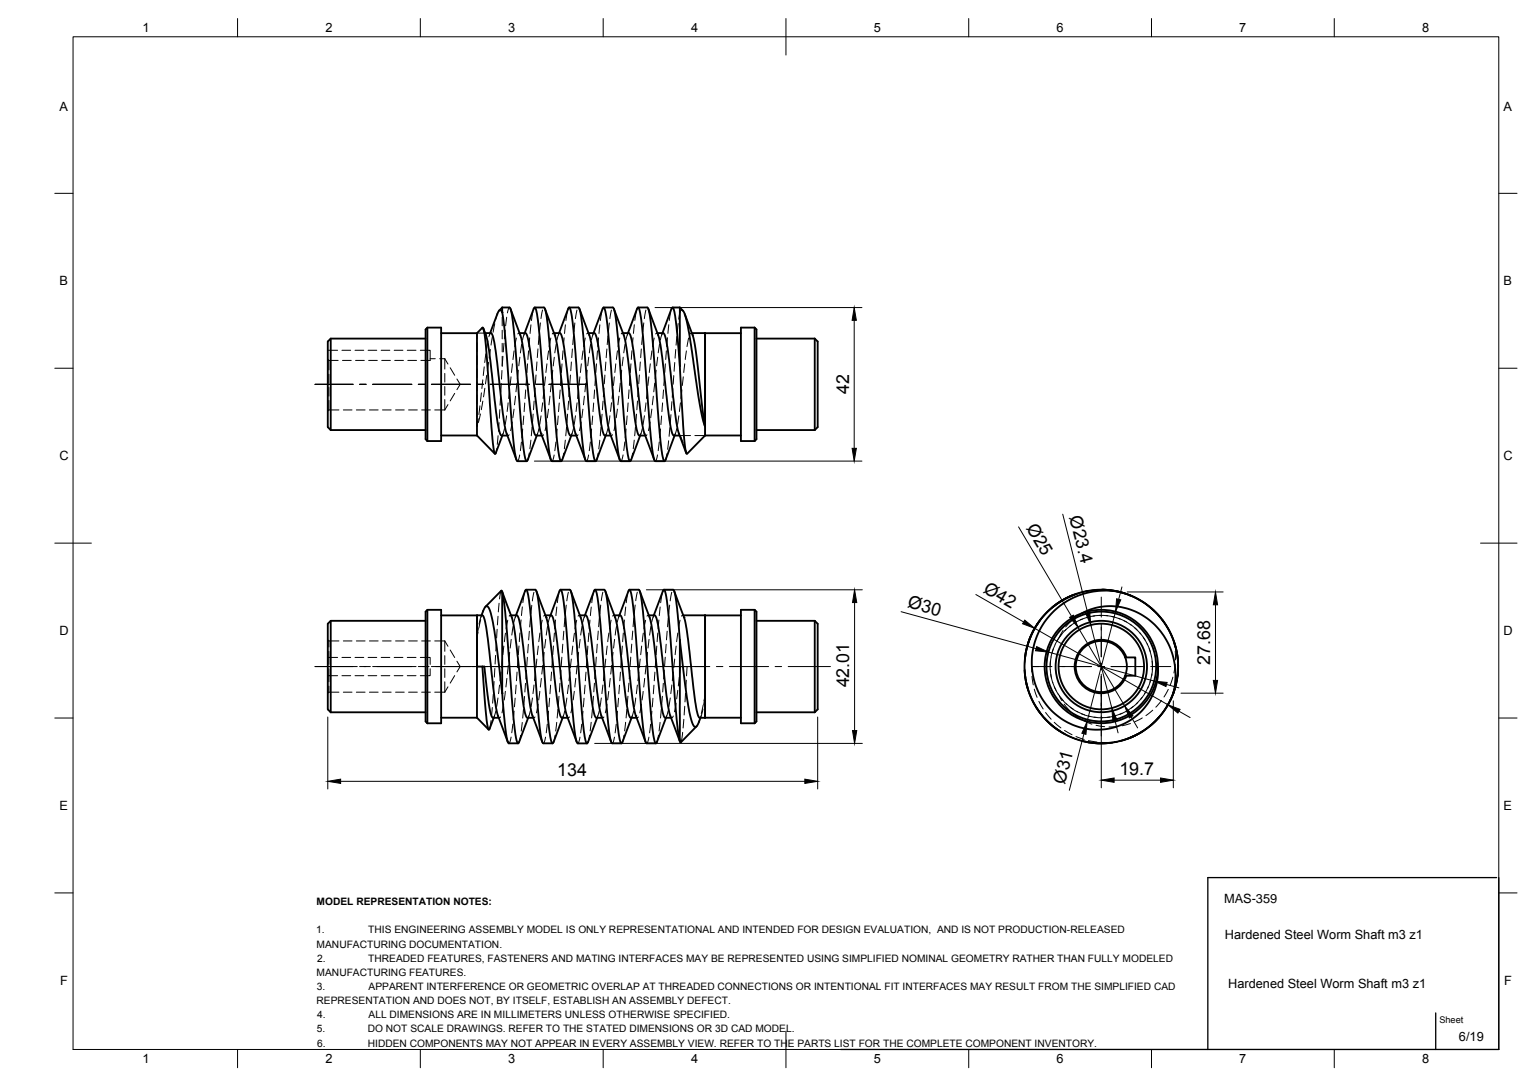
ISO-10303-21;
HEADER;
/* Generated by software containing ST-Developer
 * from STEP Tools, Inc. (www.steptools.com) 
 */

FILE_DESCRIPTION(
/* description */ (''),
/* implementation_level */ '2;1');

FILE_NAME(
/* name */ 'Hardened Steel Worm Shaft m3 z1.step',
/* time_stamp */ '2026-10-15T14:25:16-07:00',
/* author */ (''),
/* organization */ (''),
/* preprocessor_version */ 'ST-DEVELOPER v20.2',
/* originating_system */ 'Autodesk Translation Framework v15.15.0.0',
/* authorisation */ '');

FILE_SCHEMA (('AUTOMOTIVE_DESIGN { 1 0 10303 214 3 1 1 }'));
ENDSEC;

DATA;
#10=MECHANICAL_DESIGN_GEOMETRIC_PRESENTATION_REPRESENTATION('',(#326),#86429);
#161=B_SPLINE_SURFACE_WITH_KNOTS('',3,3,((#24275,#24276,#24277,#24278,#24279,
#24280,#24281,#24282,#24283,#24284,#24285,#24286,#24287,#24288,#24289,#24290,
#24291,#24292,#24293,#24294,#24295,#24296,#24297,#24298,#24299,#24300,#24301,
#24302,#24303,#24304,#24305,#24306,#24307,#24308,#24309,#24310,#24311,#24312,
#24313,#24314,#24315,#24316,#24317,#24318,#24319,#24320,#24321,#24322,#24323,
#24324,#24325,#24326,#24327,#24328,#24329,#24330,#24331,#24332,#24333,#24334,
#24335,#24336,#24337,#24338,#24339,#24340,#24341,#24342,#24343,#24344,#24345,
#24346,#24347,#24348,#24349,#24350,#24351,#24352,#24353,#24354,#24355,#24356,
#24357,#24358,#24359,#24360,#24361,#24362,#24363,#24364,#24365,#24366,#24367,
#24368,#24369,#24370,#24371,#24372,#24373,#24374,#24375,#24376,#24377,#24378,
#24379,#24380,#24381,#24382,#24383,#24384,#24385,#24386,#24387,#24388,#24389,
#24390,#24391,#24392,#24393,#24394,#24395,#24396,#24397,#24398,#24399,#24400,
#24401,#24402,#24403,#24404,#24405,#24406,#24407,#24408,#24409,#24410,#24411,
#24412,#24413,#24414,#24415,#24416,#24417),(#24418,#24419,#24420,#24421,
#24422,#24423,#24424,#24425,#24426,#24427,#24428,#24429,#24430,#24431,#24432,
#24433,#24434,#24435,#24436,#24437,#24438,#24439,#24440,#24441,#24442,#24443,
#24444,#24445,#24446,#24447,#24448,#24449,#24450,#24451,#24452,#24453,#24454,
#24455,#24456,#24457,#24458,#24459,#24460,#24461,#24462,#24463,#24464,#24465,
#24466,#24467,#24468,#24469,#24470,#24471,#24472,#24473,#24474,#24475,#24476,
#24477,#24478,#24479,#24480,#24481,#24482,#24483,#24484,#24485,#24486,#24487,
#24488,#24489,#24490,#24491,#24492,#24493,#24494,#24495,#24496,#24497,#24498,
#24499,#24500,#24501,#24502,#24503,#24504,#24505,#24506,#24507,#24508,#24509,
#24510,#24511,#24512,#24513,#24514,#24515,#24516,#24517,#24518,#24519,#24520,
#24521,#24522,#24523,#24524,#24525,#24526,#24527,#24528,#24529,#24530,#24531,
#24532,#24533,#24534,#24535,#24536,#24537,#24538,#24539,#24540,#24541,#24542,
#24543,#24544,#24545,#24546,#24547,#24548,#24549,#24550,#24551,#24552,#24553,
#24554,#24555,#24556,#24557,#24558,#24559,#24560),(#24561,#24562,#24563,
#24564,#24565,#24566,#24567,#24568,#24569,#24570,#24571,#24572,#24573,#24574,
#24575,#24576,#24577,#24578,#24579,#24580,#24581,#24582,#24583,#24584,#24585,
#24586,#24587,#24588,#24589,#24590,#24591,#24592,#24593,#24594,#24595,#24596,
#24597,#24598,#24599,#24600,#24601,#24602,#24603,#24604,#24605,#24606,#24607,
#24608,#24609,#24610,#24611,#24612,#24613,#24614,#24615,#24616,#24617,#24618,
#24619,#24620,#24621,#24622,#24623,#24624,#24625,#24626,#24627,#24628,#24629,
#24630,#24631,#24632,#24633,#24634,#24635,#24636,#24637,#24638,#24639,#24640,
#24641,#24642,#24643,#24644,#24645,#24646,#24647,#24648,#24649,#24650,#24651,
#24652,#24653,#24654,#24655,#24656,#24657,#24658,#24659,#24660,#24661,#24662,
#24663,#24664,#24665,#24666,#24667,#24668,#24669,#24670,#24671,#24672,#24673,
#24674,#24675,#24676,#24677,#24678,#24679,#24680,#24681,#24682,#24683,#24684,
#24685,#24686,#24687,#24688,#24689,#24690,#24691,#24692,#24693,#24694,#24695,
#24696,#24697,#24698,#24699,#24700,#24701,#24702,#24703),(#24704,#24705,
#24706,#24707,#24708,#24709,#24710,#24711,#24712,#24713,#24714,#24715,#24716,
#24717,#24718,#24719,#24720,#24721,#24722,#24723,#24724,#24725,#24726,#24727,
#24728,#24729,#24730,#24731,#24732,#24733,#24734,#24735,#24736,#24737,#24738,
#24739,#24740,#24741,#24742,#24743,#24744,#24745,#24746,#24747,#24748,#24749,
#24750,#24751,#24752,#24753,#24754,#24755,#24756,#24757,#24758,#24759,#24760,
#24761,#24762,#24763,#24764,#24765,#24766,#24767,#24768,#24769,#24770,#24771,
#24772,#24773,#24774,#24775,#24776,#24777,#24778,#24779,#24780,#24781,#24782,
#24783,#24784,#24785,#24786,#24787,#24788,#24789,#24790,#24791,#24792,#24793,
#24794,#24795,#24796,#24797,#24798,#24799,#24800,#24801,#24802,#24803,#24804,
#24805,#24806,#24807,#24808,#24809,#24810,#24811,#24812,#24813,#24814,#24815,
#24816,#24817,#24818,#24819,#24820,#24821,#24822,#24823,#24824,#24825,#24826,
#24827,#24828,#24829,#24830,#24831,#24832,#24833,#24834,#24835,#24836,#24837,
#24838,#24839,#24840,#24841,#24842,#24843,#24844,#24845,#24846)),
 .UNSPECIFIED.,.F.,.F.,.F.,(4,4),(4,1,1,1,2,1,1,1,1,1,1,1,1,1,2,1,1,1,1,
2,1,1,1,1,2,1,1,2,2,1,1,1,1,1,1,2,1,2,1,1,1,2,1,1,1,2,1,1,1,2,1,1,1,2,1,
1,1,2,1,1,1,2,1,1,1,2,1,1,1,1,1,2,1,1,1,1,1,1,2,2,1,1,2,1,1,1,1,2,1,1,1,
1,2,1,1,1,1,1,1,1,1,1,2,1,1,1,1,1,2,2,1,1,1,1,1,1,4),(-7.42398645807014E-6,
0.252864181465206),(0.121233664526765,0.122596153817018,0.123197115362701,
0.123397435877929,0.124999999999751,0.135817307706478,0.146634615413206,
0.15745192309109,0.168269230768974,0.177884615384371,0.187499999999768,
0.199519230740103,0.206730769230503,0.210336538446854,0.211538461538235,
0.213942307720923,0.218749999970821,0.228365384586246,0.237980769201671,
0.249999999999808,0.25841346152381,0.266826923047812,0.281250000028623,
0.289663461552636,0.298076923076649,0.312499999999747,0.31971153849016,
0.326923076922846,0.33653846153821,0.338942307720942,0.340144230783416,
0.343749999970879,0.353365384586257,0.358173076951719,0.362980769201619,
0.365384615384414,0.370192307692066,0.37499999999969,0.389423076922836,
0.397836538475728,0.406250000028619,0.413461538461298,0.420673076893946,
0.425480769259405,0.427884615384363,0.432692307692057,0.433894230783419,
0.43509615387478,0.437499999999749,0.442307692307468,0.455528846139201,
0.468749999970934,0.483173076951685,0.49999999999975,0.516826923047797,
0.531250000028611,0.544471153860329,0.557692307692047,0.562499999999739,
0.563701923062234,0.564903846124729,0.567307692307427,0.569711538490167,
0.574519230740095,0.579326923105555,0.586538461538202,0.593749999970866,
0.602163461523769,0.610576923076672,0.624999999999777,0.629807692307439,
0.634615384615125,0.637019230797861,0.641826923047781,0.646634615413246,
0.656250000028622,0.659855769216081,0.661057692278563,0.663461538461287,
0.673076923076666,0.680288461509321,0.687499999999755,0.701923076922838,
0.710336538446858,0.718749999970878,0.733173076951697,0.741586538475723,
0.749999999999749,0.762019230797881,0.771634615413259,0.781250000028636,
0.786057692278561,0.788461538461294,0.78966346155265,0.793269230768981,
0.800480769259399,0.812499999999748,0.822115384615134,0.83173076923052,
0.842548076908385,0.853365384586251,0.864182692292999,0.874999999999748,
0.876602564121565,0.876802884636793,0.877403846182474,0.879807692307444,
0.882211538432407,0.884615384615134,0.894230769230516,0.895432692321882,
0.906250000028634,0.915865384644013,0.926682692321841,0.937499999999668,
0.949519230731432,0.955682525542283),.UNSPECIFIED.);
#162=B_SPLINE_SURFACE_WITH_KNOTS('',3,3,((#25484,#25485,#25486,#25487,#25488,
#25489,#25490,#25491,#25492,#25493,#25494,#25495,#25496,#25497,#25498,#25499,
#25500,#25501,#25502,#25503,#25504,#25505,#25506,#25507,#25508,#25509,#25510,
#25511,#25512,#25513,#25514,#25515,#25516,#25517,#25518,#25519,#25520,#25521,
#25522,#25523,#25524,#25525,#25526,#25527,#25528,#25529,#25530,#25531,#25532,
#25533,#25534,#25535,#25536,#25537,#25538,#25539,#25540,#25541,#25542,#25543,
#25544,#25545,#25546,#25547,#25548,#25549,#25550,#25551,#25552,#25553,#25554,
#25555,#25556,#25557,#25558,#25559,#25560,#25561,#25562,#25563,#25564,#25565,
#25566,#25567,#25568,#25569,#25570,#25571,#25572,#25573,#25574,#25575,#25576,
#25577,#25578,#25579,#25580,#25581,#25582,#25583,#25584,#25585,#25586,#25587,
#25588,#25589,#25590,#25591,#25592,#25593,#25594,#25595,#25596,#25597,#25598,
#25599,#25600,#25601,#25602,#25603,#25604,#25605,#25606,#25607,#25608,#25609,
#25610,#25611,#25612,#25613,#25614,#25615,#25616,#25617,#25618,#25619,#25620,
#25621,#25622,#25623,#25624,#25625,#25626,#25627,#25628,#25629,#25630,#25631,
#25632,#25633,#25634,#25635,#25636,#25637,#25638,#25639,#25640,#25641,#25642,
#25643,#25644,#25645,#25646),(#25647,#25648,#25649,#25650,#25651,#25652,
#25653,#25654,#25655,#25656,#25657,#25658,#25659,#25660,#25661,#25662,#25663,
#25664,#25665,#25666,#25667,#25668,#25669,#25670,#25671,#25672,#25673,#25674,
#25675,#25676,#25677,#25678,#25679,#25680,#25681,#25682,#25683,#25684,#25685,
#25686,#25687,#25688,#25689,#25690,#25691,#25692,#25693,#25694,#25695,#25696,
#25697,#25698,#25699,#25700,#25701,#25702,#25703,#25704,#25705,#25706,#25707,
#25708,#25709,#25710,#25711,#25712,#25713,#25714,#25715,#25716,#25717,#25718,
#25719,#25720,#25721,#25722,#25723,#25724,#25725,#25726,#25727,#25728,#25729,
#25730,#25731,#25732,#25733,#25734,#25735,#25736,#25737,#25738,#25739,#25740,
#25741,#25742,#25743,#25744,#25745,#25746,#25747,#25748,#25749,#25750,#25751,
#25752,#25753,#25754,#25755,#25756,#25757,#25758,#25759,#25760,#25761,#25762,
#25763,#25764,#25765,#25766,#25767,#25768,#25769,#25770,#25771,#25772,#25773,
#25774,#25775,#25776,#25777,#25778,#25779,#25780,#25781,#25782,#25783,#25784,
#25785,#25786,#25787,#25788,#25789,#25790,#25791,#25792,#25793,#25794,#25795,
#25796,#25797,#25798,#25799,#25800,#25801,#25802,#25803,#25804,#25805,#25806,
#25807,#25808,#25809),(#25810,#25811,#25812,#25813,#25814,#25815,#25816,
#25817,#25818,#25819,#25820,#25821,#25822,#25823,#25824,#25825,#25826,#25827,
#25828,#25829,#25830,#25831,#25832,#25833,#25834,#25835,#25836,#25837,#25838,
#25839,#25840,#25841,#25842,#25843,#25844,#25845,#25846,#25847,#25848,#25849,
#25850,#25851,#25852,#25853,#25854,#25855,#25856,#25857,#25858,#25859,#25860,
#25861,#25862,#25863,#25864,#25865,#25866,#25867,#25868,#25869,#25870,#25871,
#25872,#25873,#25874,#25875,#25876,#25877,#25878,#25879,#25880,#25881,#25882,
#25883,#25884,#25885,#25886,#25887,#25888,#25889,#25890,#25891,#25892,#25893,
#25894,#25895,#25896,#25897,#25898,#25899,#25900,#25901,#25902,#25903,#25904,
#25905,#25906,#25907,#25908,#25909,#25910,#25911,#25912,#25913,#25914,#25915,
#25916,#25917,#25918,#25919,#25920,#25921,#25922,#25923,#25924,#25925,#25926,
#25927,#25928,#25929,#25930,#25931,#25932,#25933,#25934,#25935,#25936,#25937,
#25938,#25939,#25940,#25941,#25942,#25943,#25944,#25945,#25946,#25947,#25948,
#25949,#25950,#25951,#25952,#25953,#25954,#25955,#25956,#25957,#25958,#25959,
#25960,#25961,#25962,#25963,#25964,#25965,#25966,#25967,#25968,#25969,#25970,
#25971,#25972),(#25973,#25974,#25975,#25976,#25977,#25978,#25979,#25980,
#25981,#25982,#25983,#25984,#25985,#25986,#25987,#25988,#25989,#25990,#25991,
#25992,#25993,#25994,#25995,#25996,#25997,#25998,#25999,#26000,#26001,#26002,
#26003,#26004,#26005,#26006,#26007,#26008,#26009,#26010,#26011,#26012,#26013,
#26014,#26015,#26016,#26017,#26018,#26019,#26020,#26021,#26022,#26023,#26024,
#26025,#26026,#26027,#26028,#26029,#26030,#26031,#26032,#26033,#26034,#26035,
#26036,#26037,#26038,#26039,#26040,#26041,#26042,#26043,#26044,#26045,#26046,
#26047,#26048,#26049,#26050,#26051,#26052,#26053,#26054,#26055,#26056,#26057,
#26058,#26059,#26060,#26061,#26062,#26063,#26064,#26065,#26066,#26067,#26068,
#26069,#26070,#26071,#26072,#26073,#26074,#26075,#26076,#26077,#26078,#26079,
#26080,#26081,#26082,#26083,#26084,#26085,#26086,#26087,#26088,#26089,#26090,
#26091,#26092,#26093,#26094,#26095,#26096,#26097,#26098,#26099,#26100,#26101,
#26102,#26103,#26104,#26105,#26106,#26107,#26108,#26109,#26110,#26111,#26112,
#26113,#26114,#26115,#26116,#26117,#26118,#26119,#26120,#26121,#26122,#26123,
#26124,#26125,#26126,#26127,#26128,#26129,#26130,#26131,#26132,#26133,#26134,
#26135)),.UNSPECIFIED.,.F.,.F.,.F.,(4,4),(4,1,1,1,1,1,1,1,1,1,1,2,2,1,1,
1,1,1,2,1,1,1,1,1,1,1,1,1,2,1,1,1,1,2,1,1,1,1,2,1,1,2,2,1,1,1,1,1,1,2,1,
2,1,1,1,2,1,1,1,2,1,1,1,2,1,1,1,2,1,1,1,2,1,1,1,2,1,1,1,2,1,1,1,2,1,2,1,
1,1,1,1,1,2,2,1,1,2,1,1,1,1,2,1,1,1,1,2,1,1,1,1,1,1,1,1,1,2,1,1,1,1,1,2,
2,1,1,1,1,1,1,1,1,1,4),(0.0100803267684296,0.756239113823487),(-3.07676242782602E-5,
0.00841344965183915,0.0168268993036783,0.0312500013956658,0.0408653845261411,
0.0504807692681131,0.062499999999838,0.0733173076776515,0.0841346153554649,
0.0937499999708451,0.104567307677615,0.105769230768995,0.115384615384363,
0.117788461567088,0.120192307692056,0.122596153817018,0.123197115362701,
0.123397435877929,0.124999999999751,0.135817307706478,0.146634615413206,
0.15745192309109,0.168269230768974,0.177884615384371,0.187499999999768,
0.199519230740103,0.206730769230503,0.210336538446854,0.211538461538235,
0.213942307720923,0.218749999970821,0.228365384586246,0.237980769201671,
0.249999999999808,0.25841346152381,0.266826923047812,0.281250000028623,
0.289663461552636,0.298076923076649,0.312499999999747,0.31971153849016,
0.326923076922846,0.33653846153821,0.338942307720942,0.340144230783416,
0.343749999970879,0.353365384586257,0.358173076951719,0.362980769201619,
0.365384615384414,0.370192307692066,0.37499999999969,0.389423076922836,
0.397836538475728,0.406250000028619,0.413461538461298,0.420673076893946,
0.425480769259405,0.427884615384363,0.432692307692057,0.433894230783419,
0.43509615387478,0.437499999999749,0.442307692307468,0.455528846139201,
0.468749999970934,0.483173076951685,0.49999999999975,0.516826923047797,
0.531250000028611,0.544471153860329,0.557692307692047,0.562499999999739,
0.563701923062234,0.564903846124729,0.567307692307427,0.569711538490167,
0.574519230740095,0.579326923105555,0.586538461538202,0.593749999970866,
0.602163461523769,0.610576923076672,0.624999999999777,0.629807692307439,
0.634615384615125,0.637019230797861,0.641826923047781,0.646634615413246,
0.656250000028622,0.659855769216081,0.661057692278563,0.663461538461287,
0.673076923076666,0.680288461509321,0.687499999999755,0.701923076922838,
0.710336538446858,0.718749999970878,0.733173076951697,0.741586538475723,
0.749999999999749,0.762019230797881,0.771634615413259,0.781250000028636,
0.786057692278561,0.788461538461294,0.78966346155265,0.793269230768981,
0.800480769259399,0.812499999999748,0.822115384615134,0.83173076923052,
0.842548076908385,0.853365384586251,0.864182692292999,0.874999999999748,
0.876602564121565,0.876802884636793,0.877403846182474,0.879807692307444,
0.882211538432407,0.884615384615134,0.894230769230516,0.895432692321882,
0.906250000028634,0.915865384644013,0.926682692321841,0.937499999999668,
0.949519230731432,0.95913461547336,0.968749998603834,0.983173100695849,
0.985231553658313),.UNSPECIFIED.);
#163=B_SPLINE_SURFACE_WITH_KNOTS('',3,3,((#26138,#26139,#26140,#26141,#26142,
#26143,#26144,#26145,#26146,#26147,#26148,#26149,#26150,#26151,#26152,#26153,
#26154,#26155,#26156,#26157,#26158,#26159,#26160,#26161,#26162,#26163,#26164,
#26165,#26166,#26167,#26168,#26169,#26170,#26171,#26172,#26173,#26174,#26175,
#26176,#26177,#26178,#26179,#26180,#26181,#26182,#26183,#26184,#26185,#26186,
#26187,#26188,#26189,#26190,#26191,#26192,#26193,#26194,#26195,#26196,#26197,
#26198,#26199,#26200,#26201,#26202,#26203,#26204,#26205,#26206,#26207,#26208,
#26209,#26210,#26211,#26212,#26213,#26214,#26215,#26216,#26217,#26218,#26219,
#26220,#26221,#26222,#26223,#26224,#26225,#26226,#26227,#26228,#26229,#26230,
#26231,#26232,#26233,#26234,#26235,#26236,#26237,#26238,#26239,#26240,#26241,
#26242,#26243,#26244,#26245,#26246,#26247,#26248,#26249,#26250,#26251,#26252,
#26253,#26254,#26255,#26256,#26257,#26258,#26259,#26260,#26261,#26262,#26263,
#26264,#26265,#26266,#26267,#26268,#26269,#26270,#26271,#26272,#26273,#26274,
#26275,#26276,#26277,#26278,#26279,#26280,#26281,#26282,#26283,#26284,#26285,
#26286,#26287,#26288,#26289,#26290,#26291,#26292,#26293),(#26294,#26295,
#26296,#26297,#26298,#26299,#26300,#26301,#26302,#26303,#26304,#26305,#26306,
#26307,#26308,#26309,#26310,#26311,#26312,#26313,#26314,#26315,#26316,#26317,
#26318,#26319,#26320,#26321,#26322,#26323,#26324,#26325,#26326,#26327,#26328,
#26329,#26330,#26331,#26332,#26333,#26334,#26335,#26336,#26337,#26338,#26339,
#26340,#26341,#26342,#26343,#26344,#26345,#26346,#26347,#26348,#26349,#26350,
#26351,#26352,#26353,#26354,#26355,#26356,#26357,#26358,#26359,#26360,#26361,
#26362,#26363,#26364,#26365,#26366,#26367,#26368,#26369,#26370,#26371,#26372,
#26373,#26374,#26375,#26376,#26377,#26378,#26379,#26380,#26381,#26382,#26383,
#26384,#26385,#26386,#26387,#26388,#26389,#26390,#26391,#26392,#26393,#26394,
#26395,#26396,#26397,#26398,#26399,#26400,#26401,#26402,#26403,#26404,#26405,
#26406,#26407,#26408,#26409,#26410,#26411,#26412,#26413,#26414,#26415,#26416,
#26417,#26418,#26419,#26420,#26421,#26422,#26423,#26424,#26425,#26426,#26427,
#26428,#26429,#26430,#26431,#26432,#26433,#26434,#26435,#26436,#26437,#26438,
#26439,#26440,#26441,#26442,#26443,#26444,#26445,#26446,#26447,#26448,#26449),
(#26450,#26451,#26452,#26453,#26454,#26455,#26456,#26457,#26458,#26459,
#26460,#26461,#26462,#26463,#26464,#26465,#26466,#26467,#26468,#26469,#26470,
#26471,#26472,#26473,#26474,#26475,#26476,#26477,#26478,#26479,#26480,#26481,
#26482,#26483,#26484,#26485,#26486,#26487,#26488,#26489,#26490,#26491,#26492,
#26493,#26494,#26495,#26496,#26497,#26498,#26499,#26500,#26501,#26502,#26503,
#26504,#26505,#26506,#26507,#26508,#26509,#26510,#26511,#26512,#26513,#26514,
#26515,#26516,#26517,#26518,#26519,#26520,#26521,#26522,#26523,#26524,#26525,
#26526,#26527,#26528,#26529,#26530,#26531,#26532,#26533,#26534,#26535,#26536,
#26537,#26538,#26539,#26540,#26541,#26542,#26543,#26544,#26545,#26546,#26547,
#26548,#26549,#26550,#26551,#26552,#26553,#26554,#26555,#26556,#26557,#26558,
#26559,#26560,#26561,#26562,#26563,#26564,#26565,#26566,#26567,#26568,#26569,
#26570,#26571,#26572,#26573,#26574,#26575,#26576,#26577,#26578,#26579,#26580,
#26581,#26582,#26583,#26584,#26585,#26586,#26587,#26588,#26589,#26590,#26591,
#26592,#26593,#26594,#26595,#26596,#26597,#26598,#26599,#26600,#26601,#26602,
#26603,#26604,#26605),(#26606,#26607,#26608,#26609,#26610,#26611,#26612,
#26613,#26614,#26615,#26616,#26617,#26618,#26619,#26620,#26621,#26622,#26623,
#26624,#26625,#26626,#26627,#26628,#26629,#26630,#26631,#26632,#26633,#26634,
#26635,#26636,#26637,#26638,#26639,#26640,#26641,#26642,#26643,#26644,#26645,
#26646,#26647,#26648,#26649,#26650,#26651,#26652,#26653,#26654,#26655,#26656,
#26657,#26658,#26659,#26660,#26661,#26662,#26663,#26664,#26665,#26666,#26667,
#26668,#26669,#26670,#26671,#26672,#26673,#26674,#26675,#26676,#26677,#26678,
#26679,#26680,#26681,#26682,#26683,#26684,#26685,#26686,#26687,#26688,#26689,
#26690,#26691,#26692,#26693,#26694,#26695,#26696,#26697,#26698,#26699,#26700,
#26701,#26702,#26703,#26704,#26705,#26706,#26707,#26708,#26709,#26710,#26711,
#26712,#26713,#26714,#26715,#26716,#26717,#26718,#26719,#26720,#26721,#26722,
#26723,#26724,#26725,#26726,#26727,#26728,#26729,#26730,#26731,#26732,#26733,
#26734,#26735,#26736,#26737,#26738,#26739,#26740,#26741,#26742,#26743,#26744,
#26745,#26746,#26747,#26748,#26749,#26750,#26751,#26752,#26753,#26754,#26755,
#26756,#26757,#26758,#26759,#26760,#26761)),.UNSPECIFIED.,.F.,.F.,.F.,(4,
4),(4,1,1,2,2,1,1,1,1,1,2,1,1,1,1,1,1,1,1,1,2,1,1,1,1,2,1,1,1,1,2,1,1,2,
2,1,1,1,1,1,1,2,1,2,1,1,1,2,1,1,1,2,1,1,1,2,1,1,1,2,1,1,1,2,1,1,1,2,1,1,
1,2,1,1,1,2,1,2,1,1,1,1,1,1,2,2,1,1,2,1,1,1,1,2,1,1,1,1,2,1,1,1,1,1,1,1,
1,1,2,1,1,1,1,1,2,2,1,1,1,1,1,1,1,1,1,1,4),(-0.000390275080997305,0.745485974455544),
(0.0915777109701609,0.0937499999708451,0.104567307677615,0.105769230768995,
0.115384615384363,0.117788461567088,0.120192307692056,0.122596153817018,
0.123197115362701,0.123397435877929,0.124999999999751,0.135817307706478,
0.146634615413206,0.15745192309109,0.168269230768974,0.177884615384371,
0.187499999999768,0.199519230740103,0.206730769230503,0.210336538446854,
0.211538461538235,0.213942307720923,0.218749999970821,0.228365384586246,
0.237980769201671,0.249999999999808,0.25841346152381,0.266826923047812,
0.281250000028623,0.289663461552636,0.298076923076649,0.312499999999747,
0.31971153849016,0.326923076922846,0.33653846153821,0.338942307720942,0.340144230783416,
0.343749999970879,0.353365384586257,0.358173076951719,0.362980769201619,
0.365384615384414,0.370192307692066,0.37499999999969,0.389423076922836,
0.397836538475728,0.406250000028619,0.413461538461298,0.420673076893946,
0.425480769259405,0.427884615384363,0.432692307692057,0.433894230783419,
0.43509615387478,0.437499999999749,0.442307692307468,0.455528846139201,
0.468749999970934,0.483173076951685,0.49999999999975,0.516826923047797,
0.531250000028611,0.544471153860329,0.557692307692047,0.562499999999739,
0.563701923062234,0.564903846124729,0.567307692307427,0.569711538490167,
0.574519230740095,0.579326923105555,0.586538461538202,0.593749999970866,
0.602163461523769,0.610576923076672,0.624999999999777,0.629807692307439,
0.634615384615125,0.637019230797861,0.641826923047781,0.646634615413246,
0.656250000028622,0.659855769216081,0.661057692278563,0.663461538461287,
0.673076923076666,0.680288461509321,0.687499999999755,0.701923076922838,
0.710336538446858,0.718749999970878,0.733173076951697,0.741586538475723,
0.749999999999749,0.762019230797881,0.771634615413259,0.781250000028636,
0.786057692278561,0.788461538461294,0.78966346155265,0.793269230768981,
0.800480769259399,0.812499999999748,0.822115384615134,0.83173076923052,
0.842548076908385,0.853365384586251,0.864182692292999,0.874999999999748,
0.876602564121565,0.876802884636793,0.877403846182474,0.879807692307444,
0.882211538432407,0.884615384615134,0.894230769230516,0.895432692321882,
0.906250000028634,0.915865384644013,0.926682692321841,0.937499999999668,
0.949519230731432,0.95913461547336,0.968749998603834,0.983173100695849,
0.991586550347924,1.0000372584433),.UNSPECIFIED.);
#260=(
BOUNDED_CURVE()
B_SPLINE_CURVE(2,(#23943,#23944,#23945),.UNSPECIFIED.,.F.,.F.)
B_SPLINE_CURVE_WITH_KNOTS((3,3),(0.,0.0438796975155138),.UNSPECIFIED.)
CURVE()
GEOMETRIC_REPRESENTATION_ITEM()
RATIONAL_B_SPLINE_CURVE((1.,1.00025082231383,1.))
REPRESENTATION_ITEM('')
);
#261=(
BOUNDED_CURVE()
B_SPLINE_CURVE(2,(#23957,#23958,#23959),.UNSPECIFIED.,.F.,.F.)
B_SPLINE_CURVE_WITH_KNOTS((3,3),(0.,0.0438796975155138),.UNSPECIFIED.)
CURVE()
GEOMETRIC_REPRESENTATION_ITEM()
RATIONAL_B_SPLINE_CURVE((1.,1.00025082231383,1.))
REPRESENTATION_ITEM('')
);
#290=SHAPE_REPRESENTATION_RELATIONSHIP('SRR','None',#86505,#308);
#308=ADVANCED_BREP_SHAPE_REPRESENTATION('',(#344),#86414);
#326=STYLED_ITEM('',(#86604),#344);
#344=MANIFOLD_SOLID_BREP('Body1',#15616);
#395=B_SPLINE_CURVE_WITH_KNOTS('',3,(#23127,#23128,#23129,#23130,#23131,
#23132,#23133,#23134,#23135,#23136,#23137,#23138,#23139,#23140,#23141,#23142,
#23143,#23144,#23145,#23146,#23147,#23148,#23149,#23150,#23151,#23152,#23153,
#23154,#23155,#23156,#23157,#23158,#23159,#23160,#23161,#23162,#23163,#23164,
#23165,#23166,#23167,#23168,#23169,#23170,#23171,#23172,#23173,#23174,#23175,
#23176,#23177,#23178,#23179,#23180,#23181,#23182,#23183,#23184,#23185,#23186,
#23187,#23188),.UNSPECIFIED.,.F.,.F.,(4,2,2,2,2,2,2,2,2,2,2,2,2,2,2,2,2,
2,2,2,2,2,2,2,2,2,2,2,2,2,4),(48.3095209509747,48.3438126061204,48.481226208238,
48.7564115875427,48.8943879405152,49.1670882523347,49.4057479328213,49.5435390452519,
49.8157502041263,50.086596913725,50.3608603822337,50.907937332897,51.1838264118632,
51.4592719418958,52.0080440963282,52.2810596578922,52.4186420978999,52.6942356980283,
53.2414178320407,53.3792880152578,53.6599840542201,53.9346199725026,54.4787854744381,
54.7497288191555,55.0208858330499,55.5745224561154,55.8470714557858,56.2861992300559,
56.5144008207168,56.6298096390493,56.7452388041896),.UNSPECIFIED.);
#396=B_SPLINE_CURVE_WITH_KNOTS('',3,(#23193,#23194,#23195,#23196,#23197,
#23198),.UNSPECIFIED.,.F.,.F.,(4,2,4),(0.000824378371301782,0.307333000414166,
0.426549198415677),.UNSPECIFIED.);
#397=B_SPLINE_CURVE_WITH_KNOTS('',3,(#23203,#23204,#23205,#23206,#23207,
#23208,#23209,#23210,#23211,#23212,#23213,#23214,#23215,#23216,#23217,#23218,
#23219,#23220,#23221,#23222,#23223,#23224,#23225,#23226,#23227,#23228,#23229,
#23230,#23231,#23232,#23233,#23234,#23235,#23236,#23237,#23238,#23239,#23240,
#23241,#23242,#23243,#23244,#23245,#23246,#23247,#23248,#23249,#23250,#23251,
#23252,#23253,#23254,#23255,#23256,#23257,#23258),.UNSPECIFIED.,.F.,.F.,
(4,2,2,2,2,2,2,2,2,2,2,2,2,2,2,2,2,2,2,2,2,2,2,2,2,2,2,4),(39.4473895294157,
39.6410372250372,40.0957750453416,40.3654377525067,40.6583563356197,40.9344854155672,
41.4872248887745,41.755996746073,42.1841163903161,42.557814705178,42.8338667979832,
43.1095103949903,43.6634534770776,43.9349491227225,44.2067442703658,44.4807550283175,
44.7532491351571,45.0271301508351,45.3010640927362,45.5768720367176,46.1309839511959,
46.5611880266105,46.8321636906455,47.0750044321246,47.350424720883,47.6223526303686,
47.8963704741162,48.3095209509747),.UNSPECIFIED.);
#398=B_SPLINE_CURVE_WITH_KNOTS('',3,(#23259,#23260,#23261,#23262,#23263,
#23264,#23265,#23266,#23267,#23268,#23269,#23270,#23271,#23272,#23273,#23274,
#23275,#23276,#23277,#23278,#23279,#23280,#23281,#23282,#23283,#23284,#23285,
#23286,#23287,#23288,#23289,#23290,#23291,#23292,#23293,#23294,#23295,#23296,
#23297,#23298,#23299,#23300,#23301,#23302,#23303,#23304,#23305,#23306,#23307,
#23308,#23309,#23310,#23311,#23312,#23313,#23314,#23315,#23316,#23317,#23318),
 .UNSPECIFIED.,.F.,.F.,(4,2,2,2,2,2,2,2,2,2,2,2,2,2,2,2,2,2,2,2,2,2,2,2,
2,2,2,2,2,4),(0.426549198415677,0.614191706618979,1.01002600072371,1.48582906984535,
1.73759812188067,2.01062010057207,2.56389527135009,2.83633022706529,3.1081672480776,
3.64857217350429,3.78620389269443,4.34106360761934,4.61723684328365,4.89201771080173,
5.16743328258393,5.44296844699991,5.58036719526417,6.12790418811079,6.4032185522103,
6.67910469076678,6.95504464088112,7.2275421020416,7.36514240490451,7.83280211438953,
7.97052980987632,8.45937656117122,8.59709328117351,9.08556481291611,9.22324652695596,
9.28838277977079),.UNSPECIFIED.);
#399=B_SPLINE_CURVE_WITH_KNOTS('',3,(#23323,#23324,#23325,#23326,#23327,
#23328,#23329,#23330,#23331,#23332,#23333,#23334,#23335,#23336,#23337,#23338,
#23339,#23340,#23341,#23342,#23343,#23344,#23345,#23346,#23347,#23348,#23349,
#23350,#23351,#23352,#23353,#23354,#23355,#23356,#23357,#23358,#23359,#23360,
#23361,#23362,#23363,#23364,#23365,#23366,#23367,#23368,#23369,#23370,#23371,
#23372,#23373,#23374,#23375,#23376,#23377,#23378,#23379,#23380,#23381,#23382,
#23383,#23384,#23385,#23386,#23387,#23388,#23389,#23390),.UNSPECIFIED.,
 .F.,.F.,(4,2,2,2,2,2,2,2,2,2,2,2,2,2,2,2,2,2,2,2,2,2,2,2,2,2,2,2,2,2,2,
2,2,4),(30.5866212966661,30.6469362186711,31.0261209213079,31.2978607379824,
31.7939621385182,32.0654867500116,32.2460223109104,32.7976124523937,32.9354482217323,
33.0733378306324,33.2112285916035,33.3491078585792,33.6242471271187,33.7619713364408,
34.0361140014156,34.1738247544983,34.4478069684183,34.7232900527495,35.2770415980905,
35.5501868477252,35.7887137967358,36.3430806261292,36.6190105141371,36.8949931496492,
37.1708524034991,37.4465777704499,37.5844613566104,37.8577982383939,37.9952584033865,
38.2699550429054,38.5435740429261,38.8173456070261,39.0912255075645,39.4473895294157),
 .UNSPECIFIED.);
#400=B_SPLINE_CURVE_WITH_KNOTS('',3,(#23391,#23392,#23393,#23394,#23395,
#23396,#23397,#23398,#23399,#23400,#23401,#23402,#23403,#23404,#23405,#23406,
#23407,#23408,#23409,#23410,#23411,#23412,#23413,#23414,#23415,#23416,#23417,
#23418,#23419,#23420,#23421,#23422,#23423,#23424,#23425,#23426,#23427,#23428,
#23429,#23430,#23431,#23432,#23433,#23434,#23435,#23436,#23437,#23438,#23439,
#23440,#23441,#23442,#23443,#23444,#23445,#23446,#23447,#23448),
 .UNSPECIFIED.,.F.,.F.,(4,2,2,2,2,2,2,2,2,2,2,2,2,2,2,2,2,2,2,2,2,2,2,2,
2,2,2,2,4),(9.28838277977079,9.69957849302504,9.97380096579599,10.2462470500306,
10.3838569093476,10.8129824883417,10.9507459110335,11.5141586961433,11.7884642076982,
12.0640566356795,12.3397813255604,12.614174112575,12.8892030655763,13.1614192721906,
13.2991037273397,13.5746845444855,14.1259124003885,14.2636924951075,14.8151556448298,
15.0915097232107,15.3718497780372,15.9274951705087,16.0651506906214,16.6104057666243,
16.8859839527044,17.2493313174359,17.5200638539738,18.0608178392373,18.1514671267416),
 .UNSPECIFIED.);
#401=B_SPLINE_CURVE_WITH_KNOTS('',3,(#23453,#23454,#23455,#23456,#23457,
#23458,#23459,#23460,#23461,#23462,#23463,#23464,#23465,#23466,#23467,#23468,
#23469,#23470,#23471,#23472,#23473,#23474,#23475,#23476,#23477,#23478,#23479,
#23480,#23481,#23482,#23483,#23484,#23485,#23486,#23487,#23488,#23489,#23490,
#23491,#23492,#23493,#23494,#23495,#23496,#23497,#23498,#23499,#23500,#23501,
#23502,#23503,#23504,#23505,#23506,#23507,#23508,#23509,#23510,#23511,#23512,
#23513,#23514,#23515,#23516,#23517,#23518,#23519,#23520),.UNSPECIFIED.,
 .F.,.F.,(4,2,2,2,2,2,2,2,2,2,2,2,2,2,2,2,2,2,2,2,2,2,2,2,2,2,2,2,2,2,2,
2,2,4),(21.7281508769804,21.859292462676,22.1347421134665,22.4138620953436,
22.6872284752932,22.9632671779943,23.1008811145477,23.3736294193785,23.6486966165464,
23.7864302925312,24.0619441755822,24.199625648023,24.3374800874459,24.6134095278544,
24.7512635221148,25.0272402972866,25.1650661303055,25.3026888072312,25.5774460693942,
25.8508320352646,26.2838985525551,26.5551310298002,26.9440332751233,27.2126940433332,
27.7565528573337,28.0278344389847,28.3724041446136,28.708047633284,28.9733600116614,
29.2041603109075,29.5653567879662,29.8366592676533,30.3783623722413,30.5866212966661),
 .UNSPECIFIED.);
#402=B_SPLINE_CURVE_WITH_KNOTS('',3,(#23521,#23522,#23523,#23524,#23525,
#23526,#23527,#23528,#23529,#23530,#23531,#23532,#23533,#23534,#23535,#23536,
#23537,#23538,#23539,#23540,#23541,#23542,#23543,#23544,#23545,#23546,#23547,
#23548,#23549,#23550,#23551,#23552,#23553,#23554,#23555,#23556,#23557,#23558,
#23559,#23560,#23561,#23562,#23563,#23564,#23565,#23566,#23567,#23568,#23569,
#23570,#23571,#23572,#23573,#23574,#23575,#23576,#23577,#23578,#23579,#23580,
#23581,#23582,#23583,#23584,#23585,#23586,#23587,#23588),.UNSPECIFIED.,
 .F.,.F.,(4,2,2,2,2,2,2,2,2,2,2,2,2,2,2,2,2,2,2,2,2,2,2,2,2,2,2,2,2,2,2,
2,2,4),(18.1514671267416,18.3359725867351,18.8879297461098,19.1636965767125,
19.3013917945595,19.8552808656922,20.1308659781475,20.4060615379671,20.6818851569234,
20.9577875123256,21.2337405314606,21.5081460257525,21.6197260439793,22.172500653785,
22.3102732515512,22.8627418433339,23.138149633494,23.4111694467411,23.5489071631255,
23.8222381557675,23.9599828842976,24.2346751933028,24.3725314687067,24.5103462088827,
24.6482043889914,24.785933581394,24.9238088698136,25.4775940615791,25.6160547495808,
25.8909936109743,26.1614289065469,26.7114543958306,26.9823357781454,27.0126062280082),
 .UNSPECIFIED.);
#403=B_SPLINE_CURVE_WITH_KNOTS('',3,(#23593,#23594,#23595,#23596,#23597,
#23598,#23599,#23600,#23601,#23602,#23603,#23604,#23605,#23606,#23607,#23608,
#23609,#23610,#23611,#23612,#23613,#23614,#23615,#23616,#23617,#23618,#23619,
#23620,#23621,#23622,#23623,#23624,#23625,#23626,#23627,#23628,#23629,#23630,
#23631,#23632,#23633,#23634,#23635,#23636,#23637,#23638,#23639,#23640,#23641,
#23642,#23643,#23644,#23645,#23646,#23647,#23648,#23649,#23650,#23651,#23652,
#23653,#23654),.UNSPECIFIED.,.F.,.F.,(4,2,2,2,2,2,2,2,2,2,2,2,2,2,2,2,2,
2,2,2,2,2,2,2,2,2,2,2,2,2,4),(12.8673372881869,13.1045912480947,13.3784206922435,
13.6508493140918,13.9224251719806,14.4747733220309,14.7502018033826,15.0261882292162,
15.2867204870524,15.7143806877064,16.1397500990148,16.4122973490567,16.9672169387799,
17.2033227276788,17.4726908823725,18.037876335385,18.3124420816258,18.8598305789335,
18.9974121921246,19.2729763606579,19.5488031042003,19.8228552663192,20.097625942618,
20.3704230665631,20.6463274234226,20.9217341125824,21.0596243445807,21.3351615072599,
21.4724476291603,21.721963084712,21.7281508769804),.UNSPECIFIED.);
#404=B_SPLINE_CURVE_WITH_KNOTS('',3,(#23655,#23656,#23657,#23658,#23659,
#23660,#23661,#23662,#23663,#23664,#23665,#23666,#23667,#23668,#23669,#23670,
#23671,#23672,#23673,#23674,#23675,#23676,#23677,#23678,#23679,#23680,#23681,
#23682,#23683,#23684,#23685,#23686,#23687,#23688,#23689,#23690,#23691,#23692,
#23693,#23694,#23695,#23696,#23697,#23698,#23699,#23700,#23701,#23702,#23703,
#23704,#23705,#23706,#23707,#23708,#23709,#23710,#23711,#23712,#23713,#23714,
#23715,#23716,#23717,#23718),.UNSPECIFIED.,.F.,.F.,(4,2,2,2,2,2,2,2,2,2,
2,2,2,2,2,2,2,2,2,2,2,2,2,2,2,2,2,2,2,2,2,4),(27.0126062280082,27.3028829986553,
27.8351272737622,28.0388596861804,28.4737664649467,28.7408417219884,28.9998149350992,
29.2355762469122,29.4192788621494,29.6954983810387,30.0670604013279,30.6244762789582,
30.9498794660956,31.4902800694265,31.763897147745,32.0371486886421,32.3104751893334,
32.4482035971803,32.72417276819,32.8620543008062,32.9999247087657,33.2758973613899,
33.5518702088626,33.8273566843513,33.9652030027378,34.240225672795,34.5140108716027,
34.6516577003026,34.9275167223425,35.2011094137945,35.6443705723813,35.8725192426511),
 .UNSPECIFIED.);
#405=B_SPLINE_CURVE_WITH_KNOTS('',3,(#23723,#23724,#23725,#23726,#23727,
#23728,#23729,#23730,#23731,#23732,#23733,#23734,#23735,#23736,#23737,#23738,
#23739,#23740,#23741,#23742,#23743,#23744,#23745,#23746,#23747,#23748,#23749,
#23750,#23751,#23752,#23753,#23754,#23755,#23756,#23757,#23758,#23759,#23760,
#23761,#23762,#23763,#23764,#23765,#23766,#23767,#23768,#23769,#23770,#23771,
#23772,#23773,#23774,#23775,#23776,#23777,#23778,#23779,#23780,#23781,#23782,
#23783,#23784),.UNSPECIFIED.,.F.,.F.,(4,2,2,2,2,2,2,2,2,2,2,2,2,2,2,2,2,
2,2,2,2,2,2,2,2,2,2,2,2,2,4),(4.00579666373733,4.22413930375615,4.36190267992724,
4.91034098288094,5.18600966471709,5.32349953457887,5.59632872461622,6.14663667970456,
6.42222459948757,6.69804980819117,7.2474319093848,7.38486184776289,7.83922119968481,
7.97688389264115,8.52926536854384,8.80482269152215,9.08530248842244,9.22296907620534,
9.71155236699991,9.98575858600692,10.2588795271958,10.5345327905916,10.7699146367297,
11.0408326712101,11.5939442609587,11.8696146241601,12.1455514363969,12.2834279870469,
12.5577920931176,12.8314615618714,12.8673372881869),.UNSPECIFIED.);
#406=B_SPLINE_CURVE_WITH_KNOTS('',3,(#23785,#23786,#23787,#23788,#23789,
#23790,#23791,#23792,#23793,#23794,#23795,#23796,#23797,#23798,#23799,#23800,
#23801,#23802,#23803,#23804,#23805,#23806,#23807,#23808,#23809,#23810,#23811,
#23812,#23813,#23814,#23815,#23816,#23817,#23818,#23819,#23820,#23821,#23822,
#23823,#23824,#23825,#23826,#23827,#23828,#23829,#23830,#23831,#23832,#23833,
#23834,#23835,#23836,#23837,#23838,#23839,#23840,#23841,#23842),
 .UNSPECIFIED.,.F.,.F.,(4,2,2,2,2,2,2,2,2,2,2,2,2,2,2,2,2,2,2,2,2,2,2,2,
2,2,2,2,4),(35.8725192426511,35.9151842174268,36.09983440795,36.3742808891897,
36.5122035519266,36.6501205150463,36.9260423900668,37.2019237953068,37.4769431036303,
37.7524677979035,38.3063620750602,38.4441238522539,38.7198610588383,39.2714120779741,
39.5465499155902,40.1111820373952,40.3816152785012,40.6708302493013,40.946855041263,
41.4986518734995,41.7690904826401,42.2242805568422,42.5186658754165,42.7949816988295,
43.3460251568471,43.6210829792625,43.8937594718918,44.3327289395869,44.7369456500769),
 .UNSPECIFIED.);
#407=B_SPLINE_CURVE_WITH_KNOTS('',3,(#23845,#23846,#23847,#23848,#23849,
#23850,#23851,#23852,#23853,#23854,#23855,#23856,#23857,#23858,#23859,#23860,
#23861,#23862,#23863,#23864,#23865,#23866,#23867,#23868,#23869,#23870,#23871,
#23872,#23873,#23874,#23875,#23876,#23877,#23878,#23879,#23880,#23881,#23882,
#23883,#23884,#23885,#23886,#23887,#23888,#23889,#23890,#23891,#23892,#23893,
#23894,#23895,#23896,#23897,#23898,#23899,#23900,#23901,#23902),
 .UNSPECIFIED.,.F.,.F.,(4,2,2,2,2,2,2,2,2,2,2,2,2,2,2,2,2,2,2,2,2,2,2,2,
2,2,2,2,4),(44.7369456500769,44.8867742748783,45.0245971947796,45.2985652981441,
45.5743906456427,46.1283912454116,46.5570552926755,46.8287680120469,47.0682425531597,
47.3440177136997,47.6178066999295,47.8923482402771,48.1645791411325,48.3023652432245,
48.574971680631,48.8464001383451,49.1209239039586,49.3951619578507,49.5330723902179,
49.8059417425042,50.0766678420903,50.3516170304178,50.9023268700414,51.1781921554573,
51.453978195975,51.8867436693424,52.1031849749825,52.2112916210837,52.3187924201233),
 .UNSPECIFIED.);
#408=B_SPLINE_CURVE_WITH_KNOTS('',3,(#23907,#23908,#23909,#23910,#23911,
#23912,#23913,#23914,#23915,#23916,#23917,#23918,#23919,#23920,#23921,#23922,
#23923,#23924,#23925,#23926,#23927,#23928,#23929,#23930,#23931,#23932),
 .UNSPECIFIED.,.F.,.F.,(4,2,2,2,2,2,2,2,2,2,2,2,4),(0.000824364847128334,
0.279789559980365,0.559133666621795,1.03110720678431,1.40797268178914,1.75551901563212,
2.02774233750806,2.58176080895605,2.85228694703896,3.12295036047126,3.66872486797347,
3.9434825123866,4.00579666373733),.UNSPECIFIED.);
#409=B_SPLINE_CURVE_WITH_KNOTS('',3,(#23985,#23986,#23987,#23988,#23989,
#23990,#23991,#23992,#23993,#23994,#23995,#23996,#23997,#23998,#23999,#24000,
#24001,#24002,#24003,#24004,#24005,#24006,#24007,#24008,#24009,#24010),
 .UNSPECIFIED.,.F.,.F.,(4,2,2,2,2,2,2,2,2,2,2,2,4),(9.99999998997544E-7,
0.277509193145354,0.559562005090733,1.13595993001213,1.45422004501248,2.10759695469075,
2.43887984940046,3.11114962502898,3.45649386180175,3.80276810060717,4.51975710851416,
5.24677359279633,5.41878430004213),.UNSPECIFIED.);
#410=B_SPLINE_CURVE_WITH_KNOTS('',3,(#24013,#24014,#24015,#24016,#24017,
#24018,#24019,#24020,#24021,#24022,#24023,#24024,#24025,#24026,#24027,#24028,
#24029,#24030,#24031,#24032,#24033,#24034,#24035,#24036,#24037,#24038,#24039,
#24040,#24041,#24042,#24043,#24044,#24045,#24046,#24047,#24048,#24049,#24050,
#24051,#24052,#24053,#24054,#24055,#24056,#24057,#24058,#24059,#24060,#24061,
#24062,#24063,#24064,#24065,#24066,#24067,#24068,#24069,#24070,#24071,#24072,
#24073,#24074,#24075,#24076,#24077,#24078,#24079,#24080,#24081,#24082,#24083,
#24084,#24085,#24086,#24087,#24088,#24089,#24090,#24091,#24092,#24093,#24094,
#24095,#24096,#24097,#24098,#24099,#24100,#24101,#24102,#24103,#24104,#24105,
#24106,#24107,#24108,#24109,#24110,#24111,#24112,#24113,#24114,#24115,#24116,
#24117,#24118),.UNSPECIFIED.,.F.,.F.,(4,3,3,3,3,3,3,3,3,3,3,3,3,3,3,3,3,
3,3,3,3,3,3,3,3,3,3,3,3,3,3,3,3,3,3,4),(-5.14602986437962,-4.9124571768068,
-4.71371046276571,-4.54086707520652,-4.32250456683061,-4.10713809464024,
-3.95554536139003,-3.82420547225028,-3.61585834214411,-3.41052234213242,
-3.20824947806771,-3.00469258194512,-2.97873918630968,-2.77502713067335,
-2.57493296082448,-2.49620314801143,-2.29768232080681,-2.17849548023144,
-2.06364564461087,-2.04936478423458,-2.00662821804358,-1.83737350397171,
-1.81938711170177,-1.67044184854484,-1.50530496693403,-1.31867939695959,
-1.17777177287489,-0.994244625335878,-0.867823569922663,-0.790542128771154,
-0.608686868523352,-0.571323537610721,-0.394394587266291,-0.220420986284586,
-0.120990393829573,-0.00018052822953134),.UNSPECIFIED.);
#411=B_SPLINE_CURVE_WITH_KNOTS('',3,(#24120,#24121,#24122,#24123,#24124,
#24125,#24126,#24127,#24128,#24129,#24130,#24131,#24132,#24133,#24134,#24135,
#24136,#24137,#24138,#24139,#24140,#24141,#24142,#24143,#24144,#24145,#24146,
#24147,#24148,#24149,#24150,#24151,#24152,#24153,#24154,#24155,#24156,#24157,
#24158,#24159,#24160,#24161,#24162,#24163,#24164,#24165,#24166,#24167,#24168,
#24169,#24170,#24171,#24172,#24173,#24174,#24175,#24176,#24177,#24178,#24179,
#24180,#24181,#24182,#24183),.UNSPECIFIED.,.F.,.F.,(4,3,3,3,3,3,3,3,3,3,
3,3,3,3,3,3,3,3,3,3,3,4),(-3.54929782707136,-3.43298875244871,-3.38136321121889,
-3.36415083557511,-3.22642372778473,-3.00517870020166,-2.77298587052083,
-2.54081959100311,-2.46105968243433,-2.29735828955663,-2.06510807290758,
-1.83230960956431,-1.64070659226555,-1.40756763421874,-1.36661117934383,
-1.133848457372,-0.90127112443142,-0.820353364661033,-0.587108315483886,
-0.435770693368578,-0.202446776608828,-1.64264001317083E-5),
 .UNSPECIFIED.);
#412=B_SPLINE_CURVE_WITH_KNOTS('',3,(#24184,#24185,#24186,#24187,#24188,
#24189,#24190,#24191,#24192,#24193,#24194,#24195,#24196,#24197,#24198,#24199,
#24200,#24201,#24202,#24203),.UNSPECIFIED.,.F.,.F.,(4,2,2,2,2,2,2,2,2,4),
(5.41878430004213,5.612905067052,5.98508461978949,6.35542810705476,6.73497483683354,
7.11388681821555,7.89769154966654,8.16903003314377,8.58256664643331,8.99852632498306),
 .UNSPECIFIED.);
#413=B_SPLINE_CURVE_WITH_KNOTS('',3,(#24207,#24208,#24209,#24210,#24211,
#24212,#24213,#24214,#24215,#24216,#24217,#24218,#24219,#24220,#24221,#24222,
#24223,#24224,#24225,#24226,#24227,#24228,#24229,#24230,#24231,#24232),
 .UNSPECIFIED.,.F.,.F.,(4,2,2,2,2,2,2,2,2,2,2,2,4),(2.24906504782965E-5,
0.571634272981765,1.12074908741776,1.48125473010532,1.85616076048785,2.58661322797785,
2.93330821431849,3.27144832173647,3.91512369926488,4.53192872349113,4.84787148574749,
5.00150736838493,5.15431373386902),.UNSPECIFIED.);
#414=B_SPLINE_CURVE_WITH_KNOTS('',3,(#24234,#24235,#24236,#24237,#24238,
#24239,#24240,#24241,#24242,#24243,#24244,#24245,#24246,#24247),
 .UNSPECIFIED.,.F.,.F.,(4,2,2,2,2,2,4),(0.,0.474678646281976,0.942829047193473,
1.51670727039287,1.90291538542257,2.09764827213206,2.29412506652137),
 .UNSPECIFIED.);
#415=B_SPLINE_CURVE_WITH_KNOTS('',3,(#24249,#24250,#24251,#24252,#24253,
#24254,#24255,#24256,#24257,#24258,#24259,#24260,#24261,#24262,#24263,#24264,
#24265,#24266),.UNSPECIFIED.,.F.,.F.,(4,2,2,2,2,2,2,2,4),(0.,0.350415922095155,
0.706087820863965,1.42957591857985,1.81390106464849,2.61485609197721,3.11237077026773,
3.36521279740499,3.6186598959626),.UNSPECIFIED.);
#416=B_SPLINE_CURVE_WITH_KNOTS('',3,(#24847,#24848,#24849,#24850,#24851,
#24852,#24853,#24854,#24855,#24856,#24857,#24858,#24859,#24860,#24861,#24862,
#24863,#24864,#24865,#24866,#24867,#24868,#24869,#24870,#24871,#24872,#24873,
#24874,#24875,#24876,#24877,#24878,#24879,#24880,#24881,#24882,#24883,#24884,
#24885,#24886,#24887,#24888,#24889,#24890,#24891,#24892,#24893,#24894,#24895,
#24896,#24897,#24898,#24899,#24900,#24901,#24902,#24903,#24904,#24905,#24906,
#24907,#24908,#24909,#24910,#24911,#24912,#24913,#24914,#24915,#24916,#24917,
#24918,#24919,#24920,#24921,#24922,#24923,#24924,#24925,#24926,#24927,#24928,
#24929,#24930,#24931,#24932,#24933,#24934,#24935,#24936,#24937,#24938,#24939,
#24940,#24941,#24942,#24943,#24944,#24945,#24946,#24947,#24948,#24949,#24950,
#24951,#24952,#24953,#24954,#24955,#24956,#24957,#24958,#24959,#24960,#24961,
#24962,#24963,#24964,#24965,#24966,#24967,#24968,#24969,#24970,#24971,#24972,
#24973,#24974,#24975,#24976,#24977,#24978,#24979,#24980,#24981),
 .UNSPECIFIED.,.F.,.F.,(4,1,1,1,1,1,1,2,1,1,1,1,2,1,1,1,1,2,1,1,2,2,1,1,
1,1,1,1,2,1,2,1,1,1,2,1,1,1,2,1,1,1,2,1,1,1,2,1,1,1,2,1,1,1,2,1,1,1,2,1,
1,1,1,1,2,1,1,1,1,1,1,2,2,1,1,2,1,1,1,1,2,1,1,1,1,2,1,1,1,1,1,1,1,1,1,2,
1,1,1,1,1,2,2,1,1,1,1,1,1,4),(0.162516398693048,0.168269230768974,0.177884615384371,
0.187499999999768,0.199519230740103,0.206730769230503,0.210336538446854,
0.211538461538235,0.213942307720923,0.218749999970821,0.228365384586246,
0.237980769201671,0.249999999999808,0.25841346152381,0.266826923047812,
0.281250000028623,0.289663461552636,0.298076923076649,0.312499999999747,
0.31971153849016,0.326923076922846,0.33653846153821,0.338942307720942,0.340144230783416,
0.343749999970879,0.353365384586257,0.358173076951719,0.362980769201619,
0.365384615384414,0.370192307692066,0.37499999999969,0.389423076922836,
0.397836538475728,0.406250000028619,0.413461538461298,0.420673076893946,
0.425480769259405,0.427884615384363,0.432692307692057,0.433894230783419,
0.43509615387478,0.437499999999749,0.442307692307468,0.455528846139201,
0.468749999970934,0.483173076951685,0.49999999999975,0.516826923047797,
0.531250000028611,0.544471153860329,0.557692307692047,0.562499999999739,
0.563701923062234,0.564903846124729,0.567307692307427,0.569711538490167,
0.574519230740095,0.579326923105555,0.586538461538202,0.593749999970866,
0.602163461523769,0.610576923076672,0.624999999999777,0.629807692307439,
0.634615384615125,0.637019230797861,0.641826923047781,0.646634615413246,
0.656250000028622,0.659855769216081,0.661057692278563,0.663461538461287,
0.673076923076666,0.680288461509321,0.687499999999755,0.701923076922838,
0.710336538446858,0.718749999970878,0.733173076951697,0.741586538475723,
0.749999999999749,0.762019230797881,0.771634615413259,0.781250000028636,
0.786057692278561,0.788461538461294,0.78966346155265,0.793269230768981,
0.800480769259399,0.812499999999748,0.822115384615134,0.83173076923052,
0.842548076908385,0.853365384586251,0.864182692292999,0.874999999999748,
0.876602564121565,0.876802884636793,0.877403846182474,0.879807692307444,
0.882211538432407,0.884615384615134,0.894230769230516,0.895432692321882,
0.906250000028634,0.915865384644013,0.926682692321841,0.937499999999668,
0.949519230731432,0.955682525542283),.UNSPECIFIED.);
#417=B_SPLINE_CURVE_WITH_KNOTS('',3,(#24982,#24983,#24984,#24985,#24986,
#24987,#24988,#24989,#24990,#24991,#24992,#24993,#24994,#24995,#24996,#24997,
#24998,#24999,#25000,#25001,#25002,#25003,#25004,#25005,#25006,#25007,#25008,
#25009,#25010,#25011,#25012,#25013,#25014,#25015,#25016,#25017,#25018,#25019,
#25020,#25021,#25022,#25023,#25024,#25025,#25026,#25027,#25028,#25029,#25030,
#25031,#25032,#25033,#25034,#25035,#25036,#25037,#25038,#25039,#25040,#25041,
#25042,#25043,#25044,#25045,#25046,#25047,#25048,#25049,#25050,#25051,#25052,
#25053,#25054,#25055,#25056,#25057,#25058,#25059,#25060,#25061,#25062,#25063,
#25064,#25065,#25066,#25067,#25068,#25069,#25070,#25071,#25072,#25073,#25074,
#25075,#25076,#25077,#25078,#25079,#25080,#25081,#25082,#25083,#25084,#25085,
#25086,#25087,#25088,#25089,#25090,#25091,#25092,#25093,#25094,#25095,#25096,
#25097,#25098,#25099,#25100,#25101,#25102,#25103,#25104,#25105,#25106,#25107,
#25108,#25109,#25110,#25111,#25112,#25113,#25114,#25115,#25116,#25117,#25118,
#25119,#25120,#25121,#25122,#25123,#25124,#25125,#25126,#25127,#25128,#25129,
#25130,#25131,#25132,#25133,#25134,#25135,#25136,#25137,#25138,#25139,#25140,
#25141,#25142,#25143,#25144,#25145,#25146,#25147,#25148,#25149,#25150,#25151,
#25152,#25153,#25154,#25155,#25156,#25157,#25158,#25159,#25160,#25161,#25162,
#25163,#25164,#25165,#25166,#25167,#25168,#25169,#25170,#25171,#25172,#25173,
#25174,#25175,#25176,#25177,#25178,#25179,#25180,#25181,#25182,#25183,#25184,
#25185,#25186,#25187,#25188,#25189,#25190,#25191,#25192,#25193,#25194,#25195,
#25196,#25197,#25198,#25199,#25200,#25201,#25202,#25203,#25204,#25205,#25206,
#25207,#25208,#25209,#25210,#25211,#25212,#25213,#25214,#25215,#25216,#25217,
#25218,#25219,#25220,#25221,#25222,#25223,#25224,#25225,#25226,#25227,#25228,
#25229,#25230,#25231,#25232,#25233,#25234,#25235,#25236,#25237,#25238,#25239,
#25240,#25241,#25242,#25243,#25244,#25245,#25246,#25247,#25248,#25249,#25250,
#25251,#25252,#25253,#25254,#25255,#25256,#25257,#25258,#25259,#25260,#25261,
#25262,#25263,#25264,#25265,#25266,#25267,#25268,#25269,#25270,#25271,#25272,
#25273,#25274,#25275,#25276,#25277,#25278,#25279,#25280,#25281,#25282,#25283,
#25284,#25285,#25286,#25287,#25288,#25289,#25290,#25291,#25292,#25293,#25294,
#25295,#25296,#25297,#25298,#25299,#25300,#25301,#25302,#25303,#25304,#25305,
#25306,#25307,#25308,#25309,#25310,#25311,#25312,#25313,#25314,#25315,#25316,
#25317,#25318,#25319,#25320,#25321,#25322,#25323,#25324,#25325,#25326,#25327,
#25328,#25329,#25330,#25331,#25332,#25333,#25334,#25335,#25336,#25337,#25338,
#25339,#25340,#25341,#25342,#25343,#25344,#25345,#25346,#25347,#25348,#25349,
#25350,#25351,#25352,#25353,#25354,#25355,#25356,#25357,#25358,#25359,#25360,
#25361,#25362,#25363,#25364,#25365,#25366,#25367,#25368,#25369,#25370,#25371,
#25372,#25373,#25374,#25375,#25376,#25377,#25378,#25379,#25380,#25381,#25382,
#25383,#25384,#25385,#25386,#25387,#25388,#25389,#25390,#25391,#25392,#25393,
#25394,#25395,#25396,#25397,#25398,#25399,#25400,#25401,#25402,#25403,#25404,
#25405,#25406,#25407,#25408,#25409,#25410,#25411,#25412,#25413,#25414,#25415,
#25416,#25417,#25418,#25419,#25420,#25421,#25422,#25423,#25424,#25425,#25426,
#25427,#25428,#25429,#25430,#25431,#25432,#25433,#25434,#25435,#25436,#25437,
#25438,#25439,#25440,#25441,#25442,#25443,#25444,#25445,#25446,#25447,#25448,
#25449,#25450,#25451,#25452,#25453,#25454,#25455,#25456,#25457,#25458,#25459,
#25460,#25461,#25462,#25463,#25464,#25465,#25466,#25467,#25468,#25469,#25470,
#25471,#25472,#25473,#25474,#25475,#25476,#25477,#25478,#25479,#25480,#25481,
#25482,#25483),.UNSPECIFIED.,.F.,.F.,(4,3,3,3,3,3,3,3,3,3,3,3,3,3,3,3,3,
3,3,3,3,3,3,3,3,3,3,3,3,3,3,3,3,3,3,3,3,3,3,3,3,3,3,3,3,3,3,3,3,3,3,3,3,
3,3,3,3,3,3,3,3,3,3,3,3,3,3,3,3,3,3,3,3,3,3,3,3,3,3,3,3,3,3,3,3,3,3,3,3,
3,3,3,3,3,3,3,3,3,3,3,3,3,3,3,3,3,3,3,3,3,3,3,3,3,3,3,3,3,3,3,3,3,3,3,3,
3,3,3,3,3,3,3,3,3,3,3,3,3,3,3,3,3,3,3,3,3,3,3,3,3,3,3,3,3,3,3,3,3,3,3,3,
3,3,3,3,3,3,4),(0.121241235866819,0.122596333952119,0.123197306239647,0.123397630454117,
0.125000220490707,0.135817558564196,0.146634821242987,0.157452054343042,
0.16826930039866,0.177884615384371,0.177884648357071,0.187499999999768,
0.199519216306826,0.199519230740103,0.206730748861056,0.206730769230503,
0.210336516868093,0.210336538446854,0.211538439269354,0.211538461538235,
0.213942284455432,0.213942307720923,0.21874997552603,0.218749999970821,
0.22836536738934,0.228365384586246,0.237980769201671,0.250000006012719,
0.25841346152381,0.266826923047812,0.281250000028623,0.289663461552636,
0.298076913590586,0.312499999999747,0.31971153849016,0.326923094679332,
0.336538484588579,0.338942331282927,0.340144254583534,0.343750023825251,
0.35336540594336,0.358173095018189,0.362980782487174,0.365384626334338,
0.370192307692066,0.374999999391061,0.389423076922836,0.389423093033542,
0.397836575504186,0.406250058688912,0.413461607848517,0.420673152098523,
0.42548084303445,0.427884687070039,0.432692372895138,0.433894293991556,
0.435096214869763,0.43750005599482,0.442307736943911,0.455528868281594,
0.46875003733348,0.483173076951685,0.483173116205438,0.499999999838053,
0.51682688352103,0.516826923047797,0.531249962424686,0.531250000028611,
0.544471131109026,0.544471153860329,0.557692260171344,0.557692307692047,
0.562499939446951,0.562499999999739,0.563701859758352,0.563701923062234,
0.564903780248029,0.564903846124729,0.567307621420288,0.567307692307427,
0.569711463075703,0.569711538490167,0.574519148795765,0.574519230740095,
0.579326835836925,0.579326923105555,0.586538355389812,0.586538461538202,
0.593163510583565,0.593749999970866,0.593750080688083,0.600519790385705,
0.602163221950243,0.602163461523769,0.60896006288304,0.610576923076672,
0.61057724928789,0.617292450591262,0.623876825081465,0.624999612585041,
0.624999999999777,0.628545774026805,0.629807692307439,0.629808266711979,
0.63322388056985,0.634615284988846,0.634615384615125,0.637019175058555,
0.637019230797861,0.641826862941149,0.641826923047781,0.646634549684172,
0.646634615413246,0.656249954446322,0.656250000028622,0.659855725068628,
0.659855769216081,0.661057648907858,0.661057692278563,0.663461496685113,
0.663461538461287,0.673076896175284,0.673076923076666,0.680288447579257,
0.680288461509321,0.687499999999755,0.701923087601902,0.710336548577926,
0.718749999970878,0.733173076951697,0.741586538475723,0.749999993068343,
0.762019230797881,0.771634615413259,0.771634627337508,0.781250017474292,
0.786057708639458,0.788461554153435,0.789663476774355,0.79326924518666,
0.800480769259399,0.812499999999748,0.822115384615134,0.831730763372892,
0.842548076908385,0.853365384586251,0.864182692292999,0.874999982515718,
0.874999999999748,0.87660254418179,0.876602564121565,0.876802864442705,
0.876802884636793,0.877403825127061,0.877403846182474,0.879807666207773,
0.879807692307444,0.882211507161395,0.882211538432407,0.884615347276649,
0.884615384615134,0.894230680447608,0.894230769230516,0.895432604252924,
0.895432692321882,0.906249829255419,0.906250000028634,0.914406074621021),
 .UNSPECIFIED.);
#1227=CONICAL_SURFACE('',#16438,0.74,0.785398163397459);
#1228=CONICAL_SURFACE('',#16440,0.35,1.02974425867665);
#1229=CONICAL_SURFACE('',#16444,1.764,0.7936624380571);
#1230=CONICAL_SURFACE('',#16445,1.764,0.7936624380571);
#1231=CONICAL_SURFACE('',#16453,1.21,0.785398163397459);
#1232=CONICAL_SURFACE('',#16459,1.525,0.785398163397448);
#1233=CONICAL_SURFACE('',#16468,1.525,0.785398163397448);
#1234=CONICAL_SURFACE('',#16474,1.21,0.785398163397459);
#1432=CYLINDRICAL_SURFACE('',#16420,1.4);
#1433=CYLINDRICAL_SURFACE('',#16422,1.4);
#1434=CYLINDRICAL_SURFACE('',#16423,1.4);
#1435=CYLINDRICAL_SURFACE('',#16424,1.4);
#1436=CYLINDRICAL_SURFACE('',#16425,1.4);
#1437=CYLINDRICAL_SURFACE('',#16426,1.4);
#1438=CYLINDRICAL_SURFACE('',#16427,1.4);
#1439=CYLINDRICAL_SURFACE('',#16434,0.699999999999999);
#1440=CYLINDRICAL_SURFACE('',#16441,1.398);
#1441=CYLINDRICAL_SURFACE('',#16447,1.398);
#1442=CYLINDRICAL_SURFACE('',#16455,1.25);
#1443=CYLINDRICAL_SURFACE('',#16461,1.55);
#1444=CYLINDRICAL_SURFACE('',#16466,1.55);
#1445=CYLINDRICAL_SURFACE('',#16472,1.25);
#1699=FACE_BOUND('',#3727,.T.);
#1700=FACE_BOUND('',#3731,.T.);
#1701=FACE_BOUND('',#3733,.T.);
#1702=FACE_BOUND('',#3737,.T.);
#1703=FACE_BOUND('',#3741,.T.);
#1989=CIRCLE('',#16421,1.4);
#1990=CIRCLE('',#16428,1.4);
#1991=CIRCLE('',#16431,0.699999999999999);
#1992=CIRCLE('',#16435,0.699999999999999);
#1993=CIRCLE('',#16436,0.699999999999999);
#1994=CIRCLE('',#16437,0.699999999999999);
#1995=CIRCLE('',#16439,0.73);
#1996=CIRCLE('',#16442,1.398);
#1997=CIRCLE('',#16443,1.398);
#1998=CIRCLE('',#16446,1.398);
#1999=CIRCLE('',#16448,1.398);
#2000=CIRCLE('',#16452,1.17);
#2001=CIRCLE('',#16454,1.25);
#2002=CIRCLE('',#16456,1.25);
#2003=CIRCLE('',#16458,1.5);
#2004=CIRCLE('',#16460,1.55);
#2005=CIRCLE('',#16462,1.55);
#2006=CIRCLE('',#16465,1.55);
#2007=CIRCLE('',#16467,1.55);
#2008=CIRCLE('',#16469,1.5);
#2009=CIRCLE('',#16471,1.25);
#2010=CIRCLE('',#16473,1.25);
#2011=CIRCLE('',#16475,1.17);
#2731=FACE_OUTER_BOUND('',#3700,.T.);
#2732=FACE_OUTER_BOUND('',#3701,.T.);
#2733=FACE_OUTER_BOUND('',#3702,.T.);
#2734=FACE_OUTER_BOUND('',#3703,.T.);
#2735=FACE_OUTER_BOUND('',#3704,.T.);
#2736=FACE_OUTER_BOUND('',#3705,.T.);
#2737=FACE_OUTER_BOUND('',#3706,.T.);
#2738=FACE_OUTER_BOUND('',#3707,.T.);
#2739=FACE_OUTER_BOUND('',#3708,.T.);
#2740=FACE_OUTER_BOUND('',#3709,.T.);
#2741=FACE_OUTER_BOUND('',#3710,.T.);
#2742=FACE_OUTER_BOUND('',#3711,.T.);
#2743=FACE_OUTER_BOUND('',#3712,.T.);
#2744=FACE_OUTER_BOUND('',#3713,.T.);
#2745=FACE_OUTER_BOUND('',#3714,.T.);
#2746=FACE_OUTER_BOUND('',#3715,.T.);
#2747=FACE_OUTER_BOUND('',#3716,.T.);
#2748=FACE_OUTER_BOUND('',#3717,.T.);
#2749=FACE_OUTER_BOUND('',#3718,.T.);
#2750=FACE_OUTER_BOUND('',#3719,.T.);
#2751=FACE_OUTER_BOUND('',#3720,.T.);
#2752=FACE_OUTER_BOUND('',#3721,.T.);
#2753=FACE_OUTER_BOUND('',#3722,.T.);
#2754=FACE_OUTER_BOUND('',#3723,.T.);
#2755=FACE_OUTER_BOUND('',#3724,.T.);
#2756=FACE_OUTER_BOUND('',#3725,.T.);
#2757=FACE_OUTER_BOUND('',#3726,.T.);
#2758=FACE_OUTER_BOUND('',#3728,.T.);
#2759=FACE_OUTER_BOUND('',#3729,.T.);
#2760=FACE_OUTER_BOUND('',#3730,.T.);
#2761=FACE_OUTER_BOUND('',#3732,.T.);
#2762=FACE_OUTER_BOUND('',#3734,.T.);
#2763=FACE_OUTER_BOUND('',#3735,.T.);
#2764=FACE_OUTER_BOUND('',#3736,.T.);
#2765=FACE_OUTER_BOUND('',#3738,.T.);
#2766=FACE_OUTER_BOUND('',#3739,.T.);
#2767=FACE_OUTER_BOUND('',#3740,.T.);
#3700=EDGE_LOOP('',(#11531,#11532,#11533,#11534,#11535));
#3701=EDGE_LOOP('',(#11536,#11537,#11538,#11539));
#3702=EDGE_LOOP('',(#11540,#11541,#11542,#11543));
#3703=EDGE_LOOP('',(#11544,#11545,#11546,#11547));
#3704=EDGE_LOOP('',(#11548,#11549,#11550,#11551));
#3705=EDGE_LOOP('',(#11552,#11553,#11554,#11555));
#3706=EDGE_LOOP('',(#11556,#11557,#11558,#11559,#11560));
#3707=EDGE_LOOP('',(#11561,#11562,#11563,#11564,#11565));
#3708=EDGE_LOOP('',(#11566,#11567,#11568,#11569));
#3709=EDGE_LOOP('',(#11570,#11571,#11572,#11573,#11574));
#3710=EDGE_LOOP('',(#11575,#11576,#11577,#11578));
#3711=EDGE_LOOP('',(#11579,#11580,#11581,#11582,#11583,#11584,#11585,#11586));
#3712=EDGE_LOOP('',(#11587,#11588,#11589,#11590,#11591));
#3713=EDGE_LOOP('',(#11592,#11593,#11594));
#3714=EDGE_LOOP('',(#11595,#11596,#11597,#11598));
#3715=EDGE_LOOP('',(#11599,#11600,#11601,#11602,#11603,#11604,#11605,#11606,
#11607));
#3716=EDGE_LOOP('',(#11608,#11609,#11610,#11611,#11612,#11613,#11614,#11615));
#3717=EDGE_LOOP('',(#11616,#11617,#11618,#11619));
#3718=EDGE_LOOP('',(#11620,#11621,#11622,#11623));
#3719=EDGE_LOOP('',(#11624,#11625,#11626,#11627,#11628,#11629,#11630,#11631,
#11632,#11633,#11634,#11635));
#3720=EDGE_LOOP('',(#11636,#11637,#11638));
#3721=EDGE_LOOP('',(#11639,#11640,#11641,#11642,#11643,#11644,#11645,#11646,
#11647,#11648,#11649));
#3722=EDGE_LOOP('',(#11650,#11651,#11652));
#3723=EDGE_LOOP('',(#11653));
#3724=EDGE_LOOP('',(#11654,#11655,#11656,#11657));
#3725=EDGE_LOOP('',(#11658,#11659,#11660,#11661));
#3726=EDGE_LOOP('',(#11662));
#3727=EDGE_LOOP('',(#11663));
#3728=EDGE_LOOP('',(#11664,#11665,#11666,#11667));
#3729=EDGE_LOOP('',(#11668,#11669,#11670,#11671));
#3730=EDGE_LOOP('',(#11672));
#3731=EDGE_LOOP('',(#11673));
#3732=EDGE_LOOP('',(#11674));
#3733=EDGE_LOOP('',(#11675));
#3734=EDGE_LOOP('',(#11676,#11677,#11678,#11679));
#3735=EDGE_LOOP('',(#11680,#11681,#11682,#11683));
#3736=EDGE_LOOP('',(#11684));
#3737=EDGE_LOOP('',(#11685));
#3738=EDGE_LOOP('',(#11686,#11687,#11688,#11689));
#3739=EDGE_LOOP('',(#11690,#11691,#11692,#11693));
#3740=EDGE_LOOP('',(#11694));
#3741=EDGE_LOOP('',(#11695,#11696,#11697,#11698));
#4850=LINE('',#23125,#5710);
#4851=LINE('',#23192,#5711);
#4852=LINE('',#23202,#5712);
#4853=LINE('',#23322,#5713);
#4854=LINE('',#23452,#5714);
#4855=LINE('',#23592,#5715);
#4856=LINE('',#23722,#5716);
#4857=LINE('',#23906,#5717);
#4858=LINE('',#23936,#5718);
#4859=LINE('',#23938,#5719);
#4860=LINE('',#23940,#5720);
#4861=LINE('',#23942,#5721);
#4862=LINE('',#23950,#5722);
#4863=LINE('',#23951,#5723);
#4864=LINE('',#23955,#5724);
#4865=LINE('',#23960,#5725);
#4866=LINE('',#23961,#5726);
#4867=LINE('',#23963,#5727);
#4868=LINE('',#23968,#5728);
#4869=LINE('',#23975,#5729);
#4870=LINE('',#23980,#5730);
#4871=LINE('',#24011,#5731);
#4872=LINE('',#24204,#5732);
#4873=LINE('',#24267,#5733);
#4874=LINE('',#24269,#5734);
#4875=LINE('',#24273,#5735);
#4876=LINE('',#26136,#5736);
#4877=LINE('',#26762,#5737);
#4878=LINE('',#26770,#5738);
#4879=LINE('',#26774,#5739);
#4880=LINE('',#26781,#5740);
#4881=LINE('',#26785,#5741);
#4882=LINE('',#26793,#5742);
#4883=LINE('',#26796,#5743);
#4884=LINE('',#26804,#5744);
#4885=LINE('',#26807,#5745);
#5710=VECTOR('',#19037,1.4);
#5711=VECTOR('',#19040,1.);
#5712=VECTOR('',#19043,1.4);
#5713=VECTOR('',#19046,1.4);
#5714=VECTOR('',#19049,1.4);
#5715=VECTOR('',#19052,1.4);
#5716=VECTOR('',#19055,1.4);
#5717=VECTOR('',#19060,1.);
#5718=VECTOR('',#19063,1.);
#5719=VECTOR('',#19064,1.);
#5720=VECTOR('',#19065,1.);
#5721=VECTOR('',#19066,1.);
#5722=VECTOR('',#19071,1.);
#5723=VECTOR('',#19072,1.);
#5724=VECTOR('',#19075,1.);
#5725=VECTOR('',#19076,1.);
#5726=VECTOR('',#19077,1.);
#5727=VECTOR('',#19080,1.);
#5728=VECTOR('',#19085,0.699999999999999);
#5729=VECTOR('',#19096,0.35);
#5730=VECTOR('',#19101,1.398);
#5731=VECTOR('',#19106,1.);
#5732=VECTOR('',#19107,1.764);
#5733=VECTOR('',#19110,1.);
#5734=VECTOR('',#19111,1.764);
#5735=VECTOR('',#19116,1.398);
#5736=VECTOR('',#19119,1.);
#5737=VECTOR('',#19122,1.);
#5738=VECTOR('',#19133,1.21);
#5739=VECTOR('',#19138,1.25);
#5740=VECTOR('',#19147,1.525);
#5741=VECTOR('',#19152,1.55);
#5742=VECTOR('',#19163,1.55);
#5743=VECTOR('',#19166,1.525);
#5744=VECTOR('',#19177,1.25);
#5745=VECTOR('',#19180,1.21);
#6542=VERTEX_POINT('',#23123);
#6543=VERTEX_POINT('',#23124);
#6544=VERTEX_POINT('',#23126);
#6545=VERTEX_POINT('',#23189);
#6546=VERTEX_POINT('',#23191);
#6547=VERTEX_POINT('',#23200);
#6548=VERTEX_POINT('',#23201);
#6549=VERTEX_POINT('',#23320);
#6550=VERTEX_POINT('',#23321);
#6551=VERTEX_POINT('',#23450);
#6552=VERTEX_POINT('',#23451);
#6553=VERTEX_POINT('',#23590);
#6554=VERTEX_POINT('',#23591);
#6555=VERTEX_POINT('',#23720);
#6556=VERTEX_POINT('',#23721);
#6557=VERTEX_POINT('',#23844);
#6558=VERTEX_POINT('',#23903);
#6559=VERTEX_POINT('',#23905);
#6560=VERTEX_POINT('',#23934);
#6561=VERTEX_POINT('',#23935);
#6562=VERTEX_POINT('',#23937);
#6563=VERTEX_POINT('',#23939);
#6564=VERTEX_POINT('',#23941);
#6565=VERTEX_POINT('',#23947);
#6566=VERTEX_POINT('',#23949);
#6567=VERTEX_POINT('',#23953);
#6568=VERTEX_POINT('',#23954);
#6569=VERTEX_POINT('',#23956);
#6570=VERTEX_POINT('',#23965);
#6571=VERTEX_POINT('',#23967);
#6572=VERTEX_POINT('',#23974);
#6573=VERTEX_POINT('',#23977);
#6574=VERTEX_POINT('',#23979);
#6575=VERTEX_POINT('',#23983);
#6576=VERTEX_POINT('',#23984);
#6577=VERTEX_POINT('',#24012);
#6578=VERTEX_POINT('',#24119);
#6579=VERTEX_POINT('',#24206);
#6580=VERTEX_POINT('',#24233);
#6581=VERTEX_POINT('',#24248);
#6582=VERTEX_POINT('',#24268);
#6583=VERTEX_POINT('',#24272);
#6584=VERTEX_POINT('',#26765);
#6585=VERTEX_POINT('',#26768);
#6586=VERTEX_POINT('',#26772);
#6587=VERTEX_POINT('',#26776);
#6588=VERTEX_POINT('',#26779);
#6589=VERTEX_POINT('',#26783);
#6590=VERTEX_POINT('',#26788);
#6591=VERTEX_POINT('',#26791);
#6592=VERTEX_POINT('',#26795);
#6593=VERTEX_POINT('',#26799);
#6594=VERTEX_POINT('',#26802);
#6595=VERTEX_POINT('',#26806);
#8387=EDGE_CURVE('',#6542,#6543,#4850,.T.);
#8388=EDGE_CURVE('',#6542,#6544,#395,.T.);
#8389=EDGE_CURVE('',#6544,#6545,#1989,.T.);
#8390=EDGE_CURVE('',#6545,#6546,#4851,.T.);
#8391=EDGE_CURVE('',#6546,#6543,#396,.T.);
#8392=EDGE_CURVE('',#6547,#6548,#4852,.T.);
#8393=EDGE_CURVE('',#6547,#6542,#397,.T.);
#8394=EDGE_CURVE('',#6543,#6548,#398,.T.);
#8395=EDGE_CURVE('',#6549,#6550,#4853,.T.);
#8396=EDGE_CURVE('',#6549,#6547,#399,.T.);
#8397=EDGE_CURVE('',#6548,#6550,#400,.T.);
#8398=EDGE_CURVE('',#6551,#6552,#4854,.T.);
#8399=EDGE_CURVE('',#6551,#6549,#401,.T.);
#8400=EDGE_CURVE('',#6550,#6552,#402,.T.);
#8401=EDGE_CURVE('',#6553,#6554,#4855,.T.);
#8402=EDGE_CURVE('',#6553,#6551,#403,.T.);
#8403=EDGE_CURVE('',#6552,#6554,#404,.T.);
#8404=EDGE_CURVE('',#6555,#6556,#4856,.T.);
#8405=EDGE_CURVE('',#6555,#6553,#405,.T.);
#8406=EDGE_CURVE('',#6554,#6556,#406,.T.);
#8407=EDGE_CURVE('',#6556,#6557,#407,.T.);
#8408=EDGE_CURVE('',#6557,#6558,#1990,.T.);
#8409=EDGE_CURVE('',#6558,#6559,#4857,.T.);
#8410=EDGE_CURVE('',#6559,#6555,#408,.T.);
#8411=EDGE_CURVE('',#6560,#6561,#4858,.T.);
#8412=EDGE_CURVE('',#6560,#6562,#4859,.T.);
#8413=EDGE_CURVE('',#6563,#6562,#4860,.T.);
#8414=EDGE_CURVE('',#6564,#6563,#4861,.T.);
#8415=EDGE_CURVE('',#6561,#6564,#260,.T.);
#8416=EDGE_CURVE('',#6563,#6565,#1991,.T.);
#8417=EDGE_CURVE('',#6562,#6566,#4862,.T.);
#8418=EDGE_CURVE('',#6565,#6566,#4863,.T.);
#8419=EDGE_CURVE('',#6567,#6568,#4864,.T.);
#8420=EDGE_CURVE('',#6569,#6567,#261,.T.);
#8421=EDGE_CURVE('',#6565,#6569,#4865,.T.);
#8422=EDGE_CURVE('',#6566,#6568,#4866,.T.);
#8423=EDGE_CURVE('',#6568,#6560,#4867,.T.);
#8424=EDGE_CURVE('',#6570,#6570,#1992,.T.);
#8425=EDGE_CURVE('',#6570,#6571,#4868,.T.);
#8426=EDGE_CURVE('',#6571,#6564,#1993,.T.);
#8427=EDGE_CURVE('',#6569,#6571,#1994,.T.);
#8428=EDGE_CURVE('',#6561,#6567,#1995,.T.);
#8429=EDGE_CURVE('',#6572,#6570,#4869,.T.);
#8430=EDGE_CURVE('',#6573,#6573,#1996,.T.);
#8431=EDGE_CURVE('',#6573,#6574,#4870,.T.);
#8432=EDGE_CURVE('',#6574,#6574,#1997,.T.);
#8433=EDGE_CURVE('',#6575,#6576,#409,.T.);
#8434=EDGE_CURVE('',#6558,#6575,#4871,.T.);
#8435=EDGE_CURVE('',#6577,#6557,#410,.T.);
#8436=EDGE_CURVE('',#6578,#6577,#411,.T.);
#8437=EDGE_CURVE('',#6576,#6578,#412,.T.);
#8438=EDGE_CURVE('',#6576,#6574,#4872,.T.);
#8439=EDGE_CURVE('',#6579,#6544,#413,.T.);
#8440=EDGE_CURVE('',#6580,#6579,#414,.T.);
#8441=EDGE_CURVE('',#6581,#6580,#415,.T.);
#8442=EDGE_CURVE('',#6545,#6581,#4873,.T.);
#8443=EDGE_CURVE('',#6545,#6582,#4874,.T.);
#8444=EDGE_CURVE('',#6582,#6582,#1998,.T.);
#8445=EDGE_CURVE('',#6582,#6583,#4875,.T.);
#8446=EDGE_CURVE('',#6583,#6583,#1999,.T.);
#8447=EDGE_CURVE('',#6577,#6580,#416,.T.);
#8448=EDGE_CURVE('',#6578,#6579,#417,.T.);
#8449=EDGE_CURVE('',#6559,#6575,#4876,.T.);
#8450=EDGE_CURVE('',#6581,#6546,#4877,.T.);
#8451=EDGE_CURVE('',#6584,#6584,#2000,.T.);
#8452=EDGE_CURVE('',#6585,#6585,#2001,.T.);
#8453=EDGE_CURVE('',#6585,#6584,#4878,.T.);
#8454=EDGE_CURVE('',#6586,#6586,#2002,.T.);
#8455=EDGE_CURVE('',#6586,#6585,#4879,.T.);
#8456=EDGE_CURVE('',#6587,#6587,#2003,.T.);
#8457=EDGE_CURVE('',#6588,#6588,#2004,.T.);
#8458=EDGE_CURVE('',#6588,#6587,#4880,.T.);
#8459=EDGE_CURVE('',#6589,#6589,#2005,.T.);
#8460=EDGE_CURVE('',#6589,#6588,#4881,.T.);
#8461=EDGE_CURVE('',#6590,#6590,#2006,.T.);
#8462=EDGE_CURVE('',#6591,#6591,#2007,.T.);
#8463=EDGE_CURVE('',#6591,#6590,#4882,.T.);
#8464=EDGE_CURVE('',#6591,#6592,#4883,.T.);
#8465=EDGE_CURVE('',#6592,#6592,#2008,.T.);
#8466=EDGE_CURVE('',#6593,#6593,#2009,.T.);
#8467=EDGE_CURVE('',#6594,#6594,#2010,.T.);
#8468=EDGE_CURVE('',#6594,#6593,#4884,.T.);
#8469=EDGE_CURVE('',#6594,#6595,#4885,.T.);
#8470=EDGE_CURVE('',#6595,#6595,#2011,.T.);
#11531=ORIENTED_EDGE('',*,*,#8387,.F.);
#11532=ORIENTED_EDGE('',*,*,#8388,.T.);
#11533=ORIENTED_EDGE('',*,*,#8389,.T.);
#11534=ORIENTED_EDGE('',*,*,#8390,.T.);
#11535=ORIENTED_EDGE('',*,*,#8391,.T.);
#11536=ORIENTED_EDGE('',*,*,#8392,.F.);
#11537=ORIENTED_EDGE('',*,*,#8393,.T.);
#11538=ORIENTED_EDGE('',*,*,#8387,.T.);
#11539=ORIENTED_EDGE('',*,*,#8394,.T.);
#11540=ORIENTED_EDGE('',*,*,#8395,.F.);
#11541=ORIENTED_EDGE('',*,*,#8396,.T.);
#11542=ORIENTED_EDGE('',*,*,#8392,.T.);
#11543=ORIENTED_EDGE('',*,*,#8397,.T.);
#11544=ORIENTED_EDGE('',*,*,#8398,.F.);
#11545=ORIENTED_EDGE('',*,*,#8399,.T.);
#11546=ORIENTED_EDGE('',*,*,#8395,.T.);
#11547=ORIENTED_EDGE('',*,*,#8400,.T.);
#11548=ORIENTED_EDGE('',*,*,#8401,.F.);
#11549=ORIENTED_EDGE('',*,*,#8402,.T.);
#11550=ORIENTED_EDGE('',*,*,#8398,.T.);
#11551=ORIENTED_EDGE('',*,*,#8403,.T.);
#11552=ORIENTED_EDGE('',*,*,#8404,.F.);
#11553=ORIENTED_EDGE('',*,*,#8405,.T.);
#11554=ORIENTED_EDGE('',*,*,#8401,.T.);
#11555=ORIENTED_EDGE('',*,*,#8406,.T.);
#11556=ORIENTED_EDGE('',*,*,#8404,.T.);
#11557=ORIENTED_EDGE('',*,*,#8407,.T.);
#11558=ORIENTED_EDGE('',*,*,#8408,.T.);
#11559=ORIENTED_EDGE('',*,*,#8409,.T.);
#11560=ORIENTED_EDGE('',*,*,#8410,.T.);
#11561=ORIENTED_EDGE('',*,*,#8411,.F.);
#11562=ORIENTED_EDGE('',*,*,#8412,.T.);
#11563=ORIENTED_EDGE('',*,*,#8413,.F.);
#11564=ORIENTED_EDGE('',*,*,#8414,.F.);
#11565=ORIENTED_EDGE('',*,*,#8415,.F.);
#11566=ORIENTED_EDGE('',*,*,#8416,.F.);
#11567=ORIENTED_EDGE('',*,*,#8413,.T.);
#11568=ORIENTED_EDGE('',*,*,#8417,.T.);
#11569=ORIENTED_EDGE('',*,*,#8418,.F.);
#11570=ORIENTED_EDGE('',*,*,#8419,.F.);
#11571=ORIENTED_EDGE('',*,*,#8420,.F.);
#11572=ORIENTED_EDGE('',*,*,#8421,.F.);
#11573=ORIENTED_EDGE('',*,*,#8418,.T.);
#11574=ORIENTED_EDGE('',*,*,#8422,.T.);
#11575=ORIENTED_EDGE('',*,*,#8423,.F.);
#11576=ORIENTED_EDGE('',*,*,#8422,.F.);
#11577=ORIENTED_EDGE('',*,*,#8417,.F.);
#11578=ORIENTED_EDGE('',*,*,#8412,.F.);
#11579=ORIENTED_EDGE('',*,*,#8424,.F.);
#11580=ORIENTED_EDGE('',*,*,#8425,.T.);
#11581=ORIENTED_EDGE('',*,*,#8426,.T.);
#11582=ORIENTED_EDGE('',*,*,#8414,.T.);
#11583=ORIENTED_EDGE('',*,*,#8416,.T.);
#11584=ORIENTED_EDGE('',*,*,#8421,.T.);
#11585=ORIENTED_EDGE('',*,*,#8427,.T.);
#11586=ORIENTED_EDGE('',*,*,#8425,.F.);
#11587=ORIENTED_EDGE('',*,*,#8415,.T.);
#11588=ORIENTED_EDGE('',*,*,#8426,.F.);
#11589=ORIENTED_EDGE('',*,*,#8427,.F.);
#11590=ORIENTED_EDGE('',*,*,#8420,.T.);
#11591=ORIENTED_EDGE('',*,*,#8428,.F.);
#11592=ORIENTED_EDGE('',*,*,#8429,.T.);
#11593=ORIENTED_EDGE('',*,*,#8424,.T.);
#11594=ORIENTED_EDGE('',*,*,#8429,.F.);
#11595=ORIENTED_EDGE('',*,*,#8430,.F.);
#11596=ORIENTED_EDGE('',*,*,#8431,.T.);
#11597=ORIENTED_EDGE('',*,*,#8432,.T.);
#11598=ORIENTED_EDGE('',*,*,#8431,.F.);
#11599=ORIENTED_EDGE('',*,*,#8433,.F.);
#11600=ORIENTED_EDGE('',*,*,#8434,.F.);
#11601=ORIENTED_EDGE('',*,*,#8408,.F.);
#11602=ORIENTED_EDGE('',*,*,#8435,.F.);
#11603=ORIENTED_EDGE('',*,*,#8436,.F.);
#11604=ORIENTED_EDGE('',*,*,#8437,.F.);
#11605=ORIENTED_EDGE('',*,*,#8438,.T.);
#11606=ORIENTED_EDGE('',*,*,#8432,.F.);
#11607=ORIENTED_EDGE('',*,*,#8438,.F.);
#11608=ORIENTED_EDGE('',*,*,#8389,.F.);
#11609=ORIENTED_EDGE('',*,*,#8439,.F.);
#11610=ORIENTED_EDGE('',*,*,#8440,.F.);
#11611=ORIENTED_EDGE('',*,*,#8441,.F.);
#11612=ORIENTED_EDGE('',*,*,#8442,.F.);
#11613=ORIENTED_EDGE('',*,*,#8443,.T.);
#11614=ORIENTED_EDGE('',*,*,#8444,.T.);
#11615=ORIENTED_EDGE('',*,*,#8443,.F.);
#11616=ORIENTED_EDGE('',*,*,#8444,.F.);
#11617=ORIENTED_EDGE('',*,*,#8445,.T.);
#11618=ORIENTED_EDGE('',*,*,#8446,.T.);
#11619=ORIENTED_EDGE('',*,*,#8445,.F.);
#11620=ORIENTED_EDGE('',*,*,#8436,.T.);
#11621=ORIENTED_EDGE('',*,*,#8447,.T.);
#11622=ORIENTED_EDGE('',*,*,#8440,.T.);
#11623=ORIENTED_EDGE('',*,*,#8448,.F.);
#11624=ORIENTED_EDGE('',*,*,#8433,.T.);
#11625=ORIENTED_EDGE('',*,*,#8437,.T.);
#11626=ORIENTED_EDGE('',*,*,#8448,.T.);
#11627=ORIENTED_EDGE('',*,*,#8439,.T.);
#11628=ORIENTED_EDGE('',*,*,#8388,.F.);
#11629=ORIENTED_EDGE('',*,*,#8393,.F.);
#11630=ORIENTED_EDGE('',*,*,#8396,.F.);
#11631=ORIENTED_EDGE('',*,*,#8399,.F.);
#11632=ORIENTED_EDGE('',*,*,#8402,.F.);
#11633=ORIENTED_EDGE('',*,*,#8405,.F.);
#11634=ORIENTED_EDGE('',*,*,#8410,.F.);
#11635=ORIENTED_EDGE('',*,*,#8449,.T.);
#11636=ORIENTED_EDGE('',*,*,#8434,.T.);
#11637=ORIENTED_EDGE('',*,*,#8449,.F.);
#11638=ORIENTED_EDGE('',*,*,#8409,.F.);
#11639=ORIENTED_EDGE('',*,*,#8435,.T.);
#11640=ORIENTED_EDGE('',*,*,#8407,.F.);
#11641=ORIENTED_EDGE('',*,*,#8406,.F.);
#11642=ORIENTED_EDGE('',*,*,#8403,.F.);
#11643=ORIENTED_EDGE('',*,*,#8400,.F.);
#11644=ORIENTED_EDGE('',*,*,#8397,.F.);
#11645=ORIENTED_EDGE('',*,*,#8394,.F.);
#11646=ORIENTED_EDGE('',*,*,#8391,.F.);
#11647=ORIENTED_EDGE('',*,*,#8450,.F.);
#11648=ORIENTED_EDGE('',*,*,#8441,.T.);
#11649=ORIENTED_EDGE('',*,*,#8447,.F.);
#11650=ORIENTED_EDGE('',*,*,#8442,.T.);
#11651=ORIENTED_EDGE('',*,*,#8450,.T.);
#11652=ORIENTED_EDGE('',*,*,#8390,.F.);
#11653=ORIENTED_EDGE('',*,*,#8451,.F.);
#11654=ORIENTED_EDGE('',*,*,#8452,.F.);
#11655=ORIENTED_EDGE('',*,*,#8453,.T.);
#11656=ORIENTED_EDGE('',*,*,#8451,.T.);
#11657=ORIENTED_EDGE('',*,*,#8453,.F.);
#11658=ORIENTED_EDGE('',*,*,#8454,.F.);
#11659=ORIENTED_EDGE('',*,*,#8455,.T.);
#11660=ORIENTED_EDGE('',*,*,#8452,.T.);
#11661=ORIENTED_EDGE('',*,*,#8455,.F.);
#11662=ORIENTED_EDGE('',*,*,#8456,.F.);
#11663=ORIENTED_EDGE('',*,*,#8454,.T.);
#11664=ORIENTED_EDGE('',*,*,#8457,.F.);
#11665=ORIENTED_EDGE('',*,*,#8458,.T.);
#11666=ORIENTED_EDGE('',*,*,#8456,.T.);
#11667=ORIENTED_EDGE('',*,*,#8458,.F.);
#11668=ORIENTED_EDGE('',*,*,#8459,.F.);
#11669=ORIENTED_EDGE('',*,*,#8460,.T.);
#11670=ORIENTED_EDGE('',*,*,#8457,.T.);
#11671=ORIENTED_EDGE('',*,*,#8460,.F.);
#11672=ORIENTED_EDGE('',*,*,#8459,.T.);
#11673=ORIENTED_EDGE('',*,*,#8446,.F.);
#11674=ORIENTED_EDGE('',*,*,#8461,.F.);
#11675=ORIENTED_EDGE('',*,*,#8430,.T.);
#11676=ORIENTED_EDGE('',*,*,#8462,.F.);
#11677=ORIENTED_EDGE('',*,*,#8463,.T.);
#11678=ORIENTED_EDGE('',*,*,#8461,.T.);
#11679=ORIENTED_EDGE('',*,*,#8463,.F.);
#11680=ORIENTED_EDGE('',*,*,#8462,.T.);
#11681=ORIENTED_EDGE('',*,*,#8464,.T.);
#11682=ORIENTED_EDGE('',*,*,#8465,.F.);
#11683=ORIENTED_EDGE('',*,*,#8464,.F.);
#11684=ORIENTED_EDGE('',*,*,#8465,.T.);
#11685=ORIENTED_EDGE('',*,*,#8466,.F.);
#11686=ORIENTED_EDGE('',*,*,#8467,.F.);
#11687=ORIENTED_EDGE('',*,*,#8468,.T.);
#11688=ORIENTED_EDGE('',*,*,#8466,.T.);
#11689=ORIENTED_EDGE('',*,*,#8468,.F.);
#11690=ORIENTED_EDGE('',*,*,#8467,.T.);
#11691=ORIENTED_EDGE('',*,*,#8469,.T.);
#11692=ORIENTED_EDGE('',*,*,#8470,.F.);
#11693=ORIENTED_EDGE('',*,*,#8469,.F.);
#11694=ORIENTED_EDGE('',*,*,#8470,.T.);
#11695=ORIENTED_EDGE('',*,*,#8411,.T.);
#11696=ORIENTED_EDGE('',*,*,#8428,.T.);
#11697=ORIENTED_EDGE('',*,*,#8419,.T.);
#11698=ORIENTED_EDGE('',*,*,#8423,.T.);
#14642=PLANE('',#16429);
#14643=PLANE('',#16430);
#14644=PLANE('',#16432);
#14645=PLANE('',#16433);
#14646=PLANE('',#16449);
#14647=PLANE('',#16450);
#14648=PLANE('',#16451);
#14649=PLANE('',#16457);
#14650=PLANE('',#16463);
#14651=PLANE('',#16464);
#14652=PLANE('',#16470);
#14653=PLANE('',#16476);
#15087=ADVANCED_FACE('',(#2731),#1432,.T.);
#15088=ADVANCED_FACE('',(#2732),#1433,.T.);
#15089=ADVANCED_FACE('',(#2733),#1434,.T.);
#15090=ADVANCED_FACE('',(#2734),#1435,.T.);
#15091=ADVANCED_FACE('',(#2735),#1436,.T.);
#15092=ADVANCED_FACE('',(#2736),#1437,.T.);
#15093=ADVANCED_FACE('',(#2737),#1438,.T.);
#15094=ADVANCED_FACE('',(#2738),#14642,.F.);
#15095=ADVANCED_FACE('',(#2739),#14643,.F.);
#15096=ADVANCED_FACE('',(#2740),#14644,.F.);
#15097=ADVANCED_FACE('',(#2741),#14645,.F.);
#15098=ADVANCED_FACE('',(#2742),#1439,.F.);
#15099=ADVANCED_FACE('',(#2743),#1227,.F.);
#15100=ADVANCED_FACE('',(#2744),#1228,.F.);
#15101=ADVANCED_FACE('',(#2745),#1440,.T.);
#15102=ADVANCED_FACE('',(#2746),#1229,.T.);
#15103=ADVANCED_FACE('',(#2747),#1230,.T.);
#15104=ADVANCED_FACE('',(#2748),#1441,.T.);
#15105=ADVANCED_FACE('',(#2749),#161,.T.);
#15106=ADVANCED_FACE('',(#2750),#162,.T.);
#15107=ADVANCED_FACE('',(#2751),#14646,.T.);
#15108=ADVANCED_FACE('',(#2752),#163,.T.);
#15109=ADVANCED_FACE('',(#2753),#14647,.T.);
#15110=ADVANCED_FACE('',(#2754),#14648,.T.);
#15111=ADVANCED_FACE('',(#2755),#1231,.T.);
#15112=ADVANCED_FACE('',(#2756),#1442,.T.);
#15113=ADVANCED_FACE('',(#2757,#1699),#14649,.T.);
#15114=ADVANCED_FACE('',(#2758),#1232,.T.);
#15115=ADVANCED_FACE('',(#2759),#1443,.T.);
#15116=ADVANCED_FACE('',(#2760,#1700),#14650,.T.);
#15117=ADVANCED_FACE('',(#2761,#1701),#14651,.T.);
#15118=ADVANCED_FACE('',(#2762),#1444,.T.);
#15119=ADVANCED_FACE('',(#2763),#1233,.T.);
#15120=ADVANCED_FACE('',(#2764,#1702),#14652,.T.);
#15121=ADVANCED_FACE('',(#2765),#1445,.T.);
#15122=ADVANCED_FACE('',(#2766),#1234,.T.);
#15123=ADVANCED_FACE('',(#2767,#1703),#14653,.T.);
#15616=CLOSED_SHELL('',(#15087,#15088,#15089,#15090,#15091,#15092,#15093,
#15094,#15095,#15096,#15097,#15098,#15099,#15100,#15101,#15102,#15103,#15104,
#15105,#15106,#15107,#15108,#15109,#15110,#15111,#15112,#15113,#15114,#15115,
#15116,#15117,#15118,#15119,#15120,#15121,#15122,#15123));
#16419=AXIS2_PLACEMENT_3D('',#23121,#19033,#19034);
#16420=AXIS2_PLACEMENT_3D('',#23122,#19035,#19036);
#16421=AXIS2_PLACEMENT_3D('',#23190,#19038,#19039);
#16422=AXIS2_PLACEMENT_3D('',#23199,#19041,#19042);
#16423=AXIS2_PLACEMENT_3D('',#23319,#19044,#19045);
#16424=AXIS2_PLACEMENT_3D('',#23449,#19047,#19048);
#16425=AXIS2_PLACEMENT_3D('',#23589,#19050,#19051);
#16426=AXIS2_PLACEMENT_3D('',#23719,#19053,#19054);
#16427=AXIS2_PLACEMENT_3D('',#23843,#19056,#19057);
#16428=AXIS2_PLACEMENT_3D('',#23904,#19058,#19059);
#16429=AXIS2_PLACEMENT_3D('',#23933,#19061,#19062);
#16430=AXIS2_PLACEMENT_3D('',#23946,#19067,#19068);
#16431=AXIS2_PLACEMENT_3D('',#23948,#19069,#19070);
#16432=AXIS2_PLACEMENT_3D('',#23952,#19073,#19074);
#16433=AXIS2_PLACEMENT_3D('',#23962,#19078,#19079);
#16434=AXIS2_PLACEMENT_3D('',#23964,#19081,#19082);
#16435=AXIS2_PLACEMENT_3D('',#23966,#19083,#19084);
#16436=AXIS2_PLACEMENT_3D('',#23969,#19086,#19087);
#16437=AXIS2_PLACEMENT_3D('',#23970,#19088,#19089);
#16438=AXIS2_PLACEMENT_3D('',#23971,#19090,#19091);
#16439=AXIS2_PLACEMENT_3D('',#23972,#19092,#19093);
#16440=AXIS2_PLACEMENT_3D('',#23973,#19094,#19095);
#16441=AXIS2_PLACEMENT_3D('',#23976,#19097,#19098);
#16442=AXIS2_PLACEMENT_3D('',#23978,#19099,#19100);
#16443=AXIS2_PLACEMENT_3D('',#23981,#19102,#19103);
#16444=AXIS2_PLACEMENT_3D('',#23982,#19104,#19105);
#16445=AXIS2_PLACEMENT_3D('',#24205,#19108,#19109);
#16446=AXIS2_PLACEMENT_3D('',#24270,#19112,#19113);
#16447=AXIS2_PLACEMENT_3D('',#24271,#19114,#19115);
#16448=AXIS2_PLACEMENT_3D('',#24274,#19117,#19118);
#16449=AXIS2_PLACEMENT_3D('',#26137,#19120,#19121);
#16450=AXIS2_PLACEMENT_3D('',#26763,#19123,#19124);
#16451=AXIS2_PLACEMENT_3D('',#26764,#19125,#19126);
#16452=AXIS2_PLACEMENT_3D('',#26766,#19127,#19128);
#16453=AXIS2_PLACEMENT_3D('',#26767,#19129,#19130);
#16454=AXIS2_PLACEMENT_3D('',#26769,#19131,#19132);
#16455=AXIS2_PLACEMENT_3D('',#26771,#19134,#19135);
#16456=AXIS2_PLACEMENT_3D('',#26773,#19136,#19137);
#16457=AXIS2_PLACEMENT_3D('',#26775,#19139,#19140);
#16458=AXIS2_PLACEMENT_3D('',#26777,#19141,#19142);
#16459=AXIS2_PLACEMENT_3D('',#26778,#19143,#19144);
#16460=AXIS2_PLACEMENT_3D('',#26780,#19145,#19146);
#16461=AXIS2_PLACEMENT_3D('',#26782,#19148,#19149);
#16462=AXIS2_PLACEMENT_3D('',#26784,#19150,#19151);
#16463=AXIS2_PLACEMENT_3D('',#26786,#19153,#19154);
#16464=AXIS2_PLACEMENT_3D('',#26787,#19155,#19156);
#16465=AXIS2_PLACEMENT_3D('',#26789,#19157,#19158);
#16466=AXIS2_PLACEMENT_3D('',#26790,#19159,#19160);
#16467=AXIS2_PLACEMENT_3D('',#26792,#19161,#19162);
#16468=AXIS2_PLACEMENT_3D('',#26794,#19164,#19165);
#16469=AXIS2_PLACEMENT_3D('',#26797,#19167,#19168);
#16470=AXIS2_PLACEMENT_3D('',#26798,#19169,#19170);
#16471=AXIS2_PLACEMENT_3D('',#26800,#19171,#19172);
#16472=AXIS2_PLACEMENT_3D('',#26801,#19173,#19174);
#16473=AXIS2_PLACEMENT_3D('',#26803,#19175,#19176);
#16474=AXIS2_PLACEMENT_3D('',#26805,#19178,#19179);
#16475=AXIS2_PLACEMENT_3D('',#26808,#19181,#19182);
#16476=AXIS2_PLACEMENT_3D('',#26809,#19183,#19184);
#19033=DIRECTION('axis',(0.,0.,1.));
#19034=DIRECTION('refdir',(1.,0.,0.));
#19035=DIRECTION('center_axis',(-1.,0.,0.));
#19036=DIRECTION('ref_axis',(0.,0.437755261071371,0.899094172711811));
#19037=DIRECTION('',(1.,0.,0.));
#19038=DIRECTION('center_axis',(-1.,0.,0.));
#19039=DIRECTION('ref_axis',(0.,0.,1.));
#19040=DIRECTION('',(-1.,2.62207686119176E-10,0.));
#19041=DIRECTION('center_axis',(-1.,0.,0.));
#19042=DIRECTION('ref_axis',(0.,0.297498178236103,0.954722385799244));
#19043=DIRECTION('',(1.,0.,0.));
#19044=DIRECTION('center_axis',(-1.,0.,0.));
#19045=DIRECTION('ref_axis',(0.,0.297498178236103,0.954722385799244));
#19046=DIRECTION('',(1.,0.,0.));
#19047=DIRECTION('center_axis',(-1.,0.,0.));
#19048=DIRECTION('ref_axis',(0.,0.297498178236103,0.954722385799244));
#19049=DIRECTION('',(1.,0.,0.));
#19050=DIRECTION('center_axis',(-1.,0.,0.));
#19051=DIRECTION('ref_axis',(0.,0.297498178236103,0.954722385799244));
#19052=DIRECTION('',(1.,0.,0.));
#19053=DIRECTION('center_axis',(-1.,0.,0.));
#19054=DIRECTION('ref_axis',(0.,0.297498178236103,0.954722385799244));
#19055=DIRECTION('',(1.,0.,0.));
#19056=DIRECTION('center_axis',(-1.,0.,0.));
#19057=DIRECTION('ref_axis',(0.,-0.150453659663836,0.988617062513974));
#19058=DIRECTION('center_axis',(1.,0.,0.));
#19059=DIRECTION('ref_axis',(0.,0.,1.));
#19060=DIRECTION('',(1.,0.,0.));
#19061=DIRECTION('center_axis',(0.,-1.,0.));
#19062=DIRECTION('ref_axis',(1.,0.,0.));
#19063=DIRECTION('',(0.,0.,-1.));
#19064=DIRECTION('',(1.,0.,0.));
#19065=DIRECTION('',(0.,0.,1.));
#19066=DIRECTION('',(1.,0.,0.));
#19067=DIRECTION('center_axis',(1.,0.,0.));
#19068=DIRECTION('ref_axis',(0.,1.,0.));
#19069=DIRECTION('center_axis',(-1.,0.,0.));
#19070=DIRECTION('ref_axis',(0.,0.,1.));
#19071=DIRECTION('',(0.,1.,0.));
#19072=DIRECTION('',(0.,0.,1.));
#19073=DIRECTION('center_axis',(0.,1.,0.));
#19074=DIRECTION('ref_axis',(-1.,0.,0.));
#19075=DIRECTION('',(0.,0.,1.));
#19076=DIRECTION('',(-1.,0.,0.));
#19077=DIRECTION('',(-1.,0.,0.));
#19078=DIRECTION('center_axis',(0.,0.,1.));
#19079=DIRECTION('ref_axis',(1.,0.,0.));
#19080=DIRECTION('',(0.,-1.,0.));
#19081=DIRECTION('center_axis',(-1.,0.,0.));
#19082=DIRECTION('ref_axis',(0.,0.,1.));
#19083=DIRECTION('center_axis',(-1.,0.,0.));
#19084=DIRECTION('ref_axis',(0.,0.,1.));
#19085=DIRECTION('',(-1.,0.,0.));
#19086=DIRECTION('center_axis',(-1.,0.,0.));
#19087=DIRECTION('ref_axis',(0.,0.,1.));
#19088=DIRECTION('center_axis',(-1.,0.,0.));
#19089=DIRECTION('ref_axis',(0.,0.,1.));
#19090=DIRECTION('center_axis',(-1.,0.,0.));
#19091=DIRECTION('ref_axis',(0.,-1.22464679914735E-16,-1.));
#19092=DIRECTION('center_axis',(1.,0.,0.));
#19093=DIRECTION('ref_axis',(0.,0.,1.));
#19094=DIRECTION('center_axis',(-1.,0.,0.));
#19095=DIRECTION('ref_axis',(0.,0.,1.));
#19096=DIRECTION('',(-0.515038074910058,-1.04972719113862E-16,-0.85716730070211));
#19097=DIRECTION('center_axis',(-1.,0.,0.));
#19098=DIRECTION('ref_axis',(0.,0.,1.));
#19099=DIRECTION('center_axis',(-1.,0.,0.));
#19100=DIRECTION('ref_axis',(0.,0.,1.));
#19101=DIRECTION('',(1.,0.,0.));
#19102=DIRECTION('center_axis',(-1.,0.,0.));
#19103=DIRECTION('ref_axis',(0.,0.,1.));
#19104=DIRECTION('center_axis',(1.,0.,0.));
#19105=DIRECTION('ref_axis',(0.,0.,1.));
#19106=DIRECTION('',(0.701238976116887,0.,0.712926292385503));
#19107=DIRECTION('',(-0.701238976116887,-8.73082901997896E-17,0.712926292385503));
#19108=DIRECTION('center_axis',(-1.,0.,0.));
#19109=DIRECTION('ref_axis',(0.,0.,1.));
#19110=DIRECTION('',(-0.701238976116887,1.83871647159407E-10,-0.712926292385503));
#19111=DIRECTION('',(0.701238976116887,8.73082901997896E-17,0.712926292385503));
#19112=DIRECTION('center_axis',(-1.,0.,0.));
#19113=DIRECTION('ref_axis',(0.,0.,1.));
#19114=DIRECTION('center_axis',(-1.,0.,0.));
#19115=DIRECTION('ref_axis',(0.,0.,1.));
#19116=DIRECTION('',(1.,0.,0.));
#19117=DIRECTION('center_axis',(-1.,0.,0.));
#19118=DIRECTION('ref_axis',(0.,0.,1.));
#19119=DIRECTION('',(-0.342020143325669,0.,0.939692620785908));
#19120=DIRECTION('center_axis',(0.,1.,0.));
#19121=DIRECTION('ref_axis',(1.,0.,0.));
#19122=DIRECTION('',(-0.34202014332565,8.96784698282884E-11,0.939692620785916));
#19123=DIRECTION('center_axis',(2.62207686119176E-10,1.,1.96067283990894E-15));
#19124=DIRECTION('ref_axis',(2.49435711265653E-42,-1.96067283990894E-15,
1.));
#19125=DIRECTION('center_axis',(1.,0.,0.));
#19126=DIRECTION('ref_axis',(0.,0.,-1.));
#19127=DIRECTION('center_axis',(-1.,0.,0.));
#19128=DIRECTION('ref_axis',(0.,0.,1.));
#19129=DIRECTION('center_axis',(-1.,0.,0.));
#19130=DIRECTION('ref_axis',(0.,0.,1.));
#19131=DIRECTION('center_axis',(-1.,0.,0.));
#19132=DIRECTION('ref_axis',(0.,0.,1.));
#19133=DIRECTION('',(0.70710678118654,8.65956056235503E-17,0.707106781186555));
#19134=DIRECTION('center_axis',(-1.,0.,0.));
#19135=DIRECTION('ref_axis',(0.,0.,1.));
#19136=DIRECTION('center_axis',(-1.,0.,0.));
#19137=DIRECTION('ref_axis',(0.,0.,1.));
#19138=DIRECTION('',(1.,0.,0.));
#19139=DIRECTION('center_axis',(1.,0.,0.));
#19140=DIRECTION('ref_axis',(0.,0.,-1.));
#19141=DIRECTION('center_axis',(-1.,0.,0.));
#19142=DIRECTION('ref_axis',(0.,0.,1.));
#19143=DIRECTION('center_axis',(-1.,0.,0.));
#19144=DIRECTION('ref_axis',(0.,0.,1.));
#19145=DIRECTION('center_axis',(-1.,0.,0.));
#19146=DIRECTION('ref_axis',(0.,0.,1.));
#19147=DIRECTION('',(0.707106781186548,8.65956056235493E-17,0.707106781186547));
#19148=DIRECTION('center_axis',(-1.,0.,0.));
#19149=DIRECTION('ref_axis',(0.,0.,1.));
#19150=DIRECTION('center_axis',(-1.,0.,0.));
#19151=DIRECTION('ref_axis',(0.,0.,1.));
#19152=DIRECTION('',(1.,0.,0.));
#19153=DIRECTION('center_axis',(-1.,0.,0.));
#19154=DIRECTION('ref_axis',(0.,0.,1.));
#19155=DIRECTION('center_axis',(1.,0.,0.));
#19156=DIRECTION('ref_axis',(0.,0.,-1.));
#19157=DIRECTION('center_axis',(-1.,0.,0.));
#19158=DIRECTION('ref_axis',(0.,0.,1.));
#19159=DIRECTION('center_axis',(-1.,0.,0.));
#19160=DIRECTION('ref_axis',(0.,0.,1.));
#19161=DIRECTION('center_axis',(-1.,0.,0.));
#19162=DIRECTION('ref_axis',(0.,0.,1.));
#19163=DIRECTION('',(1.,0.,0.));
#19164=DIRECTION('center_axis',(1.,0.,0.));
#19165=DIRECTION('ref_axis',(0.,0.,1.));
#19166=DIRECTION('',(-0.707106781186548,-8.65956056235493E-17,0.707106781186547));
#19167=DIRECTION('center_axis',(-1.,0.,0.));
#19168=DIRECTION('ref_axis',(0.,0.,1.));
#19169=DIRECTION('center_axis',(-1.,0.,0.));
#19170=DIRECTION('ref_axis',(0.,0.,1.));
#19171=DIRECTION('center_axis',(-1.,0.,0.));
#19172=DIRECTION('ref_axis',(0.,0.,1.));
#19173=DIRECTION('center_axis',(-1.,0.,0.));
#19174=DIRECTION('ref_axis',(0.,0.,1.));
#19175=DIRECTION('center_axis',(-1.,0.,0.));
#19176=DIRECTION('ref_axis',(0.,0.,1.));
#19177=DIRECTION('',(1.,0.,0.));
#19178=DIRECTION('center_axis',(1.,0.,0.));
#19179=DIRECTION('ref_axis',(0.,0.,1.));
#19180=DIRECTION('',(-0.70710678118654,-8.65956056235503E-17,0.707106781186555));
#19181=DIRECTION('center_axis',(-1.,0.,0.));
#19182=DIRECTION('ref_axis',(0.,0.,1.));
#19183=DIRECTION('center_axis',(-1.,0.,0.));
#19184=DIRECTION('ref_axis',(0.,0.,1.));
#23121=CARTESIAN_POINT('',(0.,0.,0.));
#23122=CARTESIAN_POINT('Origin',(0.,0.,13.5));
#23123=CARTESIAN_POINT('',(2.22083974265588,-0.416497439768541,12.1633886568391));
#23124=CARTESIAN_POINT('',(2.40093257836374,-0.416497469208933,12.163388666013));
#23125=CARTESIAN_POINT('',(0.,-0.416497449530544,12.1633886598811));
#23126=CARTESIAN_POINT('',(3.11803278688524,-0.795264618259144,12.3478046229284));
#23127=CARTESIAN_POINT('Ctrl Pts',(2.22083974265588,-0.41649743976857,12.1633886568392));
#23128=CARTESIAN_POINT('Ctrl Pts',(2.2220583526003,-0.405658322369837,12.1600111120734));
#23129=CARTESIAN_POINT('Ctrl Pts',(2.22327782186277,-0.394773680664366,
12.1567640315656));
#23130=CARTESIAN_POINT('Ctrl Pts',(2.22938824338899,-0.34005543600158,12.141163821239));
#23131=CARTESIAN_POINT('Ctrl Pts',(2.23428033926222,-0.295682000890378,
12.1308230099316));
#23132=CARTESIAN_POINT('Ctrl Pts',(2.24895685570008,-0.161170286254102,
12.10632153116));
#23133=CARTESIAN_POINT('Ctrl Pts',(2.25866610420412,-0.070073656053006,
12.0987841785454));
#23134=CARTESIAN_POINT('Ctrl Pts',(2.27331012373895,0.0668268643511414,
12.1008485412387));
#23135=CARTESIAN_POINT('Ctrl Pts',(2.27820301388258,0.112483216940743,12.1037772244606));
#23136=CARTESIAN_POINT('Ctrl Pts',(2.29279615275694,0.24770334958519,12.1191273943385));
#23137=CARTESIAN_POINT('Ctrl Pts',(2.30249930101493,0.336296155354615,12.1379899977253));
#23138=CARTESIAN_POINT('Ctrl Pts',(2.3206444637074,0.497852571538328,12.1891233324526));
#23139=CARTESIAN_POINT('Ctrl Pts',(2.3290677605188,0.571096236923704,12.2193345192887));
#23140=CARTESIAN_POINT('Ctrl Pts',(2.34241546071034,0.681984453214291,12.2764877494031));
#23141=CARTESIAN_POINT('Ctrl Pts',(2.34730489916618,0.721524101820936,12.2993802178688));
#23142=CARTESIAN_POINT('Ctrl Pts',(2.36188217783804,0.83563462320767,12.3731230947425));
#23143=CARTESIAN_POINT('Ctrl Pts',(2.3715671462109,0.906487948408386,12.4292913789087));
#23144=CARTESIAN_POINT('Ctrl Pts',(2.39082504161259,1.036075619433,12.5541652941715));
#23145=CARTESIAN_POINT('Ctrl Pts',(2.40038146080491,1.09456759418981,12.6225162833593));
#23146=CARTESIAN_POINT('Ctrl Pts',(2.41973055679119,1.19830818950665,12.7703988020955));
#23147=CARTESIAN_POINT('Ctrl Pts',(2.42948098070764,1.24313391978949,12.8497092131317));
#23148=CARTESIAN_POINT('Ctrl Pts',(2.45867561213097,1.35340306175113,13.098545263797));
#23149=CARTESIAN_POINT('Ctrl Pts',(2.47789933184414,1.39396340856472,13.2769907630923));
#23150=CARTESIAN_POINT('Ctrl Pts',(2.50712132114416,1.40210544760839,13.5495874517168));
#23151=CARTESIAN_POINT('Ctrl Pts',(2.51687140626553,1.39587676776904,13.6410204447446));
#23152=CARTESIAN_POINT('Ctrl Pts',(2.53643597386339,1.36570547636464,13.8212170813072));
#23153=CARTESIAN_POINT('Ctrl Pts',(2.54621714872809,1.34186370907104,13.9095525151614));
#23154=CARTESIAN_POINT('Ctrl Pts',(2.57551273484634,1.24530587458394,14.1650438428224));
#23155=CARTESIAN_POINT('Ctrl Pts',(2.59470675330616,1.14848483177222,14.3210067294209));
#23156=CARTESIAN_POINT('Ctrl Pts',(2.62394307084879,0.962900170700194,14.5202981151465));
#23157=CARTESIAN_POINT('Ctrl Pts',(2.63364712817475,0.894970769260525,14.5803762919486));
#23158=CARTESIAN_POINT('Ctrl Pts',(2.6482121350503,0.78480653483361,14.6602402565328));
#23159=CARTESIAN_POINT('Ctrl Pts',(2.65308657104942,0.746607731332198,14.6851816883857));
#23160=CARTESIAN_POINT('Ctrl Pts',(2.66774732143052,0.628442913409038,14.7543525783653));
#23161=CARTESIAN_POINT('Ctrl Pts',(2.67752998692593,0.54530029314993,14.7926670500713));
#23162=CARTESIAN_POINT('Ctrl Pts',(2.70677127875774,0.287719996404971,14.8820622920458));
#23163=CARTESIAN_POINT('Ctrl Pts',(2.72591975017619,0.106490054773707,14.9076709254911));
#23164=CARTESIAN_POINT('Ctrl Pts',(2.75031354364582,-0.120195919936996,
14.8955788049496));
#23165=CARTESIAN_POINT('Ctrl Pts',(2.75522162089908,-0.165671790034989,
14.8909134542766));
#23166=CARTESIAN_POINT('Ctrl Pts',(2.77009054777941,-0.302795607010329,
14.8700245083829));
#23167=CARTESIAN_POINT('Ctrl Pts',(2.77999346651961,-0.393128585453869,
14.846886229962));
#23168=CARTESIAN_POINT('Ctrl Pts',(2.79970562545924,-0.565980620889559,
14.7837246427035));
#23169=CARTESIAN_POINT('Ctrl Pts',(2.80946709376518,-0.648213481481454,
14.7442274274943));
#23170=CARTESIAN_POINT('Ctrl Pts',(2.83857898677403,-0.880210390133891,
14.6035157318107));
#23171=CARTESIAN_POINT('Ctrl Pts',(2.85755216608694,-1.01488049741367,14.4810880890802));
#23172=CARTESIAN_POINT('Ctrl Pts',(2.88658123226053,-1.17626758116645,14.2644970249803));
#23173=CARTESIAN_POINT('Ctrl Pts',(2.89623374033106,-1.22286448705829,14.1875059788387));
#23174=CARTESIAN_POINT('Ctrl Pts',(2.91546261859488,-1.30070133902556,14.0255956353864));
#23175=CARTESIAN_POINT('Ctrl Pts',(2.92503074564317,-1.33174756560988,13.9410478719655));
#23176=CARTESIAN_POINT('Ctrl Pts',(2.9542902699067,-1.40088297110484,13.6766037982742));
#23177=CARTESIAN_POINT('Ctrl Pts',(2.97375228394956,-1.41194580410859,13.4916972316156));
#23178=CARTESIAN_POINT('Ctrl Pts',(3.0031538638659,-1.37477554337072,13.2204474743347));
#23179=CARTESIAN_POINT('Ctrl Pts',(3.01284518917861,-1.35388256235668,13.1323577884262));
#23180=CARTESIAN_POINT('Ctrl Pts',(3.03801192591717,-1.27754760755037,12.9091939938116));
#23181=CARTESIAN_POINT('Ctrl Pts',(3.05337881302878,-1.20926446619212,12.7796830412083));
#23182=CARTESIAN_POINT('Ctrl Pts',(3.07715259870693,-1.07705433667825,12.602407122906));
#23183=CARTESIAN_POINT('Ctrl Pts',(3.08530606893138,-1.0270062147963,12.5455488825751));
#23184=CARTESIAN_POINT('Ctrl Pts',(3.09756951055421,-0.94510461144696,12.4664430758878));
#23185=CARTESIAN_POINT('Ctrl Pts',(3.10168008047209,-0.916517926702076,
12.4410109684072));
#23186=CARTESIAN_POINT('Ctrl Pts',(3.10986378955223,-0.857326209600113,
12.392545637421));
#23187=CARTESIAN_POINT('Ctrl Pts',(3.11393406542358,-0.826747140816238,
12.3695343892349));
#23188=CARTESIAN_POINT('Ctrl Pts',(3.11803278688524,-0.79526461825914,12.3478046229284));
#23189=CARTESIAN_POINT('',(3.11803278688524,-7.6193401827091E-11,12.1));
#23190=CARTESIAN_POINT('Origin',(3.11803278688524,0.,13.5));
#23191=CARTESIAN_POINT('',(2.4462258455051,9.9958277766099E-11,12.1));
#23192=CARTESIAN_POINT('',(2.82743338823077,3.99408172289043E-15,12.1));
#23193=CARTESIAN_POINT('Ctrl Pts',(2.44622584550511,9.99578197991013E-11,
12.1));
#23194=CARTESIAN_POINT('Ctrl Pts',(2.43535738742254,-0.101588171354874,
12.0999999999927));
#23195=CARTESIAN_POINT('Ctrl Pts',(2.4245285855633,-0.202874837380493,12.1110572920391));
#23196=CARTESIAN_POINT('Ctrl Pts',(2.40940149924196,-0.340651325123096,
12.1415015994721));
#23197=CARTESIAN_POINT('Ctrl Pts',(2.40516687749463,-0.378827339870843,
12.1516503894212));
#23198=CARTESIAN_POINT('Ctrl Pts',(2.40093257836374,-0.416497469208933,
12.163388666013));
#23199=CARTESIAN_POINT('Origin',(0.,0.,13.5));
#23200=CARTESIAN_POINT('',(1.2784105384869,-0.416497393834651,12.1633886425258));
#23201=CARTESIAN_POINT('',(1.45844776950583,-0.416497492092897,12.1633886731438));
#23202=CARTESIAN_POINT('',(0.,-0.416497449530544,12.1633886598811));
#23203=CARTESIAN_POINT('Ctrl Pts',(1.27841053848688,-0.416497393834759,
12.1633886425259));
#23204=CARTESIAN_POINT('Ctrl Pts',(1.28527178782894,-0.35549476439837,12.1443797989789));
#23205=CARTESIAN_POINT('Ctrl Pts',(1.2921365525235,-0.293132247098585,12.1295287146373));
#23206=CARTESIAN_POINT('Ctrl Pts',(1.31508503284192,-0.0811815868699625,
12.0942553113078));
#23207=CARTESIAN_POINT('Ctrl Pts',(1.33101467229848,0.0704855897874028,
12.0936793574202));
#23208=CARTESIAN_POINT('Ctrl Pts',(1.35683082249829,0.307564317060159,12.131282019496));
#23209=CARTESIAN_POINT('Ctrl Pts',(1.36646427484744,0.394276150658717,12.153697192415));
#23210=CARTESIAN_POINT('Ctrl Pts',(1.38646947732948,0.569484258485247,12.217381876624));
#23211=CARTESIAN_POINT('Ctrl Pts',(1.39676539950078,0.657015788254973,12.2599384696789));
#23212=CARTESIAN_POINT('Ctrl Pts',(1.41693666553056,0.817140830789634,12.3595378026002));
#23213=CARTESIAN_POINT('Ctrl Pts',(1.42673342773507,0.889914770527173,12.4153690187576));
#23214=CARTESIAN_POINT('Ctrl Pts',(1.4561871961819,1.09044099002743,12.6030677246971));
#23215=CARTESIAN_POINT('Ctrl Pts',(1.47577090895044,1.19831474728728,12.7532764172855));
#23216=CARTESIAN_POINT('Ctrl Pts',(1.5047821378587,1.31110480527774,13.001063248523));
#23217=CARTESIAN_POINT('Ctrl Pts',(1.51422500293577,1.34018478089476,13.0854665168065));
#23218=CARTESIAN_POINT('Ctrl Pts',(1.53890976520056,1.39428227099436,13.3099853245802));
#23219=CARTESIAN_POINT('Ctrl Pts',(1.55417473125633,1.40635549640416,13.4521616967641));
#23220=CARTESIAN_POINT('Ctrl Pts',(1.58277681906667,1.38857272398384,13.7172532563586));
#23221=CARTESIAN_POINT('Ctrl Pts',(1.59588733586668,1.3639299051115,13.8391616710263));
#23222=CARTESIAN_POINT('Ctrl Pts',(1.61888907739522,1.29376233059279,14.0427221212447));
#23223=CARTESIAN_POINT('Ctrl Pts',(1.6286552621968,1.25554658577749,14.126075444644));
#23224=CARTESIAN_POINT('Ctrl Pts',(1.64824339761474,1.16347297778776,14.284011208513));
#23225=CARTESIAN_POINT('Ctrl Pts',(1.65803625950705,1.10985864349576,14.3582285694769));
#23226=CARTESIAN_POINT('Ctrl Pts',(1.68755347029578,0.927901482507346,14.5642796080963));
#23227=CARTESIAN_POINT('Ctrl Pts',(1.70686773435893,0.780522374477723,14.6766380391314));
#23228=CARTESIAN_POINT('Ctrl Pts',(1.73623813954844,0.534872879558241,14.7969210847266));
#23229=CARTESIAN_POINT('Ctrl Pts',(1.74590859244064,0.450449288583891,14.8286042597794));
#23230=CARTESIAN_POINT('Ctrl Pts',(1.76519305260318,0.27659512533074,14.8753569881007));
#23231=CARTESIAN_POINT('Ctrl Pts',(1.77479216187826,0.187565754538626,14.8902988283207));
#23232=CARTESIAN_POINT('Ctrl Pts',(1.79417060446524,0.0071422485920177,
14.9029232059173));
#23233=CARTESIAN_POINT('Ctrl Pts',(1.80390303357478,-0.0838383583836259,
14.9004341828375));
#23234=CARTESIAN_POINT('Ctrl Pts',(1.82328449409847,-0.263534104947346,
14.8779345155732));
#23235=CARTESIAN_POINT('Ctrl Pts',(1.83290954613354,-0.351836618136786,
14.8580738231442));
#23236=CARTESIAN_POINT('Ctrl Pts',(1.85231855018614,-0.523817649789653,
14.8014806159072));
#23237=CARTESIAN_POINT('Ctrl Pts',(1.86205654006245,-0.607064073991918,
14.7647964320767));
#23238=CARTESIAN_POINT('Ctrl Pts',(1.88150900832868,-0.76529633500339,14.6758237571641));
#23239=CARTESIAN_POINT('Ctrl Pts',(1.89119673559068,-0.839905901416373,
14.6237429072962));
#23240=CARTESIAN_POINT('Ctrl Pts',(1.91071720391687,-0.978460482517055,
14.505469172187));
#23241=CARTESIAN_POINT('Ctrl Pts',(1.92048812916967,-1.04199674537574,14.4394658315659));
#23242=CARTESIAN_POINT('Ctrl Pts',(1.94994329715363,-1.21245600572361,14.2236480957466));
#23243=CARTESIAN_POINT('Ctrl Pts',(1.96951967562116,-1.29681486411763,14.058558569738));
#23244=CARTESIAN_POINT('Ctrl Pts',(2.00441118245624,-1.38579273892104,13.7447485931775));
#23245=CARTESIAN_POINT('Ctrl Pts',(2.01950536501099,-1.40350427074367,13.6024594297712));
#23246=CARTESIAN_POINT('Ctrl Pts',(2.0444644722023,-1.39685941518724,13.3702059476167));
#23247=CARTESIAN_POINT('Ctrl Pts',(2.05412297400445,-1.38566229137934,13.2809033073099));
#23248=CARTESIAN_POINT('Ctrl Pts',(2.07236012816617,-1.34835985142555,13.114770747565));
#23249=CARTESIAN_POINT('Ctrl Pts',(2.08093204423063,-1.32399268173303,13.0379183062463));
#23250=CARTESIAN_POINT('Ctrl Pts',(2.09930330238021,-1.25818800648483,12.8792800237421));
#23251=CARTESIAN_POINT('Ctrl Pts',(2.10907328381213,-1.21505694275106,12.7985966563273));
#23252=CARTESIAN_POINT('Ctrl Pts',(2.12849960866751,-1.11435028434478,12.6477420840303));
#23253=CARTESIAN_POINT('Ctrl Pts',(2.13810698755743,-1.0571992888945,12.5778017232459));
#23254=CARTESIAN_POINT('Ctrl Pts',(2.15750276471468,-0.929763103826513,
12.4493878627635));
#23255=CARTESIAN_POINT('Ctrl Pts',(2.16724806963363,-0.859682219986245,
12.3913108074149));
#23256=CARTESIAN_POINT('Ctrl Pts',(2.19165096222075,-0.67107647846954,12.2637150953956));
#23257=CARTESIAN_POINT('Ctrl Pts',(2.20615776602033,-0.54708858513539,12.2040817707949));
#23258=CARTESIAN_POINT('Ctrl Pts',(2.22083974265588,-0.416497439768571,
12.1633886568392));
#23259=CARTESIAN_POINT('Ctrl Pts',(2.40093257836374,-0.416497469208933,
12.163388666013));
#23260=CARTESIAN_POINT('Ctrl Pts',(2.3942679260537,-0.475789056022099,12.1818643404481));
#23261=CARTESIAN_POINT('Ctrl Pts',(2.3876098108882,-0.533827934293694,12.2042780440777));
#23262=CARTESIAN_POINT('Ctrl Pts',(2.36685390738263,-0.709184394622676,
12.285805323635));
#23263=CARTESIAN_POINT('Ctrl Pts',(2.3527720126406,-0.819788955100745,12.3575640409707));
#23264=CARTESIAN_POINT('Ctrl Pts',(2.32196013711664,-1.03777754350177,12.5471676522693));
#23265=CARTESIAN_POINT('Ctrl Pts',(2.30536793090488,-1.13842662625283,12.6700281321853));
#23266=CARTESIAN_POINT('Ctrl Pts',(2.27942573841901,-1.25778282043891,12.8795602954755));
#23267=CARTESIAN_POINT('Ctrl Pts',(2.27041266920003,-1.29251910490724,12.9556133187173));
#23268=CARTESIAN_POINT('Ctrl Pts',(2.25165158192398,-1.35037421679487,13.1196356318881));
#23269=CARTESIAN_POINT('Ctrl Pts',(2.24199800499422,-1.3721307398421,13.2076879561223));
#23270=CARTESIAN_POINT('Ctrl Pts',(2.21274112166428,-1.41179852640499,13.4786777448907));
#23271=CARTESIAN_POINT('Ctrl Pts',(2.19331161153257,-1.40245000186556,13.6635882072515));
#23272=CARTESIAN_POINT('Ctrl Pts',(2.16398044318386,-1.33570747042758,13.9289974853134));
#23273=CARTESIAN_POINT('Ctrl Pts',(2.15429101166608,-1.30526626220759,14.014230366182));
#23274=CARTESIAN_POINT('Ctrl Pts',(2.13492457891323,-1.22848069206958,14.1774602022811));
#23275=CARTESIAN_POINT('Ctrl Pts',(2.12533659082138,-1.18234924039453,14.2550948763787));
#23276=CARTESIAN_POINT('Ctrl Pts',(2.09659716247621,-1.02317339201938,14.4722133868433));
#23277=CARTESIAN_POINT('Ctrl Pts',(2.07743672410967,-0.890526978712175,
14.5950077189689));
#23278=CARTESIAN_POINT('Ctrl Pts',(2.05337558622913,-0.699595503347848,
14.7135266609751));
#23279=CARTESIAN_POINT('Ctrl Pts',(2.04850445727977,-0.659686081635776,
14.73567600164));
#23280=CARTESIAN_POINT('Ctrl Pts',(2.02397082167762,-0.453799667660683,
14.8371187382518));
#23281=CARTESIAN_POINT('Ctrl Pts',(2.00437023026017,-0.274422283731444,
14.8851040943022));
#23282=CARTESIAN_POINT('Ctrl Pts',(1.97493918266089,0.000437004015423861,
14.9029891737956));
#23283=CARTESIAN_POINT('Ctrl Pts',(1.96517813060858,0.0921405430985885,
14.8999600698876));
#23284=CARTESIAN_POINT('Ctrl Pts',(1.94558496699582,0.273177956461229,14.8761059608175));
#23285=CARTESIAN_POINT('Ctrl Pts',(1.93580459714485,0.362093112473848,14.8554271781499));
#23286=CARTESIAN_POINT('Ctrl Pts',(1.91627695806057,0.534844137746019,14.7970251990701));
#23287=CARTESIAN_POINT('Ctrl Pts',(1.90654738375972,0.618252854745831,14.7594030249013));
#23288=CARTESIAN_POINT('Ctrl Pts',(1.88698003020699,0.776588871269993,14.6684389306091));
#23289=CARTESIAN_POINT('Ctrl Pts',(1.87719230806854,0.851134107596775,14.615307554439));
#23290=CARTESIAN_POINT('Ctrl Pts',(1.86255386709511,0.95430049655303,14.5253704040316));
#23291=CARTESIAN_POINT('Ctrl Pts',(1.85769220445115,0.987147379380306,14.4937876919291));
#23292=CARTESIAN_POINT('Ctrl Pts',(1.83342093916487,1.14292514580336,14.3286476146511));
#23293=CARTESIAN_POINT('Ctrl Pts',(1.81405632478123,1.24060384114422,14.1736732899444));
#23294=CARTESIAN_POINT('Ctrl Pts',(1.78485771682689,1.33886019962667,13.9192612648863));
#23295=CARTESIAN_POINT('Ctrl Pts',(1.77513100297321,1.36333430114081,13.8311285134366));
#23296=CARTESIAN_POINT('Ctrl Pts',(1.75555071726262,1.39481470298217,13.6511723335134));
#23297=CARTESIAN_POINT('Ctrl Pts',(1.74575167681533,1.40170907790057,13.5597733543252));
#23298=CARTESIAN_POINT('Ctrl Pts',(1.72615648732792,1.39757523499232,13.3769231235782));
#23299=CARTESIAN_POINT('Ctrl Pts',(1.71638039675177,1.38655345072885,13.2859112806918));
#23300=CARTESIAN_POINT('Ctrl Pts',(1.69690518488617,1.34716398179204,13.1084565694359));
#23301=CARTESIAN_POINT('Ctrl Pts',(1.68724354472194,1.31910639494897,13.0223857576645));
#23302=CARTESIAN_POINT('Ctrl Pts',(1.67269223440346,1.26470051115681,12.8978268208691));
#23303=CARTESIAN_POINT('Ctrl Pts',(1.66782223879557,1.24441422456665,12.8569500556959));
#23304=CARTESIAN_POINT('Ctrl Pts',(1.64637722897859,1.1465645019785,12.6818215784041));
#23305=CARTESIAN_POINT('Ctrl Pts',(1.62980792907299,1.04901018847223,12.5599989844274));
#23306=CARTESIAN_POINT('Ctrl Pts',(1.60831216041011,0.899479242881735,12.4262119475076));
#23307=CARTESIAN_POINT('Ctrl Pts',(1.6034369151753,0.86399168139286,12.3974564960722));
#23308=CARTESIAN_POINT('Ctrl Pts',(1.58124002742741,0.696442070404857,12.2747570532381));
#23309=CARTESIAN_POINT('Ctrl Pts',(1.56393722882228,0.550091032214942,12.2024446972363));
#23310=CARTESIAN_POINT('Ctrl Pts',(1.54168997577148,0.350850647229146,12.1439073992733));
#23311=CARTESIAN_POINT('Ctrl Pts',(1.53681457014148,0.306454612382846,12.1331902129952));
#23312=CARTESIAN_POINT('Ctrl Pts',(1.51462781442213,0.10256795488322,12.0944073277006));
#23313=CARTESIAN_POINT('Ctrl Pts',(1.49733357660129,-0.0605264833183406,
12.0919708883101));
#23314=CARTESIAN_POINT('Ctrl Pts',(1.47511125510869,-0.265463597988811,
12.1246413840912));
#23315=CARTESIAN_POINT('Ctrl Pts',(1.47023957074921,-0.31014865132287,12.1340240986041));
#23316=CARTESIAN_POINT('Ctrl Pts',(1.46305678534565,-0.375181790474972,
12.1510356975939));
#23317=CARTESIAN_POINT('Ctrl Pts',(1.46075201473401,-0.395920905392733,
12.1569768639781));
#23318=CARTESIAN_POINT('Ctrl Pts',(1.45844776950582,-0.416497492092995,
12.1633886731438));
#23319=CARTESIAN_POINT('Origin',(0.,0.,13.5));
#23320=CARTESIAN_POINT('',(0.335948685957609,-0.416497449525761,12.1633886598796));
#23321=CARTESIAN_POINT('',(0.51591329100944,-0.416497503173569,12.1633886765966));
#23322=CARTESIAN_POINT('',(0.,-0.416497449530544,12.1633886598811));
#23323=CARTESIAN_POINT('Ctrl Pts',(0.33594868595761,-0.41649744952576,12.1633886598796));
#23324=CARTESIAN_POINT('Ctrl Pts',(0.338092137022063,-0.397430723115034,
12.1574473344676));
#23325=CARTESIAN_POINT('Ctrl Pts',(0.340232102393261,-0.378231240764015,
12.1519122386787));
#23326=CARTESIAN_POINT('Ctrl Pts',(0.355812558107325,-0.237457708666163,
12.1145748990151));
#23327=CARTESIAN_POINT('Ctrl Pts',(0.369115667260259,-0.112219229772241,
12.0988592976413));
#23328=CARTESIAN_POINT('Ctrl Pts',(0.392254665094067,0.103470382396172,
12.1009280078));
#23329=CARTESIAN_POINT('Ctrl Pts',(0.401944321812012,0.19321951081267,12.1104769948009));
#23330=CARTESIAN_POINT('Ctrl Pts',(0.429305497035372,0.442459199927157,
12.1616227618598));
#23331=CARTESIAN_POINT('Ctrl Pts',(0.446618745266285,0.596421336295759,
12.222773843572));
#23332=CARTESIAN_POINT('Ctrl Pts',(0.473903955602125,0.812774735809414,
12.3565435122433));
#23333=CARTESIAN_POINT('Ctrl Pts',(0.483577366325789,0.884563388325348,
12.4111276384374));
#23334=CARTESIAN_POINT('Ctrl Pts',(0.499640090606945,0.994534335407759,
12.5128422998071));
#23335=CARTESIAN_POINT('Ctrl Pts',(0.506017782138323,1.03580385112511,12.5562365973114));
#23336=CARTESIAN_POINT('Ctrl Pts',(0.53199673668229,1.19139469283705,12.7423800946747));
#23337=CARTESIAN_POINT('Ctrl Pts',(0.551404636661235,1.28002686676363,12.9042313657085));
#23338=CARTESIAN_POINT('Ctrl Pts',(0.575879097201786,1.34880308277725,13.1220893768416));
#23339=CARTESIAN_POINT('Ctrl Pts',(0.580766698942489,1.36041365575882,13.1662922129466));
#23340=CARTESIAN_POINT('Ctrl Pts',(0.590553404302888,1.37927566207682,13.2556918339382));
#23341=CARTESIAN_POINT('Ctrl Pts',(0.595446882381403,1.38651405868556,13.3008352938842));
#23342=CARTESIAN_POINT('Ctrl Pts',(0.60523878008134,1.39655005696943,13.3916681562918));
#23343=CARTESIAN_POINT('Ctrl Pts',(0.610129967868918,1.39934162048136,13.4373032431323));
#23344=CARTESIAN_POINT('Ctrl Pts',(0.619920599759535,1.40045172493147,13.5286787763786));
#23345=CARTESIAN_POINT('Ctrl Pts',(0.624814422836377,1.39876997354232,13.5743644686515));
#23346=CARTESIAN_POINT('Ctrl Pts',(0.639475059197237,1.38705003220774,13.7107244634538));
#23347=CARTESIAN_POINT('Ctrl Pts',(0.649206048549967,1.37038764506943,13.8005830608694));
#23348=CARTESIAN_POINT('Ctrl Pts',(0.663871512140508,1.33245393080345,13.9320292970078));
#23349=CARTESIAN_POINT('Ctrl Pts',(0.668763870510218,1.31766337636763,13.9752326059005));
#23350=CARTESIAN_POINT('Ctrl Pts',(0.683389203926127,1.26720104388982,14.1020414657331));
#23351=CARTESIAN_POINT('Ctrl Pts',(0.693084241148559,1.22547720712379,14.182977295026));
#23352=CARTESIAN_POINT('Ctrl Pts',(0.707714908290906,1.15145876403461,14.2976371985038));
#23353=CARTESIAN_POINT('Ctrl Pts',(0.712607191073157,1.12484960903662,14.3347429304424));
#23354=CARTESIAN_POINT('Ctrl Pts',(0.727225623704985,1.04002533502238,14.4415891269759));
#23355=CARTESIAN_POINT('Ctrl Pts',(0.736899857886182,0.97679134081702,14.5070360362464));
#23356=CARTESIAN_POINT('Ctrl Pts',(0.756396983623417,0.838164987882815,
14.6250835129975));
#23357=CARTESIAN_POINT('Ctrl Pts',(0.766173387598592,0.763040411002447,
14.6773285986624));
#23358=CARTESIAN_POINT('Ctrl Pts',(0.795621374482452,0.523215582157543,
14.8114558805551));
#23359=CARTESIAN_POINT('Ctrl Pts',(0.815191282547029,0.347000479778492,
14.8686730293357));
#23360=CARTESIAN_POINT('Ctrl Pts',(0.844409565680878,0.0748791223030258,
14.9009234741048));
#23361=CARTESIAN_POINT('Ctrl Pts',(0.854031190077165,-0.0158285778211942,
14.9028335972271));
#23362=CARTESIAN_POINT('Ctrl Pts',(0.872199699440062,-0.184895990780581,
14.8899859897267));
#23363=CARTESIAN_POINT('Ctrl Pts',(0.880694956781953,-0.263059204620027,
14.8773331552573));
#23364=CARTESIAN_POINT('Ctrl Pts',(0.908999943449859,-0.517933496143129,
14.8135780149835));
#23365=CARTESIAN_POINT('Ctrl Pts',(0.92842488150862,-0.685636395733855,
14.7343618976148));
#23366=CARTESIAN_POINT('Ctrl Pts',(0.957892544291619,-0.906734517687264,
14.5706040444889));
#23367=CARTESIAN_POINT('Ctrl Pts',(0.967663928233954,-0.97470328053528,
14.5091154198522));
#23368=CARTESIAN_POINT('Ctrl Pts',(0.987261220477669,-1.09768780537988,
14.3737534516641));
#23369=CARTESIAN_POINT('Ctrl Pts',(0.997027096616553,-1.15240592287781,
14.3002026136494));
#23370=CARTESIAN_POINT('Ctrl Pts',(1.01662000331737,-1.2466914968752,14.1435188180007));
#23371=CARTESIAN_POINT('Ctrl Pts',(1.02639719284007,-1.28603939852387,14.0607662365323));
#23372=CARTESIAN_POINT('Ctrl Pts',(1.04598492052491,-1.34802389003489,13.888818195646));
#23373=CARTESIAN_POINT('Ctrl Pts',(1.0557199396963,-1.37052024212579,13.8000374920693));
#23374=CARTESIAN_POINT('Ctrl Pts',(1.07038622751275,-1.39104982008156,13.6645238239822));
#23375=CARTESIAN_POINT('Ctrl Pts',(1.07527834582645,-1.39567792843094,13.619040724484));
#23376=CARTESIAN_POINT('Ctrl Pts',(1.08989561361535,-1.40282341212471,13.4829635874722));
#23377=CARTESIAN_POINT('Ctrl Pts',(1.09961197157324,-1.39878420382174,13.3922647135418));
#23378=CARTESIAN_POINT('Ctrl Pts',(1.11418923719126,-1.37958955273921,13.2574973538008));
#23379=CARTESIAN_POINT('Ctrl Pts',(1.11906060732706,-1.37096964926112,13.2127421404134));
#23380=CARTESIAN_POINT('Ctrl Pts',(1.13369038436817,-1.33862874088626,13.0800487859611));
#23381=CARTESIAN_POINT('Ctrl Pts',(1.14343021921865,-1.30849982164006,12.9939225852327));
#23382=CARTESIAN_POINT('Ctrl Pts',(1.16287424891295,-1.23209947466277,12.8290662240178));
#23383=CARTESIAN_POINT('Ctrl Pts',(1.17254497351587,-1.18607288397003,12.7506989625543));
#23384=CARTESIAN_POINT('Ctrl Pts',(1.1919948476445,-1.07948530677624,12.6039299282727));
#23385=CARTESIAN_POINT('Ctrl Pts',(1.201720950175,-1.01916717323023,12.5358793063566));
#23386=CARTESIAN_POINT('Ctrl Pts',(1.22114976917045,-0.886187310618468,
12.4123837972148));
#23387=CARTESIAN_POINT('Ctrl Pts',(1.23083383566112,-0.813836349809595,
12.3572370346479));
#23388=CARTESIAN_POINT('Ctrl Pts',(1.25320840746357,-0.636295706514283,
12.2473798016744));
#23389=CARTESIAN_POINT('Ctrl Pts',(1.26579107429575,-0.528695691748085,
12.1983504123869));
#23390=CARTESIAN_POINT('Ctrl Pts',(1.27841053848688,-0.41649739383476,12.1633886425259));
#23391=CARTESIAN_POINT('Ctrl Pts',(1.45844776950582,-0.416497492092994,
12.1633886731438));
#23392=CARTESIAN_POINT('Ctrl Pts',(1.44390140370835,-0.546394498428389,
12.2038654941029));
#23393=CARTESIAN_POINT('Ctrl Pts',(1.42932090092249,-0.66980860421863,12.2630972886968));
#23394=CARTESIAN_POINT('Ctrl Pts',(1.40497113230301,-0.858142498666153,
12.3901120941702));
#23395=CARTESIAN_POINT('Ctrl Pts',(1.39529191720086,-0.928364884453008,
12.4481451379525));
#23396=CARTESIAN_POINT('Ctrl Pts',(1.37589278928849,-1.0561522778362,12.5765847592017));
#23397=CARTESIAN_POINT('Ctrl Pts',(1.36621708162912,-1.11349612870909,12.6466070920168));
#23398=CARTESIAN_POINT('Ctrl Pts',(1.35165264523808,-1.18905132560126,12.7595697679454));
#23399=CARTESIAN_POINT('Ctrl Pts',(1.34677567923691,-1.21253937447488,12.7986952875696));
#23400=CARTESIAN_POINT('Ctrl Pts',(1.3266664764074,-1.30123595698637,12.9642646260475));
#23401=CARTESIAN_POINT('Ctrl Pts',(1.31143822683817,-1.34890190962999,13.099137562112));
#23402=CARTESIAN_POINT('Ctrl Pts',(1.29132750458486,-1.38394639101076,13.2837200195658));
#23403=CARTESIAN_POINT('Ctrl Pts',(1.28645640659027,-1.39026346900012,13.3289670970169));
#23404=CARTESIAN_POINT('Ctrl Pts',(1.26164462562856,-1.41110536175855,13.5604230724584));
#23405=CARTESIAN_POINT('Ctrl Pts',(1.24171274821886,-1.39047412541093,13.7478856871491));
#23406=CARTESIAN_POINT('Ctrl Pts',(1.21196375405839,-1.30604124250456,14.0123677418593));
#23407=CARTESIAN_POINT('Ctrl Pts',(1.20229122750465,-1.27002421989132,14.0960732585933));
#23408=CARTESIAN_POINT('Ctrl Pts',(1.18279514596295,-1.18206371535408,14.2556903818919));
#23409=CARTESIAN_POINT('Ctrl Pts',(1.17302428235503,-1.13025820137227,14.3311790212574));
#23410=CARTESIAN_POINT('Ctrl Pts',(1.15343684225622,-1.01265757072314,14.4710174152128));
#23411=CARTESIAN_POINT('Ctrl Pts',(1.14367565859755,-0.947136867220968,
14.5350275439779));
#23412=CARTESIAN_POINT('Ctrl Pts',(1.12414012684928,-0.804903306426751,
14.6490867902023));
#23413=CARTESIAN_POINT('Ctrl Pts',(1.11440175457461,-0.72858366905622,14.6989311100021));
#23414=CARTESIAN_POINT('Ctrl Pts',(1.09491224012219,-0.567171507992726,
14.7832088066028));
#23415=CARTESIAN_POINT('Ctrl Pts',(1.08520084686711,-0.48244522490888,14.8174045751253));
#23416=CARTESIAN_POINT('Ctrl Pts',(1.06576506079662,-0.308447106548023,
14.8685757280464));
#23417=CARTESIAN_POINT('Ctrl Pts',(1.05608578405447,-0.219637104216404,
14.88560406286));
#23418=CARTESIAN_POINT('Ctrl Pts',(1.04152804715565,-0.084374639456373,
14.8981999478329));
#23419=CARTESIAN_POINT('Ctrl Pts',(1.03665029630423,-0.0387602206887427,
14.9002070899748));
#23420=CARTESIAN_POINT('Ctrl Pts',(1.02199519541023,0.0982033775170876,
14.8995348936809));
#23421=CARTESIAN_POINT('Ctrl Pts',(1.01222986789598,0.189271681394011,14.8901501746134));
#23422=CARTESIAN_POINT('Ctrl Pts',(0.982826771131795,0.457798104227207,
14.8355875198765));
#23423=CARTESIAN_POINT('Ctrl Pts',(0.963568332078361,0.627983659964473,
14.7645194167979));
#23424=CARTESIAN_POINT('Ctrl Pts',(0.939048234817051,0.817635902210224,
14.637346262212));
#23425=CARTESIAN_POINT('Ctrl Pts',(0.934139659251513,0.854293238047118,
14.610075661621));
#23426=CARTESIAN_POINT('Ctrl Pts',(0.909573582717069,1.0306746403647,14.4649403458635));
#23427=CARTESIAN_POINT('Ctrl Pts',(0.890268741296078,1.14770538454531,14.3222983994732));
#23428=CARTESIAN_POINT('Ctrl Pts',(0.860853984559888,1.27727792581275,14.0804734489303));
#23429=CARTESIAN_POINT('Ctrl Pts',(0.851063086401508,1.31250714136801,13.9956944862125));
#23430=CARTESIAN_POINT('Ctrl Pts',(0.831247961053441,1.36628502388815,13.8192130425103));
#23431=CARTESIAN_POINT('Ctrl Pts',(0.821260870522121,1.38445311748892,13.7278637351812));
#23432=CARTESIAN_POINT('Ctrl Pts',(0.791622230502018,1.41124680096498,13.4521001652212));
#23433=CARTESIAN_POINT('Ctrl Pts',(0.772309782213003,1.3927180268365,13.2670917214919));
#23434=CARTESIAN_POINT('Ctrl Pts',(0.747567348924004,1.32559012452433,13.0473499858023));
#23435=CARTESIAN_POINT('Ctrl Pts',(0.742646789672397,1.31013735305008,13.0043981120919));
#23436=CARTESIAN_POINT('Ctrl Pts',(0.718228233628566,1.22321168507718,12.7954398106915));
#23437=CARTESIAN_POINT('Ctrl Pts',(0.699178436344836,1.12215614097056,12.643598446638));
#23438=CARTESIAN_POINT('Ctrl Pts',(0.670085606053116,0.930779510263475,
12.4502420779579));
#23439=CARTESIAN_POINT('Ctrl Pts',(0.660337607383824,0.860331074096645,
12.3917707444403));
#23440=CARTESIAN_POINT('Ctrl Pts',(0.637622694486556,0.684965571709589,
12.2730837732651));
#23441=CARTESIAN_POINT('Ctrl Pts',(0.624671890713921,0.576943551247466,
12.2187355726817));
#23442=CARTESIAN_POINT('Ctrl Pts',(0.602204515054362,0.378628769124433,
12.1491884842473));
#23443=CARTESIAN_POINT('Ctrl Pts',(0.592687701417284,0.291294760816019,
12.1277029502485));
#23444=CARTESIAN_POINT('Ctrl Pts',(0.563970789415144,0.025163055150938,
12.0887985245306));
#23445=CARTESIAN_POINT('Ctrl Pts',(0.544733641290613,-0.155515562515679,
12.0971688025917));
#23446=CARTESIAN_POINT('Ctrl Pts',(0.52232947888016,-0.358895607883152,
12.1464503794261));
#23447=CARTESIAN_POINT('Ctrl Pts',(0.519120376922039,-0.387843916658138,
12.1544600172087));
#23448=CARTESIAN_POINT('Ctrl Pts',(0.515913291009439,-0.416497503173569,
12.1633886765966));
#23449=CARTESIAN_POINT('Origin',(0.,0.,13.5));
#23450=CARTESIAN_POINT('',(-0.606544106580495,-0.416497449298501,12.1633886598088));
#23451=CARTESIAN_POINT('',(-0.426566464895915,-0.416497451671886,12.1633886605483));
#23452=CARTESIAN_POINT('',(0.,-0.416497449530544,12.1633886598811));
#23453=CARTESIAN_POINT('Ctrl Pts',(-0.606544106580495,-0.416497449298501,
12.1633886598088));
#23454=CARTESIAN_POINT('Ctrl Pts',(-0.601905488457186,-0.375006509663048,
12.1504597925999));
#23455=CARTESIAN_POINT('Ctrl Pts',(-0.597278269205687,-0.33293461748609,
12.1394694228009));
#23456=CARTESIAN_POINT('Ctrl Pts',(-0.582914697219095,-0.201117435002572,
12.1115170003321));
#23457=CARTESIAN_POINT('Ctrl Pts',(-0.57318643731515,-0.110182143195263,
12.1013607375965));
#23458=CARTESIAN_POINT('Ctrl Pts',(-0.553446929682907,0.0735757584082064,
12.0988782990464));
#23459=CARTESIAN_POINT('Ctrl Pts',(-0.54348018098935,0.165959238117452,
12.106797694933));
#23460=CARTESIAN_POINT('Ctrl Pts',(-0.523806474452879,0.345932180485655,
12.140390867513));
#23461=CARTESIAN_POINT('Ctrl Pts',(-0.514163696021878,0.433160474790576,
12.1656166336715));
#23462=CARTESIAN_POINT('Ctrl Pts',(-0.494700198953667,0.602343600699843,
12.2328968501379));
#23463=CARTESIAN_POINT('Ctrl Pts',(-0.484926277070032,0.68382862997349,
12.274950451567));
#23464=CARTESIAN_POINT('Ctrl Pts',(-0.470256490022007,0.798912786317021,
12.3494270619555));
#23465=CARTESIAN_POINT('Ctrl Pts',(-0.465378379653816,0.835965197363722,
12.3760596745377));
#23466=CARTESIAN_POINT('Ctrl Pts',(-0.450806540735884,0.94238070263997,
12.4607271465437));
#23467=CARTESIAN_POINT('Ctrl Pts',(-0.441114127584034,1.00749393308657,
12.523718727768));
#23468=CARTESIAN_POINT('Ctrl Pts',(-0.421637519360729,1.12516184376022,
12.6619549708284));
#23469=CARTESIAN_POINT('Ctrl Pts',(-0.411917585888672,1.17732541969383,
12.7369706621761));
#23470=CARTESIAN_POINT('Ctrl Pts',(-0.397263403204919,1.24410900676983,
12.8563571984881));
#23471=CARTESIAN_POINT('Ctrl Pts',(-0.392372898074839,1.26443035750525,
12.8972570085663));
#23472=CARTESIAN_POINT('Ctrl Pts',(-0.377693102703635,1.31929797812323,
13.0227279275616));
#23473=CARTESIAN_POINT('Ctrl Pts',(-0.367948862541147,1.34760789891663,
13.1097580647508));
#23474=CARTESIAN_POINT('Ctrl Pts',(-0.353273452437169,1.37705457699646,
13.2434802862271));
#23475=CARTESIAN_POINT('Ctrl Pts',(-0.348382685477986,1.38468248994158,
13.2884910085762));
#23476=CARTESIAN_POINT('Ctrl Pts',(-0.338592869039751,1.39552242749479,
13.3791528265224));
#23477=CARTESIAN_POINT('Ctrl Pts',(-0.333702520235257,1.3987224381974,13.4247506469136));
#23478=CARTESIAN_POINT('Ctrl Pts',(-0.31901389140055,1.4016192986816,13.5618417327739));
#23479=CARTESIAN_POINT('Ctrl Pts',(-0.309236318680863,1.39459013493301,
13.6532297388385));
#23480=CARTESIAN_POINT('Ctrl Pts',(-0.294543086364255,1.37076269807332,
13.7882646719869));
#23481=CARTESIAN_POINT('Ctrl Pts',(-0.289652656692205,1.36062728265345,
13.8328367382274));
#23482=CARTESIAN_POINT('Ctrl Pts',(-0.274958173542438,1.32371463845123,
13.9649122781796));
#23483=CARTESIAN_POINT('Ctrl Pts',(-0.265177775503078,1.29052677984863,
14.0503676019019));
#23484=CARTESIAN_POINT('Ctrl Pts',(-0.250484024407631,1.22862612997252,
14.172728679251));
#23485=CARTESIAN_POINT('Ctrl Pts',(-0.245591449054255,1.20602678094004,
14.2124503065406));
#23486=CARTESIAN_POINT('Ctrl Pts',(-0.235809207093606,1.15706239937249,
14.2894849551875));
#23487=CARTESIAN_POINT('Ctrl Pts',(-0.230928306990082,1.13073216643731,
14.326755504826));
#23488=CARTESIAN_POINT('Ctrl Pts',(-0.216285894299332,1.04652533933224,
14.4343847291161));
#23489=CARTESIAN_POINT('Ctrl Pts',(-0.206512619347025,0.983557927149029,
14.5004521250684));
#23490=CARTESIAN_POINT('Ctrl Pts',(-0.187095300662516,0.846029882079955,
14.6191253457583));
#23491=CARTESIAN_POINT('Ctrl Pts',(-0.177461575585183,0.771854941797795,
14.6715151752137));
#23492=CARTESIAN_POINT('Ctrl Pts',(-0.1523894013015,0.568451047806307,14.7874236212691));
#23493=CARTESIAN_POINT('Ctrl Pts',(-0.136960075163453,0.433573633496984,
14.8388842178022));
#23494=CARTESIAN_POINT('Ctrl Pts',(-0.112009582165764,0.205348834270106,
14.8877720473929));
#23495=CARTESIAN_POINT('Ctrl Pts',(-0.10246771960711,0.115847909542865,
14.8980911195459));
#23496=CARTESIAN_POINT('Ctrl Pts',(-0.0790818126658175,-0.102882316765015,
14.9021503972281));
#23497=CARTESIAN_POINT('Ctrl Pts',(-0.0652493200739028,-0.231453906580911,
14.8867361917234));
#23498=CARTESIAN_POINT('Ctrl Pts',(-0.0418508851995083,-0.442188056310697,
14.8313135019221));
#23499=CARTESIAN_POINT('Ctrl Pts',(-0.0323988608236905,-0.525933210372259,
14.8005080645975));
#23500=CARTESIAN_POINT('Ctrl Pts',(-0.0037040324834651,-0.768649969783498,
14.6839177890224));
#23501=CARTESIAN_POINT('Ctrl Pts',(0.0155776225967351,-0.914514945141154,
14.5752380582826));
#23502=CARTESIAN_POINT('Ctrl Pts',(0.0446595079971736,-1.0962344430835,
14.3754142026245));
#23503=CARTESIAN_POINT('Ctrl Pts',(0.0542063633042762,-1.15016838717273,
14.303240073177));
#23504=CARTESIAN_POINT('Ctrl Pts',(0.0758893164280386,-1.2560581069539,
14.1287738615946));
#23505=CARTESIAN_POINT('Ctrl Pts',(0.0879925333356952,-1.30313504295692,
14.0242845872087));
#23506=CARTESIAN_POINT('Ctrl Pts',(0.112234309053797,-1.36998634282861,
13.8090405622336));
#23507=CARTESIAN_POINT('Ctrl Pts',(0.124280390147709,-1.39019951632661,
13.699279640849));
#23508=CARTESIAN_POINT('Ctrl Pts',(0.145772293821565,-1.40275690694015,
13.5005638594427));
#23509=CARTESIAN_POINT('Ctrl Pts',(0.15512101706407,-1.40002642418665,13.4125026890467));
#23510=CARTESIAN_POINT('Ctrl Pts',(0.172561160499419,-1.37950805013817,
13.2493865276265));
#23511=CARTESIAN_POINT('Ctrl Pts',(0.180645864754135,-1.3637604292113,13.174413425371));
#23512=CARTESIAN_POINT('Ctrl Pts',(0.201537058586901,-1.30786707793749,
12.9863765421109));
#23513=CARTESIAN_POINT('Ctrl Pts',(0.214368119941527,-1.25919610294344,
12.8765055454839));
#23514=CARTESIAN_POINT('Ctrl Pts',(0.237031423027273,-1.15055531918141,
12.6973159661113));
#23515=CARTESIAN_POINT('Ctrl Pts',(0.246734793056764,-1.09665714528703,
12.6251142358414));
#23516=CARTESIAN_POINT('Ctrl Pts',(0.275519091084943,-0.915499506244006,
12.42571825934));
#23517=CARTESIAN_POINT('Ctrl Pts',(0.294374707439548,-0.770366427214801,
12.3173108041002));
#23518=CARTESIAN_POINT('Ctrl Pts',(0.32111414060799,-0.546585086849063,
12.2092611808737));
#23519=CARTESIAN_POINT('Ctrl Pts',(0.328547651546869,-0.482332168407897,
12.18390321911));
#23520=CARTESIAN_POINT('Ctrl Pts',(0.335948685957608,-0.416497449525761,
12.1633886598796));
#23521=CARTESIAN_POINT('Ctrl Pts',(0.515913291009439,-0.41649750317357,
12.1633886765966));
#23522=CARTESIAN_POINT('Ctrl Pts',(0.509385662631614,-0.474818349437701,
12.1815618630919));
#23523=CARTESIAN_POINT('Ctrl Pts',(0.502864638142664,-0.531918062096211,
12.203542253374));
#23524=CARTESIAN_POINT('Ctrl Pts',(0.476756448285556,-0.753481412729099,
12.3059597836098));
#23525=CARTESIAN_POINT('Ctrl Pts',(0.457267808032133,-0.902892290928627,
12.4145270387944));
#23526=CARTESIAN_POINT('Ctrl Pts',(0.427915708355189,-1.08929367372358,
12.6158094276354));
#23527=CARTESIAN_POINT('Ctrl Pts',(0.418168647906485,-1.14467899180946,
12.688788970831));
#23528=CARTESIAN_POINT('Ctrl Pts',(0.403475540394033,-1.21646022311045,
12.8055166231118));
#23529=CARTESIAN_POINT('Ctrl Pts',(0.398579668370075,-1.23845035331473,
12.8455358563514));
#23530=CARTESIAN_POINT('Ctrl Pts',(0.373982865261525,-1.33888291910941,
13.051568108984));
#23531=CARTESIAN_POINT('Ctrl Pts',(0.354487604621236,-1.38608585555331,
13.2308029737511));
#23532=CARTESIAN_POINT('Ctrl Pts',(0.325084129822677,-1.40296674794631,
13.5052012864122));
#23533=CARTESIAN_POINT('Ctrl Pts',(0.315348432130469,-1.39963998647743,
13.5966967078372));
#23534=CARTESIAN_POINT('Ctrl Pts',(0.295775690609116,-1.37522960445915,
13.7776009944865));
#23535=CARTESIAN_POINT('Ctrl Pts',(0.285989779203554,-1.35422922945079,
13.8665816749947));
#23536=CARTESIAN_POINT('Ctrl Pts',(0.266421317507451,-1.29515206523774,
14.0393867564002));
#23537=CARTESIAN_POINT('Ctrl Pts',(0.256660776143199,-1.25717829009425,
14.1227838801369));
#23538=CARTESIAN_POINT('Ctrl Pts',(0.237071198525041,-1.16550271994426,
14.2810026863609));
#23539=CARTESIAN_POINT('Ctrl Pts',(0.227285202486673,-1.11201669976392,
14.3554417807662));
#23540=CARTESIAN_POINT('Ctrl Pts',(0.207690579985672,-0.991283909256496,
14.492834862049));
#23541=CARTESIAN_POINT('Ctrl Pts',(0.197914985592649,-0.924324804420834,
14.555456496884));
#23542=CARTESIAN_POINT('Ctrl Pts',(0.178363730211615,-0.77956034377627,
14.6664291133161));
#23543=CARTESIAN_POINT('Ctrl Pts',(0.168653455761846,-0.702161868325127,
14.714594487812));
#23544=CARTESIAN_POINT('Ctrl Pts',(0.154931884130335,-0.587493405545037,
14.7713060468275));
#23545=CARTESIAN_POINT('Ctrl Pts',(0.150957159681852,-0.553710047719918,
14.7863796373724));
#23546=CARTESIAN_POINT('Ctrl Pts',(0.127324858889503,-0.349250469145506,
14.8680583278928));
#23547=CARTESIAN_POINT('Ctrl Pts',(0.108116044219979,-0.167433982443867,
14.9019724727693));
#23548=CARTESIAN_POINT('Ctrl Pts',(0.0835087904628999,0.0614075991326112,
14.8993976932663));
#23549=CARTESIAN_POINT('Ctrl Pts',(0.0785922418302401,0.107011311437968,
14.8966507365185));
#23550=CARTESIAN_POINT('Ctrl Pts',(0.0539490465634395,0.334401323629049,
14.8717499795437));
#23551=CARTESIAN_POINT('Ctrl Pts',(0.0346178541707623,0.510744903939716,
14.8163078569111));
#23552=CARTESIAN_POINT('Ctrl Pts',(0.00524394571155688,0.751512883388005,
14.6847193706286));
#23553=CARTESIAN_POINT('Ctrl Pts',(-0.00449437637938378,0.827135223948516,
14.633216073014));
#23554=CARTESIAN_POINT('Ctrl Pts',(-0.0239809671530538,0.966665453230061,
14.5167327070529));
#23555=CARTESIAN_POINT('Ctrl Pts',(-0.0336895932364449,1.03034167195237,
14.4521467881692));
#23556=CARTESIAN_POINT('Ctrl Pts',(-0.0482825683721452,1.11609336739054,
14.3464156472311));
#23557=CARTESIAN_POINT('Ctrl Pts',(-0.053164629659224,1.14309714236796,
14.309575719996));
#23558=CARTESIAN_POINT('Ctrl Pts',(-0.0677481618582202,1.21817300793428,
14.1958885992343));
#23559=CARTESIAN_POINT('Ctrl Pts',(-0.0774376677821613,1.26063801176348,
14.1156280639987));
#23560=CARTESIAN_POINT('Ctrl Pts',(-0.092038069202919,1.31239243389686,
13.989602038624));
#23561=CARTESIAN_POINT('Ctrl Pts',(-0.0969214262161361,1.32765868048064,
13.9465495779731));
#23562=CARTESIAN_POINT('Ctrl Pts',(-0.111558553938572,1.36698955369234,
13.8156386792069));
#23563=CARTESIAN_POINT('Ctrl Pts',(-0.121301079176293,1.38461760607521,
13.726101915061));
#23564=CARTESIAN_POINT('Ctrl Pts',(-0.135956737723329,1.39784990153599,
13.5900170563907));
#23565=CARTESIAN_POINT('Ctrl Pts',(-0.140847394293321,1.40004291833416,
13.5443539040244));
#23566=CARTESIAN_POINT('Ctrl Pts',(-0.150635935487247,1.39995582251888,
13.4529906466906));
#23567=CARTESIAN_POINT('Ctrl Pts',(-0.155528014375707,1.3976771103293,13.4073453936515));
#23568=CARTESIAN_POINT('Ctrl Pts',(-0.165317128395896,1.38866429108346,
13.3164271729165));
#23569=CARTESIAN_POINT('Ctrl Pts',(-0.170208300733083,1.38193418373819,
13.2712088297759));
#23570=CARTESIAN_POINT('Ctrl Pts',(-0.179996367698184,1.36408470341974,
13.1816346357667));
#23571=CARTESIAN_POINT('Ctrl Pts',(-0.184887463766744,1.35298011079629,
13.1373315573546));
#23572=CARTESIAN_POINT('Ctrl Pts',(-0.194676525210845,1.32646843542118,
13.0499227933076));
#23573=CARTESIAN_POINT('Ctrl Pts',(-0.199568583723516,1.31107267433573,
13.0068707570027));
#23574=CARTESIAN_POINT('Ctrl Pts',(-0.224133279370017,1.22341634625858,
12.7950618050139));
#23575=CARTESIAN_POINT('Ctrl Pts',(-0.243582772426096,1.12056594042943,
12.6409215730407));
#23576=CARTESIAN_POINT('Ctrl Pts',(-0.268223405498791,0.958500833830214,
12.4785393669544));
#23577=CARTESIAN_POINT('Ctrl Pts',(-0.273127971641192,0.924505941863352,
12.4476717361654));
#23578=CARTESIAN_POINT('Ctrl Pts',(-0.287763435569983,0.818663282345703,
12.360660590545));
#23579=CARTESIAN_POINT('Ctrl Pts',(-0.297460822492334,0.742790149119399,
12.3098041868957));
#23580=CARTESIAN_POINT('Ctrl Pts',(-0.316837758362703,0.583558266532999,
12.2242675683729));
#23581=CARTESIAN_POINT('Ctrl Pts',(-0.326471785116992,0.500710003383573,
12.1895335380189));
#23582=CARTESIAN_POINT('Ctrl Pts',(-0.355703250292568,0.241025341260821,
12.1089086515452));
#23583=CARTESIAN_POINT('Ctrl Pts',(-0.374841164489171,0.0580452120556191,
12.0893760843612));
#23584=CARTESIAN_POINT('Ctrl Pts',(-0.404054607129763,-0.21295706204091,
12.1133822289271));
#23585=CARTESIAN_POINT('Ctrl Pts',(-0.413718349790429,-0.301412881187743,
12.129886898215));
#23586=CARTESIAN_POINT('Ctrl Pts',(-0.424419123574571,-0.39731761879081,
12.1575249144134));
#23587=CARTESIAN_POINT('Ctrl Pts',(-0.425493451182981,-0.406924727303341,
12.1604057326115));
#23588=CARTESIAN_POINT('Ctrl Pts',(-0.426566464895915,-0.416497451671893,
12.1633886605483));
#23589=CARTESIAN_POINT('Origin',(0.,0.,13.5));
#23590=CARTESIAN_POINT('',(-1.54907858904864,-0.416497429633284,12.1633886536809));
#23591=CARTESIAN_POINT('',(-1.36903602092574,-0.416497450391696,12.1633886601494));
#23592=CARTESIAN_POINT('',(0.,-0.416497449530544,12.1633886598811));
#23593=CARTESIAN_POINT('Ctrl Pts',(-1.54907858904864,-0.416497429633283,
12.1633886536809));
#23594=CARTESIAN_POINT('Ctrl Pts',(-1.5406601768603,-0.341467258642645,
12.1400087284329));
#23595=CARTESIAN_POINT('Ctrl Pts',(-1.53223076875421,-0.264582379274244,
12.1229820008525));
#23596=CARTESIAN_POINT('Ctrl Pts',(-1.51405475451702,-0.0967165221040692,
12.1003995460753));
#23597=CARTESIAN_POINT('Ctrl Pts',(-1.50438038760605,-0.00581264136751285,
12.0970737445648));
#23598=CARTESIAN_POINT('Ctrl Pts',(-1.48499579176796,0.174894239452828,
12.1080359841145));
#23599=CARTESIAN_POINT('Ctrl Pts',(-1.47532269477495,0.264275420538007,
12.1222082992012));
#23600=CARTESIAN_POINT('Ctrl Pts',(-1.4559898682012,0.438783328667831,12.1674949504344));
#23601=CARTESIAN_POINT('Ctrl Pts',(-1.44641307495146,0.523518550496798,
12.1984511731486));
#23602=CARTESIAN_POINT('Ctrl Pts',(-1.41723115468807,0.769798342132802,
12.3163948316969));
#23603=CARTESIAN_POINT('Ctrl Pts',(-1.39765278865023,0.917799738045793,
12.4270818124817));
#23604=CARTESIAN_POINT('Ctrl Pts',(-1.36830303425761,1.10138944928039,12.630935239729));
#23605=CARTESIAN_POINT('Ctrl Pts',(-1.35856878431637,1.15569532346242,12.7045753741589));
#23606=CARTESIAN_POINT('Ctrl Pts',(-1.33898672035889,1.24928999982123,12.8615328485505));
#23607=CARTESIAN_POINT('Ctrl Pts',(-1.32920497571206,1.28832329599532,12.944492458197));
#23608=CARTESIAN_POINT('Ctrl Pts',(-1.31012567309657,1.34793079918636,13.1120084287429));
#23609=CARTESIAN_POINT('Ctrl Pts',(-1.30085354674442,1.36928881084673,13.195857172909));
#23610=CARTESIAN_POINT('Ctrl Pts',(-1.27636586378979,1.4049429148567,13.421120658934));
#23611=CARTESIAN_POINT('Ctrl Pts',(-1.26143470085253,1.40571524860204,13.563662147314));
#23612=CARTESIAN_POINT('Ctrl Pts',(-1.23123469457865,1.36454425423093,13.8433548834731));
#23613=CARTESIAN_POINT('Ctrl Pts',(-1.21608201599808,1.32306591394079,13.9789211786688));
#23614=CARTESIAN_POINT('Ctrl Pts',(-1.19116793334073,1.22295966287602,14.1874056751138));
#23615=CARTESIAN_POINT('Ctrl Pts',(-1.18154744554627,1.1760789529253,14.2648507244898));
#23616=CARTESIAN_POINT('Ctrl Pts',(-1.15228241326668,1.0120831148425,14.4846360297138));
#23617=CARTESIAN_POINT('Ctrl Pts',(-1.13281234829334,0.874135765416674,
14.6089193614054));
#23618=CARTESIAN_POINT('Ctrl Pts',(-1.1046516246046,0.648893779113152,14.7430038285068));
#23619=CARTESIAN_POINT('Ctrl Pts',(-1.09623154730318,0.578426543600241,
14.7773192602803));
#23620=CARTESIAN_POINT('Ctrl Pts',(-1.07827921096874,0.422219105135024,
14.8377963745812));
#23621=CARTESIAN_POINT('Ctrl Pts',(-1.06881041043044,0.336081057265623,
14.8619906736324));
#23622=CARTESIAN_POINT('Ctrl Pts',(-1.03931196184981,0.0638887425558035,
14.9110284431873));
#23623=CARTESIAN_POINT('Ctrl Pts',(-1.01924554289577,-0.125246622046433,
14.9069085771062));
#23624=CARTESIAN_POINT('Ctrl Pts',(-0.989427198333877,-0.396709589278914,
14.8456968435733));
#23625=CARTESIAN_POINT('Ctrl Pts',(-0.979747013658032,-0.483306516047289,
14.8170777504331));
#23626=CARTESIAN_POINT('Ctrl Pts',(-0.950619670555937,-0.732398469067639,
14.7068548157767));
#23627=CARTESIAN_POINT('Ctrl Pts',(-0.93129645471337,-0.882445703779912,
14.6019050418648));
#23628=CARTESIAN_POINT('Ctrl Pts',(-0.906998790584779,-1.03992217926085,
14.4384245136461));
#23629=CARTESIAN_POINT('Ctrl Pts',(-0.902127602436768,-1.06992979208714,
14.4040624864748));
#23630=CARTESIAN_POINT('Ctrl Pts',(-0.887481419388395,-1.15484462150804,
14.2966637353185));
#23631=CARTESIAN_POINT('Ctrl Pts',(-0.877714846127587,-1.20433645683066,
14.2196612259094));
#23632=CARTESIAN_POINT('Ctrl Pts',(-0.858105037739448,-1.28765509093986,
14.0570447439249));
#23633=CARTESIAN_POINT('Ctrl Pts',(-0.848336101586714,-1.32126823889005,
13.9718104088243));
#23634=CARTESIAN_POINT('Ctrl Pts',(-0.828815227017753,-1.37123717891394,
13.7965742090084));
#23635=CARTESIAN_POINT('Ctrl Pts',(-0.819088224933466,-1.38758415073027,
13.70702194967));
#23636=CARTESIAN_POINT('Ctrl Pts',(-0.799625119408226,-1.40272113880701,
13.5257793559006));
#23637=CARTESIAN_POINT('Ctrl Pts',(-0.789925667583875,-1.40142889436572,
13.4345167996021));
#23638=CARTESIAN_POINT('Ctrl Pts',(-0.770481057338387,-1.38121325807439,
13.2541906062254));
#23639=CARTESIAN_POINT('Ctrl Pts',(-0.760781272839151,-1.36246400098675,
13.1655392050373));
#23640=CARTESIAN_POINT('Ctrl Pts',(-0.741285534984833,-1.30782631815192,
12.9921124871005));
#23641=CARTESIAN_POINT('Ctrl Pts',(-0.73152636222953,-1.27187594788111,
12.9078081282214));
#23642=CARTESIAN_POINT('Ctrl Pts',(-0.711956793810037,-1.18413070434302,
12.7475613086016));
#23643=CARTESIAN_POINT('Ctrl Pts',(-0.702191074851079,-1.13257481192257,
12.6719880898317));
#23644=CARTESIAN_POINT('Ctrl Pts',(-0.687515128589093,-1.04472172005135,
12.5669166485645));
#23645=CARTESIAN_POINT('Ctrl Pts',(-0.682623587019187,-1.01371214468988,
12.533317165612));
#23646=CARTESIAN_POINT('Ctrl Pts',(-0.667943407696058,-0.915978980449471,
12.4373053893992));
#23647=CARTESIAN_POINT('Ctrl Pts',(-0.658177088437864,-0.844738418762731,
12.3798418084721));
#23648=CARTESIAN_POINT('Ctrl Pts',(-0.643521699190297,-0.730382585888922,
12.3047548168733));
#23649=CARTESIAN_POINT('Ctrl Pts',(-0.638653607585438,-0.691158639037145,
12.2816529733307));
#23650=CARTESIAN_POINT('Ctrl Pts',(-0.624913176954061,-0.577673895825769,
12.2220603506758));
#23651=CARTESIAN_POINT('Ctrl Pts',(-0.616028611275531,-0.501204185921513,
12.1901786140452));
#23652=CARTESIAN_POINT('Ctrl Pts',(-0.606981870383497,-0.42041157768316,
12.1646130483831));
#23653=CARTESIAN_POINT('Ctrl Pts',(-0.606762975409993,-0.41845516022692,
12.1639986962372));
#23654=CARTESIAN_POINT('Ctrl Pts',(-0.606544106580495,-0.416497449298501,
12.1633886598088));
#23655=CARTESIAN_POINT('Ctrl Pts',(-0.426566464895916,-0.416497451671892,
12.1633886605483));
#23656=CARTESIAN_POINT('Ctrl Pts',(-0.436856069340607,-0.508294551767764,
12.1919932796566));
#23657=CARTESIAN_POINT('Ctrl Pts',(-0.447040629083815,-0.59692816148061,
12.2299871481661));
#23658=CARTESIAN_POINT('Ctrl Pts',(-0.476149466322508,-0.83511538098895,
12.3625904307335));
#23659=CARTESIAN_POINT('Ctrl Pts',(-0.495150053700609,-0.971644105280062,
12.4767602650293));
#23660=CARTESIAN_POINT('Ctrl Pts',(-0.521283783031458,-1.12612952048971,
12.6654996575978));
#23661=CARTESIAN_POINT('Ctrl Pts',(-0.528447086558006,-1.16506077741258,
12.7207742336957));
#23662=CARTESIAN_POINT('Ctrl Pts',(-0.550935070772576,-1.27412220508858,
12.9021793696774));
#23663=CARTESIAN_POINT('Ctrl Pts',(-0.566218063130956,-1.32886280026531,
13.0364339089676));
#23664=CARTESIAN_POINT('Ctrl Pts',(-0.591343705020871,-1.38258883934397,
13.2627643601562));
#23665=CARTESIAN_POINT('Ctrl Pts',(-0.600938265013163,-1.39481826377124,
13.3506184312601));
#23666=CARTESIAN_POINT('Ctrl Pts',(-0.619721830656807,-1.40240900477448,
13.5247749214712));
#23667=CARTESIAN_POINT('Ctrl Pts',(-0.628824778906351,-1.39825516663194,
13.61067680339));
#23668=CARTESIAN_POINT('Ctrl Pts',(-0.646212924619432,-1.37533891727802,
13.7730353808866));
#23669=CARTESIAN_POINT('Ctrl Pts',(-0.654477069604567,-1.35796056198493,
13.8493535325463));
#23670=CARTESIAN_POINT('Ctrl Pts',(-0.669299655442823,-1.31587716252923,
13.9818440834017));
#23671=CARTESIAN_POINT('Ctrl Pts',(-0.675815032393579,-1.29368274942276,
14.0386005730431));
#23672=CARTESIAN_POINT('Ctrl Pts',(-0.692220433519471,-1.22904882393156,
14.1766217490664));
#23673=CARTESIAN_POINT('Ctrl Pts',(-0.702125852709566,-1.18219577255753,
14.2555067173899));
#23674=CARTESIAN_POINT('Ctrl Pts',(-0.725294061861772,-1.0550557000675,
14.4284481301938));
#23675=CARTESIAN_POINT('Ctrl Pts',(-0.738308575104036,-0.96936000748964,
14.5175967454973));
#23676=CARTESIAN_POINT('Ctrl Pts',(-0.771095147590407,-0.728704749111746,
14.7095919635518));
#23677=CARTESIAN_POINT('Ctrl Pts',(-0.790886881321988,-0.562925190647617,
14.7950800433673));
#23678=CARTESIAN_POINT('Ctrl Pts',(-0.822223990982272,-0.28168981208092,
14.8756008001747));
#23679=CARTESIAN_POINT('Ctrl Pts',(-0.833650660513492,-0.174944210460729,
14.8932055858379));
#23680=CARTESIAN_POINT('Ctrl Pts',(-0.864350735910949,0.111628812394898,
14.9069849291186));
#23681=CARTESIAN_POINT('Ctrl Pts',(-0.883559305371559,0.290497728729643,
14.8811880074753));
#23682=CARTESIAN_POINT('Ctrl Pts',(-0.912360850008062,0.545294985669325,
14.7926231989879));
#23683=CARTESIAN_POINT('Ctrl Pts',(-0.922009061556224,0.627844285719284,
14.7546044436973));
#23684=CARTESIAN_POINT('Ctrl Pts',(-0.941429641103666,0.784320502320354,
14.6632025432421));
#23685=CARTESIAN_POINT('Ctrl Pts',(-0.951157831762751,0.857890680035994,
14.6100549109342));
#23686=CARTESIAN_POINT('Ctrl Pts',(-0.970603595769792,0.99374928117037,
14.4902854078429));
#23687=CARTESIAN_POINT('Ctrl Pts',(-0.980243707293165,1.05571606782114,
14.4239408539999));
#23688=CARTESIAN_POINT('Ctrl Pts',(-0.994838580468196,1.13861676189503,
14.3158644134718));
#23689=CARTESIAN_POINT('Ctrl Pts',(-0.999727647061573,1.16460628651257,
14.2783155451848));
#23690=CARTESIAN_POINT('Ctrl Pts',(-1.01441146505272,1.23702331607857,14.1619183483613));
#23691=CARTESIAN_POINT('Ctrl Pts',(-1.02418705320635,1.27760755818296,14.0797253990493));
#23692=CARTESIAN_POINT('Ctrl Pts',(-1.03887470254296,1.32601335702106,13.9514156711329));
#23693=CARTESIAN_POINT('Ctrl Pts',(-1.04376480430155,1.34003821962249,13.9079032807479));
#23694=CARTESIAN_POINT('Ctrl Pts',(-1.05355449742676,1.36378158168263,13.81966697846));
#23695=CARTESIAN_POINT('Ctrl Pts',(-1.05844747059606,1.37348622838814,13.77499593399));
#23696=CARTESIAN_POINT('Ctrl Pts',(-1.07313867235388,1.39600857517004,13.6397241422986));
#23697=CARTESIAN_POINT('Ctrl Pts',(-1.08290931164055,1.40215313332635,13.5482629108958));
#23698=CARTESIAN_POINT('Ctrl Pts',(-1.10250933181918,1.39651712469916,13.3654539108859));
#23699=CARTESIAN_POINT('Ctrl Pts',(-1.11227241806947,1.3847500654353,13.2745447561302));
#23700=CARTESIAN_POINT('Ctrl Pts',(-1.13184640717828,1.34369127902684,13.0964815911587));
#23701=CARTESIAN_POINT('Ctrl Pts',(-1.14161942173393,1.31452875233355,13.0097474187859));
#23702=CARTESIAN_POINT('Ctrl Pts',(-1.15628531409457,1.25841897095193,12.8848023314274));
#23703=CARTESIAN_POINT('Ctrl Pts',(-1.16117209841051,1.23767832878196,12.8440740817254));
#23704=CARTESIAN_POINT('Ctrl Pts',(-1.17582898554725,1.16970591158298,12.7253430500136));
#23705=CARTESIAN_POINT('Ctrl Pts',(-1.18559009693822,1.1168129127689,12.6508625288843));
#23706=CARTESIAN_POINT('Ctrl Pts',(-1.2050522836408,0.997571959916159,12.5135512491387));
#23707=CARTESIAN_POINT('Ctrl Pts',(-1.21472655783085,0.9315683882803,12.4509951955105));
#23708=CARTESIAN_POINT('Ctrl Pts',(-1.229337525625,0.82398700372118,12.3672485533638));
#23709=CARTESIAN_POINT('Ctrl Pts',(-1.23422763508291,0.786647482698989,
12.3410064175952));
#23710=CARTESIAN_POINT('Ctrl Pts',(-1.24892256039466,0.670828831577373,
12.2677888014863));
#23711=CARTESIAN_POINT('Ctrl Pts',(-1.25868707861522,0.588965527511864,
12.22662839331));
#23712=CARTESIAN_POINT('Ctrl Pts',(-1.27822616168259,0.41908910589679,12.1611261320018));
#23713=CARTESIAN_POINT('Ctrl Pts',(-1.28795438003646,0.331530453908728,
12.1368025075342));
#23714=CARTESIAN_POINT('Ctrl Pts',(-1.31333296220026,0.0975617312448524,
12.0957002236768));
#23715=CARTESIAN_POINT('Ctrl Pts',(-1.3288531321092,-0.0502088032899908,
12.0932117268099));
#23716=CARTESIAN_POINT('Ctrl Pts',(-1.35276419127933,-0.270507663066689,
12.1243034285597));
#23717=CARTESIAN_POINT('Ctrl Pts',(-1.36090638824632,-0.344364594037876,
12.1409115571464));
#23718=CARTESIAN_POINT('Ctrl Pts',(-1.36903602092574,-0.416497450391695,
12.1633886601494));
#23719=CARTESIAN_POINT('Origin',(0.,0.,13.5));
#23720=CARTESIAN_POINT('',(-2.49153227027379,-0.416497403609636,12.1633886455718));
#23721=CARTESIAN_POINT('',(-2.31145225782316,-0.416497494886935,12.1633886740144));
#23722=CARTESIAN_POINT('',(0.,-0.416497449530544,12.1633886598811));
#23723=CARTESIAN_POINT('Ctrl Pts',(-2.49153227027379,-0.416497403609637,
12.1633886455718));
#23724=CARTESIAN_POINT('Ctrl Pts',(-2.48377759386758,-0.347468400922449,
12.1418787277503));
#23725=CARTESIAN_POINT('Ctrl Pts',(-2.47601354514147,-0.276847582414752,
12.1257394777351));
#23726=CARTESIAN_POINT('Ctrl Pts',(-2.46337215890503,-0.160100728167568,
12.1084352599308));
#23727=CARTESIAN_POINT('Ctrl Pts',(-2.45849711705798,-0.114634837042245,
12.1039542840005));
#23728=CARTESIAN_POINT('Ctrl Pts',(-2.43419614037067,0.112519097027662,
12.0927401847591));
#23729=CARTESIAN_POINT('Ctrl Pts',(-2.41480592826936,0.294086936803198,
12.1192203848806));
#23730=CARTESIAN_POINT('Ctrl Pts',(-2.38556824782432,0.551677657416333,
12.2100390762164));
#23731=CARTESIAN_POINT('Ctrl Pts',(-2.37582669014715,0.634662303048093,
12.2487801906221));
#23732=CARTESIAN_POINT('Ctrl Pts',(-2.36115008617931,0.752488449996106,
12.3185443183758));
#23733=CARTESIAN_POINT('Ctrl Pts',(-2.35626398826519,0.790541390226631,
12.3436606570512));
#23734=CARTESIAN_POINT('Ctrl Pts',(-2.34168031498338,0.900246641204636,
12.4240204249908));
#23735=CARTESIAN_POINT('Ctrl Pts',(-2.33204530358468,0.967844787647961,
12.4843952604642));
#23736=CARTESIAN_POINT('Ctrl Pts',(-2.30287250743473,1.15279927099767,12.684941919434));
#23737=CARTESIAN_POINT('Ctrl Pts',(-2.28340827706671,1.24906570563351,12.8418966503144));
#23738=CARTESIAN_POINT('Ctrl Pts',(-2.25411301591339,1.34430474565109,13.098518628679));
#23739=CARTESIAN_POINT('Ctrl Pts',(-2.24437372807563,1.36762809005532,13.1870532149905));
#23740=CARTESIAN_POINT('Ctrl Pts',(-2.22478159000079,1.39670824504616,13.3674755372028));
#23741=CARTESIAN_POINT('Ctrl Pts',(-2.21498909654132,1.40238025146898,13.4589340742773));
#23742=CARTESIAN_POINT('Ctrl Pts',(-2.18568716103912,1.39255584062942,13.7322520605856));
#23743=CARTESIAN_POINT('Ctrl Pts',(-2.16633857511812,1.35057933199256,13.9112040608549));
#23744=CARTESIAN_POINT('Ctrl Pts',(-2.14198168246296,1.25674829820127,14.1185938447382));
#23745=CARTESIAN_POINT('Ctrl Pts',(-2.13711836627855,1.23595875252239,14.1591514505222));
#23746=CARTESIAN_POINT('Ctrl Pts',(-2.11614875473995,1.13808286942347,14.32912266523));
#23747=CARTESIAN_POINT('Ctrl Pts',(-2.10003915852141,1.04237141114805,14.4466453455716));
#23748=CARTESIAN_POINT('Ctrl Pts',(-2.07902261227106,0.895684084578088,
14.5769547781812));
#23749=CARTESIAN_POINT('Ctrl Pts',(-2.07415016887986,0.860113650291088,
14.6055705253448));
#23750=CARTESIAN_POINT('Ctrl Pts',(-2.04970556948249,0.675127730358556,
14.7400480198235));
#23751=CARTESIAN_POINT('Ctrl Pts',(-2.03017148796127,0.507359241860883,
14.817612551329));
#23752=CARTESIAN_POINT('Ctrl Pts',(-2.00082455849128,0.240662255076382,
14.8821802881563));
#23753=CARTESIAN_POINT('Ctrl Pts',(-1.99109139201528,0.150010486708826,
14.8949326508275));
#23754=CARTESIAN_POINT('Ctrl Pts',(-1.97133043004739,-0.0341083947857306,
14.9026679937534));
#23755=CARTESIAN_POINT('Ctrl Pts',(-1.96134793998215,-0.127141301000997,
14.8973103419758));
#23756=CARTESIAN_POINT('Ctrl Pts',(-1.94650726074608,-0.264019383396102,
14.8756363941141));
#23757=CARTESIAN_POINT('Ctrl Pts',(-1.94163609258797,-0.308708703192616,
14.8663018582216));
#23758=CARTESIAN_POINT('Ctrl Pts',(-1.91945790680511,-0.509566913570251,
14.8139876521769));
#23759=CARTESIAN_POINT('Ctrl Pts',(-1.90216586855344,-0.658006283194157,
14.7462935509965));
#23760=CARTESIAN_POINT('Ctrl Pts',(-1.87507752023587,-0.866521505981471,
14.6033581069912));
#23761=CARTESIAN_POINT('Ctrl Pts',(-1.86539795153523,-0.936297771913995,
14.5447991730715));
#23762=CARTESIAN_POINT('Ctrl Pts',(-1.84597259989742,-1.06326139298109,
14.4152424783883));
#23763=CARTESIAN_POINT('Ctrl Pts',(-1.8362713986498,-1.12019802305971,14.3446004003708));
#23764=CARTESIAN_POINT('Ctrl Pts',(-1.81678516152418,-1.22009380401549,
14.1926161974074));
#23765=CARTESIAN_POINT('Ctrl Pts',(-1.80703971528604,-1.26267897580898,
14.1115453629672));
#23766=CARTESIAN_POINT('Ctrl Pts',(-1.78887058392302,-1.32642166587171,
13.9546328582154));
#23767=CARTESIAN_POINT('Ctrl Pts',(-1.78049468158165,-1.34968935628625,
13.8800317236812));
#23768=CARTESIAN_POINT('Ctrl Pts',(-1.76250218670362,-1.38611096094181,
13.7162361092004));
#23769=CARTESIAN_POINT('Ctrl Pts',(-1.75295731014169,-1.39712351726591,
13.6269174236735));
#23770=CARTESIAN_POINT('Ctrl Pts',(-1.72377142004812,-1.40437243116028,
13.353908122551));
#23771=CARTESIAN_POINT('Ctrl Pts',(-1.70415058337538,-1.3731989144026,13.1714742819655));
#23772=CARTESIAN_POINT('Ctrl Pts',(-1.67478380946666,-1.27514573804416,
12.9148925399848));
#23773=CARTESIAN_POINT('Ctrl Pts',(-1.66505071523327,-1.23425531818042,
12.8329460698071));
#23774=CARTESIAN_POINT('Ctrl Pts',(-1.64547168751001,-1.13704679109676,
12.6781193062635));
#23775=CARTESIAN_POINT('Ctrl Pts',(-1.63568267335985,-1.08094703361817,
12.6056193489201));
#23776=CARTESIAN_POINT('Ctrl Pts',(-1.62099125749229,-0.986817086254176,
12.5058772385525));
#23777=CARTESIAN_POINT('Ctrl Pts',(-1.61609821231226,-0.953846142866909,
12.4742000397494));
#23778=CARTESIAN_POINT('Ctrl Pts',(-1.60146146019077,-0.850811108408571,
12.3844783193595));
#23779=CARTESIAN_POINT('Ctrl Pts',(-1.59173204114866,-0.776582088982317,
12.3315872605324));
#23780=CARTESIAN_POINT('Ctrl Pts',(-1.57226834088642,-0.619119849626152,
12.2410651847151));
#23781=CARTESIAN_POINT('Ctrl Pts',(-1.56260707085518,-0.536281388983477,
12.2036093642709));
#23782=CARTESIAN_POINT('Ctrl Pts',(-1.55162440893478,-0.439145982974093,
12.1706045824513));
#23783=CARTESIAN_POINT('Ctrl Pts',(-1.55035155684989,-0.427842917316238,
12.1669239868733));
#23784=CARTESIAN_POINT('Ctrl Pts',(-1.54907858904864,-0.416497429633283,
12.1633886536809));
#23785=CARTESIAN_POINT('Ctrl Pts',(-1.36903602092574,-0.416497450391695,
12.1633886601494));
#23786=CARTESIAN_POINT('Ctrl Pts',(-1.37055630404986,-0.429986665530214,
12.1675919940173));
#23787=CARTESIAN_POINT('Ctrl Pts',(-1.37207596709313,-0.443415607308437,
12.1720005753452));
#23788=CARTESIAN_POINT('Ctrl Pts',(-1.38016695316969,-0.514617638283364,
12.1965766368901));
#23789=CARTESIAN_POINT('Ctrl Pts',(-1.38668001305955,-0.57108368251163,
12.2203096644137));
#23790=CARTESIAN_POINT('Ctrl Pts',(-1.40296155657829,-0.707169183262192,
12.2883142054731));
#23791=CARTESIAN_POINT('Ctrl Pts',(-1.4126955046026,-0.784366074695015,
12.3367973222343));
#23792=CARTESIAN_POINT('Ctrl Pts',(-1.42733008015005,-0.892470436642723,
12.42037724037));
#23793=CARTESIAN_POINT('Ctrl Pts',(-1.43222273412454,-0.927236836738582,
12.4500854254159));
#23794=CARTESIAN_POINT('Ctrl Pts',(-1.44201572448199,-0.993737226622791,
12.5127943896425));
#23795=CARTESIAN_POINT('Ctrl Pts',(-1.44690951607711,-1.02543152920955,
12.5457574910582));
#23796=CARTESIAN_POINT('Ctrl Pts',(-1.46160331503236,-1.11552634929339,
12.6491412336523));
#23797=CARTESIAN_POINT('Ctrl Pts',(-1.47136592281737,-1.16869919717314,
12.7237900733827));
#23798=CARTESIAN_POINT('Ctrl Pts',(-1.4909596634891,-1.25972038856916,12.882374098493));
#23799=CARTESIAN_POINT('Ctrl Pts',(-1.50073942681233,-1.29735262604247,
12.9659275401047));
#23800=CARTESIAN_POINT('Ctrl Pts',(-1.52029606830947,-1.35569686312962,
13.1389029286828));
#23801=CARTESIAN_POINT('Ctrl Pts',(-1.53000129719526,-1.37632231821543,
13.2278933038496));
#23802=CARTESIAN_POINT('Ctrl Pts',(-1.54953196511918,-1.40000539138166,
13.4087824924846));
#23803=CARTESIAN_POINT('Ctrl Pts',(-1.55931752269324,-1.40297366362121,
13.5002514645915));
#23804=CARTESIAN_POINT('Ctrl Pts',(-1.58881724745846,-1.38503995608772,
13.7744997609866));
#23805=CARTESIAN_POINT('Ctrl Pts',(-1.60827700302614,-1.33716438228231,
13.9535192941375));
#23806=CARTESIAN_POINT('Ctrl Pts',(-1.63279556542512,-1.23595895928569,
14.1591580854752));
#23807=CARTESIAN_POINT('Ctrl Pts',(-1.63767465958672,-1.21381003363761,
14.1991059284103));
#23808=CARTESIAN_POINT('Ctrl Pts',(-1.65234396474022,-1.14159072792032,
14.3155483615572));
#23809=CARTESIAN_POINT('Ctrl Pts',(-1.66213210403576,-1.08594656988133,
14.3882950615527));
#23810=CARTESIAN_POINT('Ctrl Pts',(-1.69154038888768,-0.898932281795321,
14.5887250831049));
#23811=CARTESIAN_POINT('Ctrl Pts',(-1.7108834370603,-0.749282123885,14.6966528911975));
#23812=CARTESIAN_POINT('Ctrl Pts',(-1.74026139106864,-0.500243991061622,
14.8107508678375));
#23813=CARTESIAN_POINT('Ctrl Pts',(-1.75004056336101,-0.413847590560855,
14.8405379461715));
#23814=CARTESIAN_POINT('Ctrl Pts',(-1.7798787288382,-0.143192886693771,
14.9051692043203));
#23815=CARTESIAN_POINT('Ctrl Pts',(-1.79951934952144,0.0456593073224952,
14.911707423503));
#23816=CARTESIAN_POINT('Ctrl Pts',(-1.82928632628386,0.318590552131681,
14.8662099324968));
#23817=CARTESIAN_POINT('Ctrl Pts',(-1.83894752496594,0.405360836840588,
14.8430236418812));
#23818=CARTESIAN_POINT('Ctrl Pts',(-1.85883289055153,0.579108170720027,
14.7782087981025));
#23819=CARTESIAN_POINT('Ctrl Pts',(-1.86900114187339,0.665222765504545,
14.7355822452673));
#23820=CARTESIAN_POINT('Ctrl Pts',(-1.88903956520451,0.823694474386146,
14.6357348058695));
#23821=CARTESIAN_POINT('Ctrl Pts',(-1.89883311377528,0.896115948541066,
14.5795100191461));
#23822=CARTESIAN_POINT('Ctrl Pts',(-1.92824791000986,1.09530820757515,14.3909163792467));
#23823=CARTESIAN_POINT('Ctrl Pts',(-1.94779722878606,1.20218403566685,14.240399190362));
#23824=CARTESIAN_POINT('Ctrl Pts',(-1.97682766485052,1.31382113728833,13.9918391985901));
#23825=CARTESIAN_POINT('Ctrl Pts',(-1.98633002286068,1.34260384155628,13.9067507459095));
#23826=CARTESIAN_POINT('Ctrl Pts',(-2.0120400414814,1.39747926223019,13.6726392534436));
#23827=CARTESIAN_POINT('Ctrl Pts',(-2.02828849510217,1.40794165964757,13.5211808202616));
#23828=CARTESIAN_POINT('Ctrl Pts',(-2.05497486306235,1.38505568715582,13.2738684574458));
#23829=CARTESIAN_POINT('Ctrl Pts',(-2.06533068198525,1.36594077564537,13.177941121327));
#23830=CARTESIAN_POINT('Ctrl Pts',(-2.08552170664394,1.30985235566511,12.997336518746));
#23831=CARTESIAN_POINT('Ctrl Pts',(-2.09529461618589,1.27418345627835,12.9127694663235));
#23832=CARTESIAN_POINT('Ctrl Pts',(-2.12465204047475,1.14343094971824,12.6718056249336));
#23833=CARTESIAN_POINT('Ctrl Pts',(-2.14414013309284,1.0257830350729,12.5298908410156));
#23834=CARTESIAN_POINT('Ctrl Pts',(-2.17335866262273,0.813545005322425,
12.3569986300674));
#23835=CARTESIAN_POINT('Ctrl Pts',(-2.18306730770509,0.737427447863767,
12.3064726590416));
#23836=CARTESIAN_POINT('Ctrl Pts',(-2.20253472026112,0.577156163115864,
12.2213075788084));
#23837=CARTESIAN_POINT('Ctrl Pts',(-2.21224818242629,0.493451613008539,
12.1867335142098));
#23838=CARTESIAN_POINT('Ctrl Pts',(-2.23754581469018,0.267832394698486,
12.1181815529036));
#23839=CARTESIAN_POINT('Ctrl Pts',(-2.2529785965965,0.12291760233651,12.0978415590498));
#23840=CARTESIAN_POINT('Ctrl Pts',(-2.28294885814402,-0.156439897817064,
12.1023354354469));
#23841=CARTESIAN_POINT('Ctrl Pts',(-2.29715378790174,-0.289106120400033,
12.1236926252734));
#23842=CARTESIAN_POINT('Ctrl Pts',(-2.31145225782327,-0.416497494887886,
12.1633886740147));
#23843=CARTESIAN_POINT('Origin',(0.,0.,13.5));
#23844=CARTESIAN_POINT('',(-3.1180327855299,0.795259447899244,12.3478010527258));
#23845=CARTESIAN_POINT('Ctrl Pts',(-2.31145225782327,-0.416497494887886,
12.1633886740147));
#23846=CARTESIAN_POINT('Ctrl Pts',(-2.3167521873648,-0.463716904565301,
12.1781025743524));
#23847=CARTESIAN_POINT('Ctrl Pts',(-2.32206620895333,-0.510211567222956,
12.1953357212503));
#23848=CARTESIAN_POINT('Ctrl Pts',(-2.33229991020307,-0.597693045802501,
12.233173817206));
#23849=CARTESIAN_POINT('Ctrl Pts',(-2.33720164067599,-0.638696499194981,
12.253343498657));
#23850=CARTESIAN_POINT('Ctrl Pts',(-2.35182609492161,-0.758044075161683,
12.3194871727543));
#23851=CARTESIAN_POINT('Ctrl Pts',(-2.36151340155549,-0.83297903747351,
12.371112325251));
#23852=CARTESIAN_POINT('Ctrl Pts',(-2.38103415191372,-0.97226540446231,
12.4885388985911));
#23853=CARTESIAN_POINT('Ctrl Pts',(-2.3908061863421,-1.03620742481829,12.5541523183872));
#23854=CARTESIAN_POINT('Ctrl Pts',(-2.42025680254283,-1.20796240853674,
12.7688866301326));
#23855=CARTESIAN_POINT('Ctrl Pts',(-2.43982312600438,-1.29331998098181,
12.9334109226447));
#23856=CARTESIAN_POINT('Ctrl Pts',(-2.47466620114974,-1.38409577536895,
13.2461198462985));
#23857=CARTESIAN_POINT('Ctrl Pts',(-2.48970038938532,-1.402704004665,13.3877645272084));
#23858=CARTESIAN_POINT('Ctrl Pts',(-2.51462424398795,-1.39776875624929,
13.6197852242924));
#23859=CARTESIAN_POINT('Ctrl Pts',(-2.52430994314769,-1.38717554817382,
13.7094050293777));
#23860=CARTESIAN_POINT('Ctrl Pts',(-2.54245933154651,-1.35119409578135,
13.8749286173372));
#23861=CARTESIAN_POINT('Ctrl Pts',(-2.55091248218538,-1.32777537595692,
13.9508989001517));
#23862=CARTESIAN_POINT('Ctrl Pts',(-2.56917308308684,-1.2638119902416,14.1092046896047));
#23863=CARTESIAN_POINT('Ctrl Pts',(-2.57895229850129,-1.22136348749128,
14.190378113102));
#23864=CARTESIAN_POINT('Ctrl Pts',(-2.59846139720312,-1.12161698798404,
14.3427373178754));
#23865=CARTESIAN_POINT('Ctrl Pts',(-2.6081322712015,-1.06466344008099,14.4136315100372));
#23866=CARTESIAN_POINT('Ctrl Pts',(-2.62760843372855,-0.937668490314083,
14.543577447306));
#23867=CARTESIAN_POINT('Ctrl Pts',(-2.63737030289336,-0.867893247000527,
14.6022872855144));
#23868=CARTESIAN_POINT('Ctrl Pts',(-2.65679337332192,-0.718574559597896,
14.7049015851361));
#23869=CARTESIAN_POINT('Ctrl Pts',(-2.66639112991186,-0.639466084224944,
14.7486875801947));
#23870=CARTESIAN_POINT('Ctrl Pts',(-2.68092952061222,-0.514803287617618,
14.8027134017972));
#23871=CARTESIAN_POINT('Ctrl Pts',(-2.68581920989598,-0.472048025464354,
14.8188082341359));
#23872=CARTESIAN_POINT('Ctrl Pts',(-2.70041223268387,-0.342590669370393,
14.8604378397063));
#23873=CARTESIAN_POINT('Ctrl Pts',(-2.71011363466229,-0.254121430526818,
14.8797037187546));
#23874=CARTESIAN_POINT('Ctrl Pts',(-2.7294086780924,-0.0750932251353697,
14.9008749733284));
#23875=CARTESIAN_POINT('Ctrl Pts',(-2.73898533044384,0.0150370781420963,
14.9028055849289));
#23876=CARTESIAN_POINT('Ctrl Pts',(-2.75836409190454,0.195440539002722,
14.8892725344481));
#23877=CARTESIAN_POINT('Ctrl Pts',(-2.76812368298385,0.285274149539204,
14.8736424048526));
#23878=CARTESIAN_POINT('Ctrl Pts',(-2.78762987367098,0.460540422606209,
14.8252019094676));
#23879=CARTESIAN_POINT('Ctrl Pts',(-2.79730018784044,0.545563984803865,
14.792523874345));
#23880=CARTESIAN_POINT('Ctrl Pts',(-2.81190854088784,0.667683178766226,
14.7313762949139));
#23881=CARTESIAN_POINT('Ctrl Pts',(-2.81679996050081,0.7075189164068,14.7089273179091));
#23882=CARTESIAN_POINT('Ctrl Pts',(-2.83139954255971,0.822688831613105,
14.6363795055697));
#23883=CARTESIAN_POINT('Ctrl Pts',(-2.84110944631101,0.894345491985826,
14.5808893635849));
#23884=CARTESIAN_POINT('Ctrl Pts',(-2.86039366562439,1.02543771398911,14.457353248677));
#23885=CARTESIAN_POINT('Ctrl Pts',(-2.86994280580073,1.08466095268082,14.3896956913934));
#23886=CARTESIAN_POINT('Ctrl Pts',(-2.88930432824196,1.19016061908563,14.2428448976629));
#23887=CARTESIAN_POINT('Ctrl Pts',(-2.89907467613071,1.23596830086219,14.1638393708666));
#23888=CARTESIAN_POINT('Ctrl Pts',(-2.92843101455799,1.34949690146608,13.9149187599842));
#23889=CARTESIAN_POINT('Ctrl Pts',(-2.94777333733644,1.39203401948613,13.7356737401434));
#23890=CARTESIAN_POINT('Ctrl Pts',(-2.97712004430575,1.40246577308113,13.4619756526989));
#23891=CARTESIAN_POINT('Ctrl Pts',(-2.98687033518447,1.39699251432984,13.3705080545567));
#23892=CARTESIAN_POINT('Ctrl Pts',(-3.00643901032036,1.36829687580028,13.1899756322952));
#23893=CARTESIAN_POINT('Ctrl Pts',(-3.01622731821428,1.34514862602942,13.101344544025));
#23894=CARTESIAN_POINT('Ctrl Pts',(-3.04141266551141,1.26391422487236,12.8810618542207));
#23895=CARTESIAN_POINT('Ctrl Pts',(-3.05661944091923,1.19391980854937,12.7549364988526));
#23896=CARTESIAN_POINT('Ctrl Pts',(-3.07966134533297,1.0620265877888,12.5849899766776));
#23897=CARTESIAN_POINT('Ctrl Pts',(-3.08735366480303,1.01376606064143,12.5317945273643));
#23898=CARTESIAN_POINT('Ctrl Pts',(-3.09890496797339,0.935610634270255,
12.4579271143655));
#23899=CARTESIAN_POINT('Ctrl Pts',(-3.10275037665096,0.908641978613474,
12.4343297929454));
#23900=CARTESIAN_POINT('Ctrl Pts',(-3.11040658761295,0.853109352415768,
12.3893815571006));
#23901=CARTESIAN_POINT('Ctrl Pts',(-3.11421620510946,0.824575859088257,
12.3680355398651));
#23902=CARTESIAN_POINT('Ctrl Pts',(-3.11803278657939,0.7952594475796,12.3478010540556));
#23903=CARTESIAN_POINT('',(-3.11803278688524,0.,14.9));
#23904=CARTESIAN_POINT('Origin',(-3.11803278688524,0.,13.5));
#23905=CARTESIAN_POINT('',(-2.91746474354357,0.,14.9));
#23906=CARTESIAN_POINT('',(0.,0.,14.9));
#23907=CARTESIAN_POINT('Ctrl Pts',(-2.91746474354356,8.32667268468867E-16,
14.9));
#23908=CARTESIAN_POINT('Ctrl Pts',(-2.90757293093835,-0.0924594044157247,
14.9));
#23909=CARTESIAN_POINT('Ctrl Pts',(-2.89771271548873,-0.184691566429423,
14.8908406471496));
#23910=CARTESIAN_POINT('Ctrl Pts',(-2.87788082299124,-0.366121167923027,
14.8544471970385));
#23911=CARTESIAN_POINT('Ctrl Pts',(-2.86796372368023,-0.454867233609991,
14.8272782269122));
#23912=CARTESIAN_POINT('Ctrl Pts',(-2.84124661433094,-0.684587979546175,
14.7311818185962));
#23913=CARTESIAN_POINT('Ctrl Pts',(-2.82448139317192,-0.817770227731554,
14.6470506633447));
#23914=CARTESIAN_POINT('Ctrl Pts',(-2.79449519173347,-1.02730970995846,
14.4592906694374));
#23915=CARTESIAN_POINT('Ctrl Pts',(-2.78130510865068,-1.10876333275197,
14.3638553696772));
#23916=CARTESIAN_POINT('Ctrl Pts',(-2.75555577135647,-1.23891302852057,
14.1620902827348));
#23917=CARTESIAN_POINT('Ctrl Pts',(-2.74312347368462,-1.2891672738364,14.0579558991923));
#23918=CARTESIAN_POINT('Ctrl Pts',(-2.72099075705634,-1.35502115159312,
13.8633967680281));
#23919=CARTESIAN_POINT('Ctrl Pts',(-2.71138423761646,-1.37561913391642,
13.7753415654217));
#23920=CARTESIAN_POINT('Ctrl Pts',(-2.68215668485679,-1.41198572154935,
13.5039122886093));
#23921=CARTESIAN_POINT('Ctrl Pts',(-2.66271368248315,-1.40032578005776,
13.3188842013009));
#23922=CARTESIAN_POINT('Ctrl Pts',(-2.63340568277471,-1.33032649598374,
13.0547244643092));
#23923=CARTESIAN_POINT('Ctrl Pts',(-2.6237756819577,-1.29908768118497,12.9704626653747));
#23924=CARTESIAN_POINT('Ctrl Pts',(-2.60451951442829,-1.22090765216068,
12.8090359941975));
#23925=CARTESIAN_POINT('Ctrl Pts',(-2.59497820215046,-1.17413824150344,
12.7322455266302));
#23926=CARTESIAN_POINT('Ctrl Pts',(-2.56608332448149,-1.01186755014022,
12.5157005711754));
#23927=CARTESIAN_POINT('Ctrl Pts',(-2.54672775468785,-0.876360220239523,
12.393332780747));
#23928=CARTESIAN_POINT('Ctrl Pts',(-2.51762480991736,-0.643287763981639,
12.2532148297775));
#23929=CARTESIAN_POINT('Ctrl Pts',(-2.50792686736518,-0.560851342787942,
12.2140225281083));
#23930=CARTESIAN_POINT('Ctrl Pts',(-2.49595816639203,-0.455768936955594,
12.1761037787382));
#23931=CARTESIAN_POINT('Ctrl Pts',(-2.49374542515372,-0.43619801600797,
12.169527493552));
#23932=CARTESIAN_POINT('Ctrl Pts',(-2.49153227027379,-0.416497403609637,
12.1633886455718));
#23933=CARTESIAN_POINT('Origin',(-7.25,-0.25,13.5));
#23934=CARTESIAN_POINT('',(-7.2,-0.25,14.43));
#23935=CARTESIAN_POINT('',(-7.2,-0.25,14.1858571279793));
#23936=CARTESIAN_POINT('',(-7.2,-0.25,13.5));
#23937=CARTESIAN_POINT('',(-4.4,-0.25,14.43));
#23938=CARTESIAN_POINT('',(-7.25,-0.25,14.43));
#23939=CARTESIAN_POINT('',(-4.4,-0.25,14.1538348415311));
#23940=CARTESIAN_POINT('',(-4.4,-0.25,13.5));
#23941=CARTESIAN_POINT('',(-7.17,-0.25,14.1538348415311));
#23942=CARTESIAN_POINT('',(-5.585,-0.25,14.1538348415311));
#23943=CARTESIAN_POINT('Ctrl Pts',(-7.2,-0.25,14.1858571279793));
#23944=CARTESIAN_POINT('Ctrl Pts',(-7.18464145915026,-0.25,14.1695100866453));
#23945=CARTESIAN_POINT('Ctrl Pts',(-7.17,-0.25,14.1538348415311));
#23946=CARTESIAN_POINT('Origin',(-4.4,-0.25,13.5));
#23947=CARTESIAN_POINT('',(-4.4,0.25,14.1538348415311));
#23948=CARTESIAN_POINT('Origin',(-4.4,0.,13.5));
#23949=CARTESIAN_POINT('',(-4.4,0.25,14.43));
#23950=CARTESIAN_POINT('',(-4.4,-0.25,14.43));
#23951=CARTESIAN_POINT('',(-4.4,0.25,13.5));
#23952=CARTESIAN_POINT('Origin',(-4.4,0.25,13.5));
#23953=CARTESIAN_POINT('',(-7.2,0.25,14.1858571279793));
#23954=CARTESIAN_POINT('',(-7.2,0.25,14.43));
#23955=CARTESIAN_POINT('',(-7.2,0.25,13.5));
#23956=CARTESIAN_POINT('',(-7.17,0.25,14.1538348415311));
#23957=CARTESIAN_POINT('Ctrl Pts',(-7.17,0.25,14.1538348415311));
#23958=CARTESIAN_POINT('Ctrl Pts',(-7.18464145915026,0.25,14.1695100866453));
#23959=CARTESIAN_POINT('Ctrl Pts',(-7.2,0.25,14.1858571279793));
#23960=CARTESIAN_POINT('',(-5.585,0.25,14.1538348415311));
#23961=CARTESIAN_POINT('',(-4.4,0.25,14.43));
#23962=CARTESIAN_POINT('Origin',(-5.825,0.,14.43));
#23963=CARTESIAN_POINT('',(-7.2,0.,14.43));
#23964=CARTESIAN_POINT('Origin',(-5.585,0.,13.5));
#23965=CARTESIAN_POINT('',(-4.,-8.57252759403146E-17,12.8));
#23966=CARTESIAN_POINT('Origin',(-4.,0.,13.5));
#23967=CARTESIAN_POINT('',(-7.17,-8.57252759403146E-17,12.8));
#23968=CARTESIAN_POINT('',(-5.585,-8.57252759403146E-17,12.8));
#23969=CARTESIAN_POINT('Origin',(-7.17,0.,13.5));
#23970=CARTESIAN_POINT('Origin',(-7.17,0.,13.5));
#23971=CARTESIAN_POINT('Origin',(-7.21,0.,13.5));
#23972=CARTESIAN_POINT('Origin',(-7.2,0.,13.5));
#23973=CARTESIAN_POINT('Origin',(-3.78969878334035,0.,13.5));
#23974=CARTESIAN_POINT('',(-3.57939756668071,0.,13.5));
#23975=CARTESIAN_POINT('',(-3.78969878334035,-4.28626379701574E-17,13.15));
#23976=CARTESIAN_POINT('Origin',(-3.61,0.,13.5));
#23977=CARTESIAN_POINT('',(-4.1,-1.712056225208E-16,12.102));
#23978=CARTESIAN_POINT('Origin',(-4.1,0.,13.5));
#23979=CARTESIAN_POINT('',(-3.12,-1.712056225208E-16,12.102));
#23980=CARTESIAN_POINT('',(-3.61,-1.712056225208E-16,12.102));
#23981=CARTESIAN_POINT('Origin',(-3.12,0.,13.5));
#23982=CARTESIAN_POINT('Origin',(-2.76,0.,13.5));
#23983=CARTESIAN_POINT('',(-2.9716366454152,0.,15.0488360771612));
#23984=CARTESIAN_POINT('',(-2.6276958156896,4.102857932342E-16,11.6014907459511));
#23985=CARTESIAN_POINT('Ctrl Pts',(-2.9716366454152,7.60502771868232E-15,
15.0488360771612));
#23986=CARTESIAN_POINT('Ctrl Pts',(-2.96513918497401,-0.0920375220506268,
15.0554418286098));
#23987=CARTESIAN_POINT('Ctrl Pts',(-2.95870046090467,-0.184510271773937,
15.0537810097104));
#23988=CARTESIAN_POINT('Ctrl Pts',(-2.94574540539509,-0.369537679687644,
15.0340535994561));
#23989=CARTESIAN_POINT('Ctrl Pts',(-2.93925228407338,-0.461737874031516,
15.0157596972663));
#23990=CARTESIAN_POINT('Ctrl Pts',(-2.91958652769516,-0.735865978954469,
14.9355197227161));
#23991=CARTESIAN_POINT('Ctrl Pts',(-2.90654874341827,-0.908932390668185,
14.8486604536394));
#23992=CARTESIAN_POINT('Ctrl Pts',(-2.88661663694525,-1.1476938338663,14.6696722402344));
#23993=CARTESIAN_POINT('Ctrl Pts',(-2.87963270291874,-1.22619265279611,
14.5977533374101));
#23994=CARTESIAN_POINT('Ctrl Pts',(-2.85827410403415,-1.44301835851629,
14.3568412674897));
#23995=CARTESIAN_POINT('Ctrl Pts',(-2.843906091307,-1.5556936748727,14.1673389814163));
#23996=CARTESIAN_POINT('Ctrl Pts',(-2.82263789490064,-1.66604286105911,
13.8572055037074));
#23997=CARTESIAN_POINT('Ctrl Pts',(-2.81559948523675,-1.69277726945658,
13.749379202055));
#23998=CARTESIAN_POINT('Ctrl Pts',(-2.79429900209064,-1.74166074208239,
13.417417949714));
#23999=CARTESIAN_POINT('Ctrl Pts',(-2.78031251610869,-1.73033660024184,
13.1908637168291));
#24000=CARTESIAN_POINT('Ctrl Pts',(-2.75909846476153,-1.64895833456621,
12.8603458898717));
#24001=CARTESIAN_POINT('Ctrl Pts',(-2.75193057197317,-1.61035130266583,
12.7511403637933));
#24002=CARTESIAN_POINT('Ctrl Pts',(-2.73773225640633,-1.51216303880933,
12.5414445443358));
#24003=CARTESIAN_POINT('Ctrl Pts',(-2.73072541788755,-1.45276422182245,
12.4414862625126));
#24004=CARTESIAN_POINT('Ctrl Pts',(-2.70917560177417,-1.24230101342177,
12.1543537334464));
#24005=CARTESIAN_POINT('Ctrl Pts',(-2.69478862312514,-1.06343354425305,
11.9910281778624));
#24006=CARTESIAN_POINT('Ctrl Pts',(-2.66611563845589,-0.64786062771374,
11.7400700233335));
#24007=CARTESIAN_POINT('Ctrl Pts',(-2.65185433641513,-0.415477599079208,
11.6563602555503));
#24008=CARTESIAN_POINT('Ctrl Pts',(-2.63435622392806,-0.115608928180287,
11.610909632013));
#24009=CARTESIAN_POINT('Ctrl Pts',(-2.63102379259863,-0.057881494981571,
11.6048741891419));
#24010=CARTESIAN_POINT('Ctrl Pts',(-2.6276958156896,-4.16333634234434E-17,
11.6014907459511));
#24011=CARTESIAN_POINT('',(-2.76,0.,15.264));
#24012=CARTESIAN_POINT('',(-2.42954235284503,-0.728141132413258,15.4696174511348));
#24013=CARTESIAN_POINT('Ctrl Pts',(-2.42950897630267,-0.72814559274872,
15.4695817140195));
#24014=CARTESIAN_POINT('Ctrl Pts',(-2.43828133387365,-0.652393922688123,
15.4881130997835));
#24015=CARTESIAN_POINT('Ctrl Pts',(-2.44710731128846,-0.575762085981697,
15.5023539166817));
#24016=CARTESIAN_POINT('Ctrl Pts',(-2.45598857155625,-0.498622745157995,
15.5122142918554));
#24017=CARTESIAN_POINT('Ctrl Pts',(-2.46354562505042,-0.432984974443784,
15.5206044730249));
#24018=CARTESIAN_POINT('Ctrl Pts',(-2.47114270491829,-0.36697910323544,
15.5258224467513));
#24019=CARTESIAN_POINT('Ctrl Pts',(-2.47878083569838,-0.300830869104269,
15.5277833167051));
#24020=CARTESIAN_POINT('Ctrl Pts',(-2.48542346325084,-0.243303956403079,
15.5294886198948));
#24021=CARTESIAN_POINT('Ctrl Pts',(-2.49209713843209,-0.185669120678873,
15.5287299263396));
#24022=CARTESIAN_POINT('Ctrl Pts',(-2.49880253512854,-0.128089393860388,
15.5255228966375));
#24023=CARTESIAN_POINT('Ctrl Pts',(-2.5072738296511,-0.0553457745803134,
15.521471280547));
#24024=CARTESIAN_POINT('Ctrl Pts',(-2.51578575259894,0.0170141412883056,
15.5134623775051));
#24025=CARTESIAN_POINT('Ctrl Pts',(-2.52435299120783,0.0886762807947775,
15.5015542669419));
#24026=CARTESIAN_POINT('Ctrl Pts',(-2.53280268327874,0.159355182085626,
15.4898095412493));
#24027=CARTESIAN_POINT('Ctrl Pts',(-2.54130618351024,0.229356191559046,
15.4742714490102));
#24028=CARTESIAN_POINT('Ctrl Pts',(-2.54987758284735,0.298357125319829,
15.454950376115));
#24029=CARTESIAN_POINT('Ctrl Pts',(-2.55591084252828,0.346925688658546,
15.44135060722));
#24030=CARTESIAN_POINT('Ctrl Pts',(-2.56197774287886,0.394998346664019,
15.4258756141398));
#24031=CARTESIAN_POINT('Ctrl Pts',(-2.56808319796508,0.442452970992676,
15.4085168966114));
#24032=CARTESIAN_POINT('Ctrl Pts',(-2.57337296203872,0.483567640310015,
15.3934773100368));
#24033=CARTESIAN_POINT('Ctrl Pts',(-2.57866827746268,0.52409371908305,15.3770890380495));
#24034=CARTESIAN_POINT('Ctrl Pts',(-2.58397493596881,0.563963099394563,
15.3593573159425));
#24035=CARTESIAN_POINT('Ctrl Pts',(-2.5923929959919,0.627208706052391,15.3312291255121));
#24036=CARTESIAN_POINT('Ctrl Pts',(-2.60083959988352,0.688803992220178,
15.2997217492959));
#24037=CARTESIAN_POINT('Ctrl Pts',(-2.60933786728269,0.748496053253066,
15.2649883767521));
#24038=CARTESIAN_POINT('Ctrl Pts',(-2.61771331374979,0.807325416723062,
15.2307569871407));
#24039=CARTESIAN_POINT('Ctrl Pts',(-2.62613894118528,0.864306631227038,
15.193391324339));
#24040=CARTESIAN_POINT('Ctrl Pts',(-2.63463688123865,0.91915493949617,15.1530124968274));
#24041=CARTESIAN_POINT('Ctrl Pts',(-2.6430080517745,0.973185038466007,15.1132360275873));
#24042=CARTESIAN_POINT('Ctrl Pts',(-2.65144939354802,1.0251457497766,15.0705348700075));
#24043=CARTESIAN_POINT('Ctrl Pts',(-2.65998206245267,1.07471716779012,15.0250116008781));
#24044=CARTESIAN_POINT('Ctrl Pts',(-2.66856889690476,1.12460326612508,14.9791993491548));
#24045=CARTESIAN_POINT('Ctrl Pts',(-2.67717652916123,1.17184634124863,14.930832044474));
#24046=CARTESIAN_POINT('Ctrl Pts',(-2.68582721608512,1.21619181790131,14.880055106104));
#24047=CARTESIAN_POINT('Ctrl Pts',(-2.68693017405182,1.22184584251129,14.873581073557));
#24048=CARTESIAN_POINT('Ctrl Pts',(-2.68803383192009,1.22745270054738,14.8670678400251));
#24049=CARTESIAN_POINT('Ctrl Pts',(-2.68913823582054,1.23301180794913,14.8605156828892));
#24050=CARTESIAN_POINT('Ctrl Pts',(-2.69780686600573,1.27664606730464,14.8090868287324));
#24051=CARTESIAN_POINT('Ctrl Pts',(-2.7065214585854,1.317342655988,14.7552605774778));
#24052=CARTESIAN_POINT('Ctrl Pts',(-2.71530432135743,1.35491020711387,14.6992948620781));
#24053=CARTESIAN_POINT('Ctrl Pts',(-2.723931202225,1.39181056596746,14.6443230867067));
#24054=CARTESIAN_POINT('Ctrl Pts',(-2.73262394988786,1.42569206891259,14.587286214873));
#24055=CARTESIAN_POINT('Ctrl Pts',(-2.74140370458174,1.45632354330652,14.5284296470777));
#24056=CARTESIAN_POINT('Ctrl Pts',(-2.74485822024362,1.46837591968032,14.5052717181443));
#24057=CARTESIAN_POINT('Ctrl Pts',(-2.74832620579143,1.47992459466916,14.4818321617964));
#24058=CARTESIAN_POINT('Ctrl Pts',(-2.75180894895332,1.49095330984029,14.4581264477211));
#24059=CARTESIAN_POINT('Ctrl Pts',(-2.76059084527361,1.51876272003126,14.3983514044491));
#24060=CARTESIAN_POINT('Ctrl Pts',(-2.76941014808247,1.5431441216538,14.3372177086219));
#24061=CARTESIAN_POINT('Ctrl Pts',(-2.77828383165334,1.56394559838933,14.2749870597415));
#24062=CARTESIAN_POINT('Ctrl Pts',(-2.78361136491003,1.57643427439537,14.2376253655986));
#24063=CARTESIAN_POINT('Ctrl Pts',(-2.78895849968681,1.58763161386914,14.199868008425));
#24064=CARTESIAN_POINT('Ctrl Pts',(-2.79432890929644,1.5974957180488,14.1617708044219));
#24065=CARTESIAN_POINT('Ctrl Pts',(-2.7995038989002,1.60700088437512,14.1250598924099));
#24066=CARTESIAN_POINT('Ctrl Pts',(-2.80470050031048,1.6152878476834,14.0880410272743));
#24067=CARTESIAN_POINT('Ctrl Pts',(-2.8099220002496,1.62232851562243,14.0507753415377));
#24068=CARTESIAN_POINT('Ctrl Pts',(-2.81057126118396,1.62320397874565,14.0461415860608));
#24069=CARTESIAN_POINT('Ctrl Pts',(-2.81122090708287,1.6240601616151,14.0415040152221));
#24070=CARTESIAN_POINT('Ctrl Pts',(-2.81187094425713,1.62489704744289,14.0368627492777));
#24071=CARTESIAN_POINT('Ctrl Pts',(-2.81381623018475,1.62740149224743,14.0229734061976));
#24072=CARTESIAN_POINT('Ctrl Pts',(-2.81576502021133,1.62973313669868,14.009050970835));
#24073=CARTESIAN_POINT('Ctrl Pts',(-2.81771748379929,1.6318903765127,13.9950985850967));
#24074=CARTESIAN_POINT('Ctrl Pts',(-2.82545005793353,1.64043395032895,13.9398412897819));
#24075=CARTESIAN_POINT('Ctrl Pts',(-2.833240250158,1.64624395051514,13.8841130893233));
#24076=CARTESIAN_POINT('Ctrl Pts',(-2.84109858067896,1.64923640968078,13.8281266562807));
#24077=CARTESIAN_POINT('Ctrl Pts',(-2.84193367124711,1.64955441290273,13.8221770793249));
#24078=CARTESIAN_POINT('Ctrl Pts',(-2.84276953130881,1.64984057390514,13.8162246004353));
#24079=CARTESIAN_POINT('Ctrl Pts',(-2.84360617348995,1.65009480603853,13.8102694912202));
#24080=CARTESIAN_POINT('Ctrl Pts',(-2.85053440500889,1.65220010161102,13.7609552487722));
#24081=CARTESIAN_POINT('Ctrl Pts',(-2.85748562231733,1.65210954291448,13.711675457902));
#24082=CARTESIAN_POINT('Ctrl Pts',(-2.86446969399717,1.64981830164746,13.6625695815424));
#24083=CARTESIAN_POINT('Ctrl Pts',(-2.87221299374171,1.64727798294357,13.6081254782596));
#24084=CARTESIAN_POINT('Ctrl Pts',(-2.87999667721129,1.6420328224924,13.553894471909));
#24085=CARTESIAN_POINT('Ctrl Pts',(-2.88783420560974,1.63407416166227,13.5000808184616));
#24086=CARTESIAN_POINT('Ctrl Pts',(-2.89669160433426,1.6250798679638,13.4392645813553));
#24087=CARTESIAN_POINT('Ctrl Pts',(-2.90561777488003,1.61258123845351,13.3789842494571));
#24088=CARTESIAN_POINT('Ctrl Pts',(-2.91463213809415,1.59662058112076,13.3195527785932));
#24089=CARTESIAN_POINT('Ctrl Pts',(-2.92143823922656,1.58456982996219,13.2746803243179));
#24090=CARTESIAN_POINT('Ctrl Pts',(-2.92829461609412,1.57054460426979,13.2302923047606));
#24091=CARTESIAN_POINT('Ctrl Pts',(-2.93520962564436,1.5545508931325,13.1865389682066));
#24092=CARTESIAN_POINT('Ctrl Pts',(-2.94421617859849,1.5337196556274,13.1295518100935));
#24093=CARTESIAN_POINT('Ctrl Pts',(-2.95327041031035,1.50967160688709,13.0739612407976));
#24094=CARTESIAN_POINT('Ctrl Pts',(-2.96239011792779,1.48249585547248,13.0200487040156));
#24095=CARTESIAN_POINT('Ctrl Pts',(-2.96867214801171,1.46377607901678,12.9829115289907));
#24096=CARTESIAN_POINT('Ctrl Pts',(-2.97498524643709,1.44357121811679,12.9465710635193));
#24097=CARTESIAN_POINT('Ctrl Pts',(-2.98133522842137,1.42189964112574,12.9111289027924));
#24098=CARTESIAN_POINT('Ctrl Pts',(-2.98521698496443,1.40865176325903,12.8894630398588));
#24099=CARTESIAN_POINT('Ctrl Pts',(-2.98911252429411,1.39487333007331,12.8681244140488));
#24100=CARTESIAN_POINT('Ctrl Pts',(-2.99302318265689,1.38055563147682,12.8471482007924));
#24101=CARTESIAN_POINT('Ctrl Pts',(-3.00222557049681,1.34686385806242,12.7977879059544));
#24102=CARTESIAN_POINT('Ctrl Pts',(-3.01151167911897,1.31018675736906,12.7504310994907));
#24103=CARTESIAN_POINT('Ctrl Pts',(-3.02089883194599,1.2707144390074,12.7053595163719));
#24104=CARTESIAN_POINT('Ctrl Pts',(-3.02282748276932,1.26260459774779,12.696099270215));
#24105=CARTESIAN_POINT('Ctrl Pts',(-3.02476039888356,1.2543767198893,12.6869356583494));
#24106=CARTESIAN_POINT('Ctrl Pts',(-3.02669773049638,1.24603239893449,12.6778713956583));
#24107=CARTESIAN_POINT('Ctrl Pts',(-3.03587169974251,1.20651900674461,12.634948817708));
#24108=CARTESIAN_POINT('Ctrl Pts',(-3.04510691998591,1.16459151076389,12.5945250929969));
#24109=CARTESIAN_POINT('Ctrl Pts',(-3.05442054614937,1.1204751933185,12.5568057770798));
#24110=CARTESIAN_POINT('Ctrl Pts',(-3.06357860128224,1.07709577693082,12.5197165093038));
#24111=CARTESIAN_POINT('Ctrl Pts',(-3.07281246497777,1.03159910549671,12.485241612509));
#24112=CARTESIAN_POINT('Ctrl Pts',(-3.08213843971222,0.984178358509514,
12.45362145311));
#24113=CARTESIAN_POINT('Ctrl Pts',(-3.08746848512046,0.957076126096147,
12.4355496815032));
#24114=CARTESIAN_POINT('Ctrl Pts',(-3.09282861781865,0.929345098676938,
12.4184112541742));
#24115=CARTESIAN_POINT('Ctrl Pts',(-3.09822187997365,0.901019921332647,
12.4022586271553));
#24116=CARTESIAN_POINT('Ctrl Pts',(-3.10477478547288,0.866604347779572,
12.3826329098479));
#24117=CARTESIAN_POINT('Ctrl Pts',(-3.11137659861426,0.831311551242717,
12.3644620673644));
#24118=CARTESIAN_POINT('Ctrl Pts',(-3.11803278626624,0.795259448582878,
12.3478010539834));
#24119=CARTESIAN_POINT('',(-2.42950819541372,2.0402249837135,13.997475649067));
#24120=CARTESIAN_POINT('Ctrl Pts',(-2.42950819541372,2.0402249837135,13.997475649067));
#24121=CARTESIAN_POINT('Ctrl Pts',(-2.42950819680997,2.03104070784062,14.0351417863892));
#24122=CARTESIAN_POINT('Ctrl Pts',(-2.4295078943495,2.02082185143214,14.0725200484997));
#24123=CARTESIAN_POINT('Ctrl Pts',(-2.4295077739925,2.00958407097205,14.1095684266328));
#24124=CARTESIAN_POINT('Ctrl Pts',(-2.42950772057022,2.0045960122126,14.1260129093958));
#24125=CARTESIAN_POINT('Ctrl Pts',(-2.42950772487925,1.99940718549468,14.1423924033825));
#24126=CARTESIAN_POINT('Ctrl Pts',(-2.42950770490987,1.99401905946343,14.1587033403071));
#24127=CARTESIAN_POINT('Ctrl Pts',(-2.42950769825192,1.99222261438882,14.164141539438));
#24128=CARTESIAN_POINT('Ctrl Pts',(-2.42950768941003,1.99040401448508,14.1695721175525));
#24129=CARTESIAN_POINT('Ctrl Pts',(-2.42950768353223,1.98856330462253,14.1749949442969));
#24130=CARTESIAN_POINT('Ctrl Pts',(-2.42950763650018,1.97383462039571,14.2183864120994));
#24131=CARTESIAN_POINT('Ctrl Pts',(-2.42950748653377,1.95769054165353,14.2612816804408));
#24132=CARTESIAN_POINT('Ctrl Pts',(-2.42950667483392,1.94015919913297,14.3036098434447));
#24133=CARTESIAN_POINT('Ctrl Pts',(-2.42950537091809,1.91199682484255,14.3716058664614));
#24134=CARTESIAN_POINT('Ctrl Pts',(-2.42953396383665,1.88022422208483,14.4381290972791));
#24135=CARTESIAN_POINT('Ctrl Pts',(-2.42955788537467,1.84497965647924,14.5029147018465));
#24136=CARTESIAN_POINT('Ctrl Pts',(-2.42958299061506,1.80799109448428,14.5709060732749));
#24137=CARTESIAN_POINT('Ctrl Pts',(-2.42960241503354,1.76731073394805,14.6367401361202));
#24138=CARTESIAN_POINT('Ctrl Pts',(-2.42960150222464,1.72316139552393,14.7001318258739));
#24139=CARTESIAN_POINT('Ctrl Pts',(-2.42960058952012,1.67901710536999,14.7635162670846));
#24140=CARTESIAN_POINT('Ctrl Pts',(-2.42957934719993,1.63140464193822,14.8244588516644));
#24141=CARTESIAN_POINT('Ctrl Pts',(-2.42955053246563,1.58052679997558,14.8826620204458));
#24142=CARTESIAN_POINT('Ctrl Pts',(-2.42954063326503,1.56304789635725,14.9026575143223));
#24143=CARTESIAN_POINT('Ctrl Pts',(-2.42953007693327,1.54518342161295,14.9223295821176));
#24144=CARTESIAN_POINT('Ctrl Pts',(-2.42952011418379,1.52694101005491,14.9416657949728));
#24145=CARTESIAN_POINT('Ctrl Pts',(-2.42949966636738,1.48949979133883,14.9813519610452));
#24146=CARTESIAN_POINT('Ctrl Pts',(-2.42948144177566,1.45058462751578,15.0194988701834));
#24147=CARTESIAN_POINT('Ctrl Pts',(-2.42948064766016,1.41028422127532,15.0560257229549));
#24148=CARTESIAN_POINT('Ctrl Pts',(-2.42947952101429,1.35310829921469,15.1078479421833));
#24149=CARTESIAN_POINT('Ctrl Pts',(-2.42951234976274,1.293143106258,15.1564118688575));
#24150=CARTESIAN_POINT('Ctrl Pts',(-2.42953875010086,1.23069375916773,15.2015470634631));
#24151=CARTESIAN_POINT('Ctrl Pts',(-2.42956521275925,1.16809699500034,15.2467888035935));
#24152=CARTESIAN_POINT('Ctrl Pts',(-2.42958504927452,1.10300405208996,15.2885852272081));
#24153=CARTESIAN_POINT('Ctrl Pts',(-2.42958398637795,1.03571625753847,15.3267370412771));
#24154=CARTESIAN_POINT('Ctrl Pts',(-2.42958311156895,0.980335546350388,
15.3581376037467));
#24155=CARTESIAN_POINT('Ctrl Pts',(-2.42956855809535,0.923467978597577,
15.3870688303849));
#24156=CARTESIAN_POINT('Ctrl Pts',(-2.42954659138197,0.865279467155291,
15.4134073011364));
#24157=CARTESIAN_POINT('Ctrl Pts',(-2.42951986269709,0.794476777723754,
15.4454554583842));
#24158=CARTESIAN_POINT('Ctrl Pts',(-2.42948178901242,0.722099894650869,
15.4734932183326));
#24159=CARTESIAN_POINT('Ctrl Pts',(-2.42946854755221,0.648485392194134,
15.4974073194238));
#24160=CARTESIAN_POINT('Ctrl Pts',(-2.42946622137184,0.635553237597292,
15.5016084053788));
#24161=CARTESIAN_POINT('Ctrl Pts',(-2.42946472289851,0.62258280157832,15.5056821886663));
#24162=CARTESIAN_POINT('Ctrl Pts',(-2.42946432430103,0.609575796683492,
15.5096279967501));
#24163=CARTESIAN_POINT('Ctrl Pts',(-2.42946205900156,0.53565470480022,15.5320527166816));
#24164=CARTESIAN_POINT('Ctrl Pts',(-2.42949335707758,0.460551672769708,
15.5503467455696));
#24165=CARTESIAN_POINT('Ctrl Pts',(-2.42951843576671,0.38461200192984,15.5644684273091));
#24166=CARTESIAN_POINT('Ctrl Pts',(-2.42954349448136,0.308732814924717,
15.578578861522));
#24167=CARTESIAN_POINT('Ctrl Pts',(-2.42956216754896,0.232018215097528,
15.5885231154159));
#24168=CARTESIAN_POINT('Ctrl Pts',(-2.42956073494453,0.154822861515672,
15.5942314929807));
#24169=CARTESIAN_POINT('Ctrl Pts',(-2.42956023651616,0.127965235290666,
15.5962175383043));
#24170=CARTESIAN_POINT('Ctrl Pts',(-2.4295575461063,0.101049510913713,15.5976906247383));
#24171=CARTESIAN_POINT('Ctrl Pts',(-2.4295528717745,0.074090926958688,15.5986471294928));
#24172=CARTESIAN_POINT('Ctrl Pts',(-2.42953939803581,-0.00361706023941163,
15.6014042497977));
#24173=CARTESIAN_POINT('Ctrl Pts',(-2.42950755976971,-0.0812632159739146,
15.5998562556563));
#24174=CARTESIAN_POINT('Ctrl Pts',(-2.42948139432591,-0.158486510405496,
15.5940383169824));
#24175=CARTESIAN_POINT('Ctrl Pts',(-2.42946441726226,-0.208591710033162,
15.590263432981));
#24176=CARTESIAN_POINT('Ctrl Pts',(-2.42945039794091,-0.258519331802215,
15.5846905206051));
#24177=CARTESIAN_POINT('Ctrl Pts',(-2.42945157053088,-0.308175379396695,
15.5773227319512));
#24178=CARTESIAN_POINT('Ctrl Pts',(-2.42945337836478,-0.384732307896107,
15.5659634857667));
#24179=CARTESIAN_POINT('Ctrl Pts',(-2.42949008892026,-0.460646632046284,
15.5503387762186));
#24180=CARTESIAN_POINT('Ctrl Pts',(-2.42952017157432,-0.535581221553956,
15.5305421991785));
#24181=CARTESIAN_POINT('Ctrl Pts',(-2.42954627109418,-0.600593996101206,
15.513366814508));
#24182=CARTESIAN_POINT('Ctrl Pts',(-2.42956765411205,-0.664868833921869,
15.4930505486365));
#24183=CARTESIAN_POINT('Ctrl Pts',(-2.42957323886436,-0.728169658321024,
15.4696424099624));
#24184=CARTESIAN_POINT('Ctrl Pts',(-2.6276958156896,1.52655665885959E-16,
11.6014907459511));
#24185=CARTESIAN_POINT('Ctrl Pts',(-2.62394006512444,0.0653215041544882,
11.5976723995432));
#24186=CARTESIAN_POINT('Ctrl Pts',(-2.62018977471018,0.130839214337266,
11.5972317286682));
#24187=CARTESIAN_POINT('Ctrl Pts',(-2.60924600079219,0.321708528580622,
11.605764455657));
#24188=CARTESIAN_POINT('Ctrl Pts',(-2.60206759657853,0.446362335031581,
11.6237172245559));
#24189=CARTESIAN_POINT('Ctrl Pts',(-2.58787639794491,0.689733221082812,
11.6835386074477));
#24190=CARTESIAN_POINT('Ctrl Pts',(-2.58088693136192,0.807990259168507,
11.7251684660431));
#24191=CARTESIAN_POINT('Ctrl Pts',(-2.566729012865,1.0376094825962,11.8316904957494));
#24192=CARTESIAN_POINT('Ctrl Pts',(-2.55958384779881,1.14832818180093,11.8969492545597));
#24193=CARTESIAN_POINT('Ctrl Pts',(-2.5454256196204,1.35516943309115,12.0478477449589));
#24194=CARTESIAN_POINT('Ctrl Pts',(-2.53844069958128,1.45094868699436,12.1331852719129));
#24195=CARTESIAN_POINT('Ctrl Pts',(-2.51696790688888,1.71765987875923,12.4211611768747));
#24196=CARTESIAN_POINT('Ctrl Pts',(-2.50269556727083,1.85703571789682,12.6487824541898));
#24197=CARTESIAN_POINT('Ctrl Pts',(-2.48361000855449,1.98085492461562,12.983639184611));
#24198=CARTESIAN_POINT('Ctrl Pts',(-2.47872042512685,2.00684884077783,13.071830082245));
#24199=CARTESIAN_POINT('Ctrl Pts',(-2.46638211843693,2.05734586452424,13.2980002064133));
#24200=CARTESIAN_POINT('Ctrl Pts',(-2.45897955765079,2.07380945906283,13.4372088906499));
#24201=CARTESIAN_POINT('Ctrl Pts',(-2.44419130460703,2.07839281191841,13.7182033191773));
#24202=CARTESIAN_POINT('Ctrl Pts',(-2.43683437473473,2.06633102056939,13.8589688601983));
#24203=CARTESIAN_POINT('Ctrl Pts',(-2.42949658771307,2.0402367405008,13.9974772490428));
#24204=CARTESIAN_POINT('',(-2.76,2.16027695369593E-16,11.736));
#24205=CARTESIAN_POINT('Origin',(2.76,0.,13.5));
#24206=CARTESIAN_POINT('',(2.42946620026141,0.728215466689312,15.4697414959281));
#24207=CARTESIAN_POINT('Ctrl Pts',(2.4295428593244,0.728207872842018,15.4696612109339));
#24208=CARTESIAN_POINT('Ctrl Pts',(2.45091245476581,0.544260182117664,15.5145058956143));
#24209=CARTESIAN_POINT('Ctrl Pts',(2.47243403011723,0.353895986727487,15.5344506012717));
#24210=CARTESIAN_POINT('Ctrl Pts',(2.51574798427622,-0.0184887986635827,
15.5203893841951));
#24211=CARTESIAN_POINT('Ctrl Pts',(2.53729267461328,-0.198366817608611,
15.4886959758906));
#24212=CARTESIAN_POINT('Ctrl Pts',(2.57335815717529,-0.484693670484068,
15.396371826893));
#24213=CARTESIAN_POINT('Ctrl Pts',(2.58772300656413,-0.594462359872026,
15.3495656517267));
#24214=CARTESIAN_POINT('Ctrl Pts',(2.61758761270735,-0.808160240452916,
15.2336270291036));
#24215=CARTESIAN_POINT('Ctrl Pts',(2.63300531424843,-0.910881098739636,
15.1641102349212));
#24216=CARTESIAN_POINT('Ctrl Pts',(2.67898127911371,-1.19167129608836,14.9304922263634));
#24217=CARTESIAN_POINT('Ctrl Pts',(2.70945231761375,-1.34589255217788,14.7416369283767));
#24218=CARTESIAN_POINT('Ctrl Pts',(2.75688651831879,-1.51006470327172,14.4249429786798));
#24219=CARTESIAN_POINT('Ctrl Pts',(2.77232144014209,-1.55283890794701,14.3180479678811));
#24220=CARTESIAN_POINT('Ctrl Pts',(2.80297552759952,-1.61574634612789,14.1008746920454));
#24221=CARTESIAN_POINT('Ctrl Pts',(2.81822477516551,-1.636289288732,13.99103340657));
#24222=CARTESIAN_POINT('Ctrl Pts',(2.86341962914337,-1.66363957104621,13.6682439161839));
#24223=CARTESIAN_POINT('Ctrl Pts',(2.8936148904857,-1.64104738498822,13.4542373098146));
#24224=CARTESIAN_POINT('Ctrl Pts',(2.95523022888075,-1.5150429038044,13.0571671419898));
#24225=CARTESIAN_POINT('Ctrl Pts',(2.98583545551893,-1.41570656735004,12.8748297123451));
#24226=CARTESIAN_POINT('Ctrl Pts',(3.0341141182629,-1.21525684562294,12.6397726471057));
#24227=CARTESIAN_POINT('Ctrl Pts',(3.05076154939996,-1.13920589486915,12.5677922695722));
#24228=CARTESIAN_POINT('Ctrl Pts',(3.07606134278261,-1.01540336829484,12.4739551790739));
#24229=CARTESIAN_POINT('Ctrl Pts',(3.08439653127644,-0.973317553865625,
12.4454466927866));
#24230=CARTESIAN_POINT('Ctrl Pts',(3.10110102258154,-0.886501873825729,
12.3931612938824));
#24231=CARTESIAN_POINT('Ctrl Pts',(3.10951634275777,-0.841391123218596,
12.3691213536139));
#24232=CARTESIAN_POINT('Ctrl Pts',(3.11803278688524,-0.79526461825914,12.3478046229284));
#24233=CARTESIAN_POINT('',(2.42950897538817,-2.04022719656258,13.9974632264163));
#24234=CARTESIAN_POINT('Ctrl Pts',(2.42950897535609,-2.04022719645617,13.9974632268527));
#24235=CARTESIAN_POINT('Ctrl Pts',(2.42950872897253,-2.00274565249741,14.1511859288549));
#24236=CARTESIAN_POINT('Ctrl Pts',(2.42930928961135,-1.94798539314298,14.3007710907449));
#24237=CARTESIAN_POINT('Ctrl Pts',(2.42923224593775,-1.80707757751576,14.5816641247516));
#24238=CARTESIAN_POINT('Ctrl Pts',(2.42952850076456,-1.72154152557879,14.7125426586374));
#24239=CARTESIAN_POINT('Ctrl Pts',(2.42971570504825,-1.50237106737774,14.9792353537282));
#24240=CARTESIAN_POINT('Ctrl Pts',(2.42911821842147,-1.30001519781745,15.1877063217083));
#24241=CARTESIAN_POINT('Ctrl Pts',(2.42962442410881,-0.773863563946308,
15.4667317038028));
#24242=CARTESIAN_POINT('Ctrl Pts',(2.42929816410876,-0.508411158962302,
15.5612192539789));
#24243=CARTESIAN_POINT('Ctrl Pts',(2.42960691697754,-0.0439201933795526,
15.6052575674409));
#24244=CARTESIAN_POINT('Ctrl Pts',(2.42973955557419,0.113432076793043,15.6025240418254));
#24245=CARTESIAN_POINT('Ctrl Pts',(2.42959753284754,0.425077640835638,15.5624814344048));
#24246=CARTESIAN_POINT('Ctrl Pts',(2.42940744355207,0.579271575329576,15.5248698940994));
#24247=CARTESIAN_POINT('Ctrl Pts',(2.42946620026141,0.728215466689312,15.4697414959281));
#24248=CARTESIAN_POINT('',(2.62767578687551,5.23812981406848E-11,11.6014703833234));
#24249=CARTESIAN_POINT('Ctrl Pts',(2.62767578687551,5.23796561680001E-11,
11.6014703833234));
#24250=CARTESIAN_POINT('Ctrl Pts',(2.62098011477951,-0.116414384474613,
11.5946631166893));
#24251=CARTESIAN_POINT('Ctrl Pts',(2.61433244389839,-0.233246843799019,
11.5986165460831));
#24252=CARTESIAN_POINT('Ctrl Pts',(2.60094196653965,-0.466404619323598,
11.6278926160068));
#24253=CARTESIAN_POINT('Ctrl Pts',(2.59422809304221,-0.582218819371836,
11.6534619509933));
#24254=CARTESIAN_POINT('Ctrl Pts',(2.57394533253695,-0.924654145743048,
11.7628407986736));
#24255=CARTESIAN_POINT('Ctrl Pts',(2.56048209332691,-1.13879792156818,11.8782924728836));
#24256=CARTESIAN_POINT('Ctrl Pts',(2.54018166141812,-1.42710311554983,12.1107845923993));
#24257=CARTESIAN_POINT('Ctrl Pts',(2.53322887545074,-1.51904167092177,12.201074994458));
#24258=CARTESIAN_POINT('Ctrl Pts',(2.5116856423392,-1.77388914413096,12.5045620247723));
#24259=CARTESIAN_POINT('Ctrl Pts',(2.4970626279049,-1.90362480482177,12.7420350185755));
#24260=CARTESIAN_POINT('Ctrl Pts',(2.4737929908366,-2.0331806915867,13.1580907394865));
#24261=CARTESIAN_POINT('Ctrl Pts',(2.46501245235341,-2.06306535902456,13.3231803556173));
#24262=CARTESIAN_POINT('Ctrl Pts',(2.45173509424097,-2.07779160731285,13.5745989517968));
#24263=CARTESIAN_POINT('Ctrl Pts',(2.44727333901277,-2.07755004137547,13.6595228653821));
#24264=CARTESIAN_POINT('Ctrl Pts',(2.43837136332853,-2.06665570422367,13.8292367080807));
#24265=CARTESIAN_POINT('Ctrl Pts',(2.43393725252676,-2.0559925643255,13.9138000778369));
#24266=CARTESIAN_POINT('Ctrl Pts',(2.42950458733698,-2.04023164095418,13.9974638311817));
#24267=CARTESIAN_POINT('',(2.76,1.76862604618026E-11,11.736));
#24268=CARTESIAN_POINT('',(3.12,-1.712056225208E-16,12.102));
#24269=CARTESIAN_POINT('',(2.76,-2.16027695369593E-16,11.736));
#24270=CARTESIAN_POINT('Origin',(3.12,0.,13.5));
#24271=CARTESIAN_POINT('Origin',(3.61,0.,13.5));
#24272=CARTESIAN_POINT('',(4.1,-1.712056225208E-16,12.102));
#24273=CARTESIAN_POINT('',(3.61,-1.712056225208E-16,12.102));
#24274=CARTESIAN_POINT('Origin',(4.1,0.,13.5));
#24275=CARTESIAN_POINT('Ctrl Pts',(-2.4295462516368,2.04037572573852,13.9968570253301));
#24276=CARTESIAN_POINT('Ctrl Pts',(-2.42676399539611,2.03115983127861,14.0347026749067));
#24277=CARTESIAN_POINT('Ctrl Pts',(-2.42275455106802,2.0163620858964,14.0888717436244));
#24278=CARTESIAN_POINT('Ctrl Pts',(-2.41833606520329,1.99767985787329,14.1478468672687));
#24279=CARTESIAN_POINT('Ctrl Pts',(-2.41342732442686,1.97585722502828,14.2130128614707));
#24280=CARTESIAN_POINT('Ctrl Pts',(-2.40974577055595,1.95769272238393,14.261277921562));
#24281=CARTESIAN_POINT('Ctrl Pts',(-2.38438395519232,1.82183653240103,14.5893116957435));
#24282=CARTESIAN_POINT('Ctrl Pts',(-2.34020530861667,1.45696855344266,15.1074622666804));
#24283=CARTESIAN_POINT('Ctrl Pts',(-2.2739373382268,0.62977347580106,15.5760953406599));
#24284=CARTESIAN_POINT('Ctrl Pts',(-2.20766936827494,-0.31829920263192,
15.6461013495652));
#24285=CARTESIAN_POINT('Ctrl Pts',(-2.14385576769032,-1.17248093264124,
15.3164944266901));
#24286=CARTESIAN_POINT('Ctrl Pts',(-2.08249653614418,-1.79133169412791,
14.6971225551438));
#24287=CARTESIAN_POINT('Ctrl Pts',(-2.01868293537138,-2.14067149238402,
13.8556172017264));
#24288=CARTESIAN_POINT('Ctrl Pts',(-1.95977807328636,-2.0990703334386,13.0070783687417));
#24289=CARTESIAN_POINT('Ctrl Pts',(-1.9131450572471,-1.81590690250113,12.410569648822));
#24290=CARTESIAN_POINT('Ctrl Pts',(-1.88860136456768,-1.60407022565932,
12.138968949739));
#24291=CARTESIAN_POINT('Ctrl Pts',(-1.87878388758855,-1.50925008150214,
12.0393936930147));
#24292=CARTESIAN_POINT('Ctrl Pts',(-1.8714207797393,-1.43636217244859,11.9664998633223));
#24293=CARTESIAN_POINT('Ctrl Pts',(-1.8566945641682,-1.28341706100303,11.8279079030736));
#24294=CARTESIAN_POINT('Ctrl Pts',(-1.82233339458021,-0.881586233572867,
11.5590960177494));
#24295=CARTESIAN_POINT('Ctrl Pts',(-1.77324600952379,-0.211348166169894,
11.355717775956));
#24296=CARTESIAN_POINT('Ctrl Pts',(-1.70943240871259,0.695366325214471,
11.444765962131));
#24297=CARTESIAN_POINT('Ctrl Pts',(-1.66525376189339,1.24201258995575,11.7719946812417));
#24298=CARTESIAN_POINT('Ctrl Pts',(-1.62352948442918,1.65511419058129,12.1850871361999));
#24299=CARTESIAN_POINT('Ctrl Pts',(-1.58916831486898,1.93554864063555,12.5840848980242));
#24300=CARTESIAN_POINT('Ctrl Pts',(-1.52535471408587,2.17939055703516,13.4583963500157));
#24301=CARTESIAN_POINT('Ctrl Pts',(-1.46154111311181,1.99758949424158,14.3723763583426));
#24302=CARTESIAN_POINT('Ctrl Pts',(-1.3977275123059,1.43775329796456,15.0868868062281));
#24303=CARTESIAN_POINT('Ctrl Pts',(-1.36336634275071,1.02596017097957,15.3480904456428));
#24304=CARTESIAN_POINT('Ctrl Pts',(-1.31673332685749,0.422785352598646,
15.5985301254968));
#24305=CARTESIAN_POINT('Ctrl Pts',(-1.27255468010616,-0.219266399693367,
15.6608495079931));
#24306=CARTESIAN_POINT('Ctrl Pts',(-1.21364981772633,-1.00437124126938,
15.3786380262801));
#24307=CARTESIAN_POINT('Ctrl Pts',(-1.18419738671256,-1.33912457693599,
15.1307661354804));
#24308=CARTESIAN_POINT('Ctrl Pts',(-1.14983621711478,-1.6792932828141,14.7905634620183));
#24309=CARTESIAN_POINT('Ctrl Pts',(-1.13020126291748,-1.83495172588154,
14.557619759006));
#24310=CARTESIAN_POINT('Ctrl Pts',(-1.10565757040559,-1.96644792402424,
14.240164168935));
#24311=CARTESIAN_POINT('Ctrl Pts',(-1.09829446266241,-2.00122704859806,
14.1429882818207));
#24312=CARTESIAN_POINT('Ctrl Pts',(-1.0835682468725,-2.05621222310087,13.9442324744642));
#24313=CARTESIAN_POINT('Ctrl Pts',(-1.05411581628574,-2.12713274945685,
13.5368487102677));
#24314=CARTESIAN_POINT('Ctrl Pts',(-1.01730027703454,-2.07558331110669,
13.0140445022799));
#24315=CARTESIAN_POINT('Ctrl Pts',(-0.978030368980419,-1.86393795722917,
12.5036741054457));
#24316=CARTESIAN_POINT('Ctrl Pts',(-0.953486676180038,-1.67220003622907,
12.2165761921044));
#24317=CARTESIAN_POINT('Ctrl Pts',(-0.938760460748136,-1.53355113591613,
12.0636380569739));
#24318=CARTESIAN_POINT('Ctrl Pts',(-0.92403424516514,-1.38777482274071,
11.9178520451545));
#24319=CARTESIAN_POINT('Ctrl Pts',(-0.904399291043347,-1.1742634362821,
11.7425661865439));
#24320=CARTESIAN_POINT('Ctrl Pts',(-0.884764336947749,-0.930655306467975,
11.6124317243282));
#24321=CARTESIAN_POINT('Ctrl Pts',(-0.84549442877046,-0.422795803049391,
11.4014872112732));
#24322=CARTESIAN_POINT('Ctrl Pts',(-0.798861412839077,0.255001957070318,
11.335773527586));
#24323=CARTESIAN_POINT('Ctrl Pts',(-0.735047811954554,1.10113310782084,
11.6633392165017));
#24324=CARTESIAN_POINT('Ctrl Pts',(-0.685960426710027,1.62914331739752,
12.1183931288629));
#24325=CARTESIAN_POINT('Ctrl Pts',(-0.654053626379446,1.86126704948603,
12.5059440282019));
#24326=CARTESIAN_POINT('Ctrl Pts',(-0.624601195412295,2.01907157883037,
12.8868615420783));
#24327=CARTESIAN_POINT('Ctrl Pts',(-0.600057502795961,2.10343342036855,
13.2238084748929));
#24328=CARTESIAN_POINT('Ctrl Pts',(-0.570605071587877,2.10336458500336,
13.6381488881852));
#24329=CARTESIAN_POINT('Ctrl Pts',(-0.546061378980283,2.05290020198756,
13.9784521638003));
#24330=CARTESIAN_POINT('Ctrl Pts',(-0.53133516342537,1.99278329430259,14.1767068394653));
#24331=CARTESIAN_POINT('Ctrl Pts',(-0.519063317041293,1.92703808468239,
14.3354372284454));
#24332=CARTESIAN_POINT('Ctrl Pts',(-0.514154578439539,1.8991827786045,14.398284675188));
#24333=CARTESIAN_POINT('Ctrl Pts',(-0.504337101639833,1.83736662386643,
14.5210899579476));
#24334=CARTESIAN_POINT('Ctrl Pts',(-0.487156516667517,1.7135883000647,14.7276726331592));
#24335=CARTESIAN_POINT('Ctrl Pts',(-0.472430301157928,1.58214497145923,
14.8877980148624));
#24336=CARTESIAN_POINT('Ctrl Pts',(-0.435614762275021,1.2179310545379,15.2525189427683));
#24337=CARTESIAN_POINT('Ctrl Pts',(-0.381618638640641,0.535697183972207,
15.6386283611074));
#24338=CARTESIAN_POINT('Ctrl Pts',(-0.298170083766961,-0.675545338924911,
15.6090937700565));
#24339=CARTESIAN_POINT('Ctrl Pts',(-0.207358420958111,-1.78071661015833,
14.8720476608843));
#24340=CARTESIAN_POINT('Ctrl Pts',(-0.143544820167066,-2.10078048070695,
13.9811745633393));
#24341=CARTESIAN_POINT('Ctrl Pts',(-0.0748224810432098,-2.10079571528789,
13.018892234084));
#24342=CARTESIAN_POINT('Ctrl Pts',(-0.0110088802683666,-1.78076034062204,
12.1280093081936));
#24343=CARTESIAN_POINT('Ctrl Pts',(0.0798027825760428,-0.675612415650728,
11.3909286410548));
#24344=CARTESIAN_POINT('Ctrl Pts',(0.163251337403203,0.535627767915652,
11.3613573628603));
#24345=CARTESIAN_POINT('Ctrl Pts',(0.217247461051789,1.21787351269776,11.7474459840713));
#24346=CARTESIAN_POINT('Ctrl Pts',(0.254062999989602,1.58209728013173,12.1121568182762));
#24347=CARTESIAN_POINT('Ctrl Pts',(0.26633484629195,1.69164149438975,12.2455893496679));
#24348=CARTESIAN_POINT('Ctrl Pts',(0.281061061609305,1.80196383977949,12.4198331801394));
#24349=CARTESIAN_POINT('Ctrl Pts',(0.290878538947051,1.86973551168152,12.539455210692));
#24350=CARTESIAN_POINT('Ctrl Pts',(0.298241646680488,1.91386222842472,12.632757087791));
#24351=CARTESIAN_POINT('Ctrl Pts',(0.308059123789946,1.96646043482015,12.7597400679814));
#24352=CARTESIAN_POINT('Ctrl Pts',(0.322785339298095,2.03602087158878,12.9540884692955));
#24353=CARTESIAN_POINT('Ctrl Pts',(0.347329031870305,2.10336694998667,13.2927234020508));
#24354=CARTESIAN_POINT('Ctrl Pts',(0.381690201597044,2.10342891367037,13.7761229454928));
#24355=CARTESIAN_POINT('Ctrl Pts',(0.40623389420153,2.01909426618207,14.1130728120558));
#24356=CARTESIAN_POINT('Ctrl Pts',(0.435686325163057,1.8613003699308,14.4939896139498));
#24357=CARTESIAN_POINT('Ctrl Pts',(0.467593125498422,1.62918101096397,14.8816101604613));
#24358=CARTESIAN_POINT('Ctrl Pts',(0.516680510744503,1.10120661715989,15.3365095698264));
#24359=CARTESIAN_POINT('Ctrl Pts',(0.580494111628017,0.255029767888532,
15.6645333138311));
#24360=CARTESIAN_POINT('Ctrl Pts',(0.636944604582806,-0.565351704997995,
15.5841353192661));
#24361=CARTESIAN_POINT('Ctrl Pts',(0.686031989830427,-1.17415741609758,
15.257079999352));
#24362=CARTESIAN_POINT('Ctrl Pts',(0.705666943950803,-1.38772915100266,
15.0822244571842));
#24363=CARTESIAN_POINT('Ctrl Pts',(0.720393159536148,-1.53350604431233,
14.9364120026342));
#24364=CARTESIAN_POINT('Ctrl Pts',(0.735119374971491,-1.67216060831638,
14.7834847823105));
#24365=CARTESIAN_POINT('Ctrl Pts',(0.759663067736636,-1.86390687171186,
14.4963874011454));
#24366=CARTESIAN_POINT('Ctrl Pts',(0.798932975863961,-2.07556857418935,
13.9860258561317));
#24367=CARTESIAN_POINT('Ctrl Pts',(0.835748515047526,-2.12713404052499,
13.4632196613971));
#24368=CARTESIAN_POINT('Ctrl Pts',(0.865200945667048,-2.05622636621962,
13.0558339354759));
#24369=CARTESIAN_POINT('Ctrl Pts',(0.879927161444758,-2.00124743186629,
12.8570763057862));
#24370=CARTESIAN_POINT('Ctrl Pts',(0.887290269190745,-1.96647136320517,
12.75989931555));
#24371=CARTESIAN_POINT('Ctrl Pts',(0.911833961708695,-1.83498513568377,
12.4424394580257));
#24372=CARTESIAN_POINT('Ctrl Pts',(0.931468915902892,-1.67933397373734,
12.2094904271853));
#24373=CARTESIAN_POINT('Ctrl Pts',(0.965830085499491,-1.33917594806349,
11.8692768701963));
#24374=CARTESIAN_POINT('Ctrl Pts',(0.99528251651406,-1.00443038587671,11.6213942448987));
#24375=CARTESIAN_POINT('Ctrl Pts',(1.05418737889393,-0.219334396744861,
11.3391578691636));
#24376=CARTESIAN_POINT('Ctrl Pts',(1.09836602564571,0.422719333041569,11.4014569267992));
#24377=CARTESIAN_POINT('Ctrl Pts',(1.14499904153829,1.02590204107926,11.6518775623672));
#24378=CARTESIAN_POINT('Ctrl Pts',(1.17936021109236,1.43770339847263,11.9130681734602));
#24379=CARTESIAN_POINT('Ctrl Pts',(1.24317381189954,1.99756208939828,12.627560943781));
#24380=CARTESIAN_POINT('Ctrl Pts',(1.30698741287357,2.1793919241302,13.5415351936699));
#24381=CARTESIAN_POINT('Ctrl Pts',(1.37080101365562,1.93557754847214,14.4158542879512));
#24382=CARTESIAN_POINT('Ctrl Pts',(1.40516218321472,1.65515568903686,14.8148608582693));
#24383=CARTESIAN_POINT('Ctrl Pts',(1.44688646067973,1.24206712723018,15.2279662967193));
#24384=CARTESIAN_POINT('Ctrl Pts',(1.49106510750054,0.695431288255876,15.5552121917209));
#24385=CARTESIAN_POINT('Ctrl Pts',(1.55487870831301,-0.211280294656861,
15.6442888912545));
#24386=CARTESIAN_POINT('Ctrl Pts',(1.60396609336863,-0.881524522312744,
15.4409317243134));
#24387=CARTESIAN_POINT('Ctrl Pts',(1.63832726295486,-1.28336371294544,15.1721324773309));
#24388=CARTESIAN_POINT('Ctrl Pts',(1.65305347852583,-1.43631314893798,15.0335453274474));
#24389=CARTESIAN_POINT('Ctrl Pts',(1.66041658637534,-1.50920334155228,14.9606537902615));
#24390=CARTESIAN_POINT('Ctrl Pts',(1.67023406335438,-1.60402660101632,14.8610815159075));
#24391=CARTESIAN_POINT('Ctrl Pts',(1.69477775603514,-1.81587172112341,14.5894874803237));
#24392=CARTESIAN_POINT('Ctrl Pts',(1.74141077207343,-2.09905323873564,13.9929876745797));
#24393=CARTESIAN_POINT('Ctrl Pts',(1.80031563416003,-2.14068062617532,13.1444501566802));
#24394=CARTESIAN_POINT('Ctrl Pts',(1.86412923492969,-1.79136523454947,12.3029338445012));
#24395=CARTESIAN_POINT('Ctrl Pts',(1.92548846647922,-1.17253132238636,11.6835425466965));
#24396=CARTESIAN_POINT('Ctrl Pts',(1.98930206706247,-0.318356075436173,
11.3539088134527));
#24397=CARTESIAN_POINT('Ctrl Pts',(2.05557003701416,0.629726925134857,11.4238851191756));
#24398=CARTESIAN_POINT('Ctrl Pts',(2.1218380074072,1.45694422261059,11.8924922830572));
#24399=CARTESIAN_POINT('Ctrl Pts',(2.16601665398091,1.82184455239142,12.4106316046563));
#24400=CARTESIAN_POINT('Ctrl Pts',(2.19137846934136,1.95771445605756,12.7386611556245));
#24401=CARTESIAN_POINT('Ctrl Pts',(2.19506002321179,1.97588078470422,12.7869256444275));
#24402=CARTESIAN_POINT('Ctrl Pts',(2.19996876398827,1.99770550570674,12.8520909604627));
#24403=CARTESIAN_POINT('Ctrl Pts',(2.2065137316803,2.02538213011809,12.9394480697009));
#24404=CARTESIAN_POINT('Ctrl Pts',(2.21755844451523,2.06300081475712,13.0896209287977));
#24405=CARTESIAN_POINT('Ctrl Pts',(2.23228457099678,2.0932917010527,13.2938014535001));
#24406=CARTESIAN_POINT('Ctrl Pts',(2.24210211668464,2.10004670844963,13.4312473488259));
#24407=CARTESIAN_POINT('Ctrl Pts',(2.26664587493493,2.10005562155831,13.7748621762512));
#24408=CARTESIAN_POINT('Ctrl Pts',(2.28628054219918,2.04541956405879,14.0496593153248));
#24409=CARTESIAN_POINT('Ctrl Pts',(2.30837007995999,1.92707046676835,14.3353692677506));
#24410=CARTESIAN_POINT('Ctrl Pts',(2.33291408542307,1.78788494078656,14.6496709541517));
#24411=CARTESIAN_POINT('Ctrl Pts',(2.37709177928891,1.39799452919363,15.1490237584087));
#24412=CARTESIAN_POINT('Ctrl Pts',(2.44090672233169,0.5945258343695,15.578593294924));
#24413=CARTESIAN_POINT('Ctrl Pts',(2.50471913818021,-0.318078252393418,
15.6459868908612));
#24414=CARTESIAN_POINT('Ctrl Pts',(2.57344108274706,-1.23849201601544,15.2914055940067));
#24415=CARTESIAN_POINT('Ctrl Pts',(2.63266364818555,-1.81210740078466,14.6585754201023));
#24416=CARTESIAN_POINT('Ctrl Pts',(2.6697881072228,-1.99847008378947,14.1687025596367));
#24417=CARTESIAN_POINT('Ctrl Pts',(2.68237314822326,-2.04021308540786,13.9975277660334));
#24418=CARTESIAN_POINT('Ctrl Pts',(-2.51383678391223,2.04037051569869,13.9968784157014));
#24419=CARTESIAN_POINT('Ctrl Pts',(-2.51105452767153,2.03115422555428,14.0347239687683));
#24420=CARTESIAN_POINT('Ctrl Pts',(-2.50704508334344,2.01635591393393,14.0888928831956));
#24421=CARTESIAN_POINT('Ctrl Pts',(-2.50262659747871,1.99767306539875,14.1478678099595));
#24422=CARTESIAN_POINT('Ctrl Pts',(-2.49771785670229,1.97584974973882,14.2130335759246));
#24423=CARTESIAN_POINT('Ctrl Pts',(-2.49403630283137,1.95768474123331,14.261298444883));
#24424=CARTESIAN_POINT('Ctrl Pts',(-2.46867448746776,1.82182511115358,14.5893307981028));
#24425=CARTESIAN_POINT('Ctrl Pts',(-2.42449584089209,1.45695170113379,15.1074775399189));
#24426=CARTESIAN_POINT('Ctrl Pts',(-2.35822787050222,0.629751710402464,
15.5761019436571));
#24427=CARTESIAN_POINT('Ctrl Pts',(-2.29195990055035,-0.318321701676844,
15.6460980120573));
#24428=CARTESIAN_POINT('Ctrl Pts',(-2.22814629996575,-1.17249997604108,
15.3164821347062));
#24429=CARTESIAN_POINT('Ctrl Pts',(-2.1667870684196,-1.79134424397442,14.6971037747127));
#24430=CARTESIAN_POINT('Ctrl Pts',(-2.10297346764681,-2.14067522041323,
13.8555947608319));
#24431=CARTESIAN_POINT('Ctrl Pts',(-2.04406860556179,-2.09906516524119,
13.0070563621922));
#24432=CARTESIAN_POINT('Ctrl Pts',(-1.99743558952253,-1.81589548119543,
12.4105506139921));
#24433=CARTESIAN_POINT('Ctrl Pts',(-1.97289189684311,-1.60405595666689,
12.1389521317244));
#24434=CARTESIAN_POINT('Ctrl Pts',(-1.96307441986398,-1.50923476887834,
12.0393778713429));
#24435=CARTESIAN_POINT('Ctrl Pts',(-1.95571131201473,-1.43634609502682,
11.9664848049889));
#24436=CARTESIAN_POINT('Ctrl Pts',(-1.94098509644363,-1.28339953200227,
11.8278944487704));
#24437=CARTESIAN_POINT('Ctrl Pts',(-1.90662392685564,-0.881565884890355,
11.5590867757594));
#24438=CARTESIAN_POINT('Ctrl Pts',(-1.85753654179922,-0.211325685334219,
11.3557155604428));
#24439=CARTESIAN_POINT('Ctrl Pts',(-1.79372294098802,0.695387870237467,
11.4447732528524));
#24440=CARTESIAN_POINT('Ctrl Pts',(-1.74954429416882,1.24203070958418,11.7720077023501));
#24441=CARTESIAN_POINT('Ctrl Pts',(-1.70782001670461,1.65512797284224,12.1851044890556));
#24442=CARTESIAN_POINT('Ctrl Pts',(-1.6734588471444,1.93555824400004,12.584105187986));
#24443=CARTESIAN_POINT('Ctrl Pts',(-1.6096452463613,2.17939099147149,13.4584191984726));
#24444=CARTESIAN_POINT('Ctrl Pts',(-1.54583164538723,1.99758034946137,14.3723973010337));
#24445=CARTESIAN_POINT('Ctrl Pts',(-1.48201804458132,1.43773666005063,15.0869018769287));
#24446=CARTESIAN_POINT('Ctrl Pts',(-1.44765687502613,1.02594079907934,15.3481012030357));
#24447=CARTESIAN_POINT('Ctrl Pts',(-1.40102385913291,0.422763348534303,
15.5985345560026));
#24448=CARTESIAN_POINT('Ctrl Pts',(-1.35684521238158,-0.219289053323828,
15.6608472100048));
#24449=CARTESIAN_POINT('Ctrl Pts',(-1.29794035000175,-1.00439093500475,
15.3786274956859));
#24450=CARTESIAN_POINT('Ctrl Pts',(-1.26848791898798,-1.33914167588447,
15.1307520966607));
#24451=CARTESIAN_POINT('Ctrl Pts',(-1.2341267493902,-1.67930680851392,14.7905458562925));
#24452=CARTESIAN_POINT('Ctrl Pts',(-1.21449179519291,-1.8349628189688,14.5576005194465));
#24453=CARTESIAN_POINT('Ctrl Pts',(-1.18994810268102,-1.96645568244719,
14.2401435539693));
#24454=CARTESIAN_POINT('Ctrl Pts',(-1.18258499493783,-2.0012337895352,14.1429673007638));
#24455=CARTESIAN_POINT('Ctrl Pts',(-1.16785877914793,-2.05621688004258,
13.9442109190832));
#24456=CARTESIAN_POINT('Ctrl Pts',(-1.13840634856118,-2.12713313546642,
13.5368264082867));
#24457=CARTESIAN_POINT('Ctrl Pts',(-1.10159080930997,-2.07557821659641,
13.0140227425138));
#24458=CARTESIAN_POINT('Ctrl Pts',(-1.06232090125584,-1.86392751211601,
12.5036545650749));
#24459=CARTESIAN_POINT('Ctrl Pts',(-1.03777720845546,-1.6721865817914,12.2165586611969));
#24460=CARTESIAN_POINT('Ctrl Pts',(-1.02305099302356,-1.53353607750216,
12.0636219802384));
#24461=CARTESIAN_POINT('Ctrl Pts',(-1.00832477744056,-1.38775823789867,
11.9178374965157));
#24462=CARTESIAN_POINT('Ctrl Pts',(-0.988689823318778,-1.17424500879164,
11.7425538760864));
#24463=CARTESIAN_POINT('Ctrl Pts',(-0.969054869223174,-0.930635521833597,
11.6124219684523));
#24464=CARTESIAN_POINT('Ctrl Pts',(-0.929784961045884,-0.422773795796279,
11.4014827783018));
#24465=CARTESIAN_POINT('Ctrl Pts',(-0.883151945114507,0.255024643293703,
11.3357762016639));
#24466=CARTESIAN_POINT('Ctrl Pts',(-0.819338344229977,1.10115236427924,
11.6633507604566));
#24467=CARTESIAN_POINT('Ctrl Pts',(-0.770250958985457,1.62915780240659,
12.1184102084985));
#24468=CARTESIAN_POINT('Ctrl Pts',(-0.738344158654869,1.86127747045704,
12.5059635409483));
#24469=CARTESIAN_POINT('Ctrl Pts',(-0.708891727687721,2.01907800775109,
12.8868827095552));
#24470=CARTESIAN_POINT('Ctrl Pts',(-0.684348035071388,2.10343631582984,
13.223830526392));
#24471=CARTESIAN_POINT('Ctrl Pts',(-0.654895603863301,2.10336313724252,
13.6381709389644));
#24472=CARTESIAN_POINT('Ctrl Pts',(-0.630351911255712,2.05289518642211,
13.9784736853838));
#24473=CARTESIAN_POINT('Ctrl Pts',(-0.615625695700795,1.99277620041693,
14.1767277310439));
#24474=CARTESIAN_POINT('Ctrl Pts',(-0.603353849316717,1.92702932690731,
14.3354574303556));
#24475=CARTESIAN_POINT('Ctrl Pts',(-0.598445110714969,1.89917336159767,
14.3983045855388));
#24476=CARTESIAN_POINT('Ctrl Pts',(-0.588627633915256,1.83735592021535,
14.5211092192054));
#24477=CARTESIAN_POINT('Ctrl Pts',(-0.571447048942948,1.71357542899754,
14.7276905988158));
#24478=CARTESIAN_POINT('Ctrl Pts',(-0.556720833433352,1.5821304245265,14.8878145993562));
#24479=CARTESIAN_POINT('Ctrl Pts',(-0.519905294550446,1.21791267958507,
15.2525317138587));
#24480=CARTESIAN_POINT('Ctrl Pts',(-0.465909170916065,0.535674767624319,
15.6386339750025));
#24481=CARTESIAN_POINT('Ctrl Pts',(-0.382460616042388,-0.675567454408333,
15.6090866894905));
#24482=CARTESIAN_POINT('Ctrl Pts',(-0.291648953233538,-1.78073099288634,
14.8720289916999));
#24483=CARTESIAN_POINT('Ctrl Pts',(-0.227835352442492,-2.10078552644068,
13.9811525387388));
#24484=CARTESIAN_POINT('Ctrl Pts',(-0.159113013318636,-2.10079066955095,
13.0188702094965));
#24485=CARTESIAN_POINT('Ctrl Pts',(-0.0952994125437925,-1.78074595791222,
12.1279906389835));
#24486=CARTESIAN_POINT('Ctrl Pts',(-0.00448774969938476,-0.675590300139453,
11.3909215605209));
#24487=CARTESIAN_POINT('Ctrl Pts',(0.0789608051277796,0.535650184199022,
11.361362976682));
#24488=CARTESIAN_POINT('Ctrl Pts',(0.132956928776363,1.21789188774156,11.7474587552716));
#24489=CARTESIAN_POINT('Ctrl Pts',(0.169772467714179,1.58211182691082,12.1121734025769));
#24490=CARTESIAN_POINT('Ctrl Pts',(0.182044314016518,1.69165464540701,12.2456070858446));
#24491=CARTESIAN_POINT('Ctrl Pts',(0.196770529333881,1.80197516219225,12.4198520707251));
#24492=CARTESIAN_POINT('Ctrl Pts',(0.206588006671623,1.86974558093869,12.539474812745));
#24493=CARTESIAN_POINT('Ctrl Pts',(0.213951114405061,1.91387131899328,12.6327771518145));
#24494=CARTESIAN_POINT('Ctrl Pts',(0.223768591514521,1.96646819424218,12.7597606835474));
#24495=CARTESIAN_POINT('Ctrl Pts',(0.238494807022666,2.03602659373201,12.9541098141789));
#24496=CARTESIAN_POINT('Ctrl Pts',(0.26303849959488,2.10336912153095,13.2927454528611));
#24497=CARTESIAN_POINT('Ctrl Pts',(0.297399669321619,2.10342601846571,13.7761449969021));
#24498=CARTESIAN_POINT('Ctrl Pts',(0.321943361926104,2.01908783680841,14.1130939795258));
#24499=CARTESIAN_POINT('Ctrl Pts',(0.351395792887634,1.86128994972974,14.494009126764));
#24500=CARTESIAN_POINT('Ctrl Pts',(0.383302593222992,1.62916652410642,14.8816272398943));
#24501=CARTESIAN_POINT('Ctrl Pts',(0.43238997846908,1.10118736333318,15.3365211140863));
#24502=CARTESIAN_POINT('Ctrl Pts',(0.496203579352586,0.25500707638925,15.6645359872915));
#24503=CARTESIAN_POINT('Ctrl Pts',(0.552654072307385,-0.565373559877596,
15.5841293911837));
#24504=CARTESIAN_POINT('Ctrl Pts',(0.601741457554998,-1.17417583117015,
15.257067690362));
#24505=CARTESIAN_POINT('Ctrl Pts',(0.621376411675378,-1.38774574185824,
15.0822099078348));
#24506=CARTESIAN_POINT('Ctrl Pts',(0.636102627260723,-1.53352110099643,
14.9363959261039));
#24507=CARTESIAN_POINT('Ctrl Pts',(0.650828842696062,-1.67217406423484,
14.7834672512282));
#24508=CARTESIAN_POINT('Ctrl Pts',(0.675372535461211,-1.86391731608368,
14.4963678608596));
#24509=CARTESIAN_POINT('Ctrl Pts',(0.714642443588536,-2.07557366934684,
13.9860040962929));
#24510=CARTESIAN_POINT('Ctrl Pts',(0.751457982772098,-2.12713365409934,
13.4631973594635));
#24511=CARTESIAN_POINT('Ctrl Pts',(0.780910413391623,-2.05622170942674,
13.0558123800778));
#24512=CARTESIAN_POINT('Ctrl Pts',(0.795636629169332,-2.00124069083438,
12.8570553247401));
#24513=CARTESIAN_POINT('Ctrl Pts',(0.80299973691532,-1.96646360481137,12.759878700581));
#24514=CARTESIAN_POINT('Ctrl Pts',(0.827543429433267,-1.8349740425443,12.4424202184717));
#24515=CARTESIAN_POINT('Ctrl Pts',(0.847178383627465,-1.67932044807009,
12.2094728214553));
#24516=CARTESIAN_POINT('Ctrl Pts',(0.881539553224067,-1.33915884910206,
11.8692628313779));
#24517=CARTESIAN_POINT('Ctrl Pts',(0.910991984238634,-1.00441069214917,
11.6213837143031));
#24518=CARTESIAN_POINT('Ctrl Pts',(0.969896846618502,-0.219311743108901,
11.3391555711753));
#24519=CARTESIAN_POINT('Ctrl Pts',(1.0140754933703,0.422741337103771,11.401461357304));
#24520=CARTESIAN_POINT('Ctrl Pts',(1.06070850926287,1.02592141298073,11.6518883197597));
#24521=CARTESIAN_POINT('Ctrl Pts',(1.09506967881695,1.43772003638653,11.9130832441603));
#24522=CARTESIAN_POINT('Ctrl Pts',(1.15888327962412,1.99757123417929,12.627581886472));
#24523=CARTESIAN_POINT('Ctrl Pts',(1.22269688059815,2.17939148969465,13.5415580421266));
#24524=CARTESIAN_POINT('Ctrl Pts',(1.2865104813802,1.93556794510799,14.4158745779137));
#24525=CARTESIAN_POINT('Ctrl Pts',(1.3208716509393,1.6551419067762,14.8148782111249));
#24526=CARTESIAN_POINT('Ctrl Pts',(1.36259592840431,1.24204900760236,15.2279793178278));
#24527=CARTESIAN_POINT('Ctrl Pts',(1.40677457522512,0.69540974323271,15.555219482443));
#24528=CARTESIAN_POINT('Ctrl Pts',(1.47058817603759,-0.211302775492013,
15.6442866757422));
#24529=CARTESIAN_POINT('Ctrl Pts',(1.51967556109321,-0.881544870996376,
15.4409224823238));
#24530=CARTESIAN_POINT('Ctrl Pts',(1.55403673067944,-1.28338124194598,15.1721190230281));
#24531=CARTESIAN_POINT('Ctrl Pts',(1.56876294625041,-1.43632922636008,15.0335302691141));
#24532=CARTESIAN_POINT('Ctrl Pts',(1.57612605409992,-1.50921865417633,14.9606379685896));
#24533=CARTESIAN_POINT('Ctrl Pts',(1.58594353107896,-1.60404087000891,14.8610646978933));
#24534=CARTESIAN_POINT('Ctrl Pts',(1.61048722375972,-1.81588314242947,14.5894684454936));
#24535=CARTESIAN_POINT('Ctrl Pts',(1.65712023979801,-2.09905840693387,13.9929656680311));
#24536=CARTESIAN_POINT('Ctrl Pts',(1.71602510188461,-2.14067689814634,13.1444277157845));
#24537=CARTESIAN_POINT('Ctrl Pts',(1.77983870265428,-1.7913526847043,12.3029150640716));
#24538=CARTESIAN_POINT('Ctrl Pts',(1.8411979342038,-1.1725122789855,11.6835302547082));
#24539=CARTESIAN_POINT('Ctrl Pts',(1.90501153478705,-0.318333576394129,
11.3539054759517));
#24540=CARTESIAN_POINT('Ctrl Pts',(1.97127950473874,0.629748690539184,11.4238917221576));
#24541=CARTESIAN_POINT('Ctrl Pts',(2.03754747513178,1.45696107490744,11.8925075563253));
#24542=CARTESIAN_POINT('Ctrl Pts',(2.08172612170549,1.8218559736609,12.4106507069619));
#24543=CARTESIAN_POINT('Ctrl Pts',(2.10708793706594,1.95772243717073,12.7386816790409));
#24544=CARTESIAN_POINT('Ctrl Pts',(2.11076949093637,1.97588826019748,12.7869463583648));
#24545=CARTESIAN_POINT('Ctrl Pts',(2.11567823171285,1.99771229805176,12.8521119034831));
#24546=CARTESIAN_POINT('Ctrl Pts',(2.12222319940488,2.02538800399747,12.9394693025088));
#24547=CARTESIAN_POINT('Ctrl Pts',(2.13326791223981,2.06300512290958,13.0896425565393));
#24548=CARTESIAN_POINT('Ctrl Pts',(2.14799403872137,2.09329385346697,13.2938233974499));
#24549=CARTESIAN_POINT('Ctrl Pts',(2.15781158440922,2.10004742944095,13.4312693672659));
#24550=CARTESIAN_POINT('Ctrl Pts',(2.18235534265953,2.10005277188115,13.7748841760795));
#24551=CARTESIAN_POINT('Ctrl Pts',(2.20199000992373,2.04541374138347,14.0496807748905));
#24552=CARTESIAN_POINT('Ctrl Pts',(2.22407954768458,1.92706171431628,14.3353894648931));
#24553=CARTESIAN_POINT('Ctrl Pts',(2.24862355314762,1.78787291788821,14.6496897709558));
#24554=CARTESIAN_POINT('Ctrl Pts',(2.29280124701354,1.39797717703433,15.1490382788963));
#24555=CARTESIAN_POINT('Ctrl Pts',(2.35661619005622,0.594504104329255,15.5785996905196));
#24556=CARTESIAN_POINT('Ctrl Pts',(2.42042860590492,-0.318100812988892,
15.6459834169773));
#24557=CARTESIAN_POINT('Ctrl Pts',(2.48915055047148,-1.23851059813794,15.2913925342509));
#24558=CARTESIAN_POINT('Ctrl Pts',(2.54837311591077,-1.81212008137858,14.6585567792867));
#24559=CARTESIAN_POINT('Ctrl Pts',(2.58549757494722,-1.99847675263324,14.1686814022878));
#24560=CARTESIAN_POINT('Ctrl Pts',(2.5980826159495,-2.0402177892642,13.997506252196));
#24561=CARTESIAN_POINT('Ctrl Pts',(-2.59812731618765,2.04036530566024,13.9968998060665));
#24562=CARTESIAN_POINT('Ctrl Pts',(-2.59534505994695,2.03114861974595,14.0347452630157));
#24563=CARTESIAN_POINT('Ctrl Pts',(-2.59133561561887,2.01634974207102,14.088914022261));
#24564=CARTESIAN_POINT('Ctrl Pts',(-2.58691712975414,1.99766627284527,14.1478887530375));
#24565=CARTESIAN_POINT('Ctrl Pts',(-2.58200838897772,1.9758422746189,14.2130542894858));
#24566=CARTESIAN_POINT('Ctrl Pts',(-2.5783268351068,1.95767675979263,14.2613189694603));
#24567=CARTESIAN_POINT('Ctrl Pts',(-2.55296501974317,1.82181369270838,14.5893498915566));
#24568=CARTESIAN_POINT('Ctrl Pts',(-2.5087863731675,1.45693484860441,15.1074928158849));
#24569=CARTESIAN_POINT('Ctrl Pts',(-2.44251840277764,0.62972994555188,15.5761085436532));
#24570=CARTESIAN_POINT('Ctrl Pts',(-2.37625043282579,-0.318344200487585,
15.6460946753124));
#24571=CARTESIAN_POINT('Ctrl Pts',(-2.31243683224114,-1.17251901929372,
15.3164698418647));
#24572=CARTESIAN_POINT('Ctrl Pts',(-2.251077600695,-1.79135679412861,14.6970849956997));
#24573=CARTESIAN_POINT('Ctrl Pts',(-2.18726399992216,-2.14067894781455,
13.8555723158434));
#24574=CARTESIAN_POINT('Ctrl Pts',(-2.12835913783721,-2.09905999758198,
13.0070343576013));
#24575=CARTESIAN_POINT('Ctrl Pts',(-2.08172612179798,-1.81588405920725,
12.4105315721756));
#24576=CARTESIAN_POINT('Ctrl Pts',(-2.05718242911857,-1.60404168806122,
12.1389353188883));
#24577=CARTESIAN_POINT('Ctrl Pts',(-2.04736495213942,-1.50921945576282,
12.0393620480447));
#24578=CARTESIAN_POINT('Ctrl Pts',(-2.04000184429017,-1.43633001895298,
11.9664697474652));
#24579=CARTESIAN_POINT('Ctrl Pts',(-2.02527562871905,-1.2833820002978,11.8278809934843));
#24580=CARTESIAN_POINT('Ctrl Pts',(-1.99091445913108,-0.881545538385891,
11.5590775340104));
#24581=CARTESIAN_POINT('Ctrl Pts',(-1.94182707407465,-0.211303206956926,
11.3557133455025));
#24582=CARTESIAN_POINT('Ctrl Pts',(-1.8780134732634,0.69540941925258,11.4447805426057));
#24583=CARTESIAN_POINT('Ctrl Pts',(-1.83383482644428,1.24204881717818,11.7720207235788));
#24584=CARTESIAN_POINT('Ctrl Pts',(-1.79211054898006,1.65514176280649,12.1851218390422));
#24585=CARTESIAN_POINT('Ctrl Pts',(-1.75774937941984,1.9355678426377,12.584125483555));
#24586=CARTESIAN_POINT('Ctrl Pts',(-1.69393577863675,2.17939142999823,13.4584420456258));
#24587=CARTESIAN_POINT('Ctrl Pts',(-1.63012217766268,1.99757120080247,14.3724182414288));
#24588=CARTESIAN_POINT('Ctrl Pts',(-1.56630857685675,1.43772002594656,15.0869169536628));
#24589=CARTESIAN_POINT('Ctrl Pts',(-1.53194740730155,1.02592141791999,15.3481119548905));
#24590=CARTESIAN_POINT('Ctrl Pts',(-1.48531439140832,0.422741355371464,
15.598538991029));
#24591=CARTESIAN_POINT('Ctrl Pts',(-1.4411357446571,-0.21931170653463,15.6608449087876));
#24592=CARTESIAN_POINT('Ctrl Pts',(-1.3822308822772,-1.00441063212639,15.37861696754));
#24593=CARTESIAN_POINT('Ctrl Pts',(-1.3527784512634,-1.33915876666712,15.1307380565637));
#24594=CARTESIAN_POINT('Ctrl Pts',(-1.31841728166562,-1.67932034588269,
14.7905282515356));
#24595=CARTESIAN_POINT('Ctrl Pts',(-1.29878232746832,-1.83497389521851,
14.5575812868999));
#24596=CARTESIAN_POINT('Ctrl Pts',(-1.27423863495645,-1.96646344354817,
14.2401229366851));
#24597=CARTESIAN_POINT('Ctrl Pts',(-1.26687552721325,-2.00124052925931,
14.1429463218818));
#24598=CARTESIAN_POINT('Ctrl Pts',(-1.25214931142335,-2.05622153683595,
13.9441893596129));
#24599=CARTESIAN_POINT('Ctrl Pts',(-1.2226968808366,-2.12713352117015,13.5368041117153));
#24600=CARTESIAN_POINT('Ctrl Pts',(-1.18588134158537,-2.07557312081611,
13.0140009829725));
#24601=CARTESIAN_POINT('Ctrl Pts',(-1.14661143353127,-1.86391706588866,
12.5036350235708));
#24602=CARTESIAN_POINT('Ctrl Pts',(-1.12206774073086,-1.67217312482415,
12.2165411311398));
#24603=CARTESIAN_POINT('Ctrl Pts',(-1.10734152529897,-1.53352101847216,
12.0636059026328));
#24604=CARTESIAN_POINT('Ctrl Pts',(-1.09261530971597,-1.38774164664309,
11.9178229476107));
#24605=CARTESIAN_POINT('Ctrl Pts',(-1.07298035559411,-1.17422658984893,
11.7425415659256));
#24606=CARTESIAN_POINT('Ctrl Pts',(-1.05334540149858,-0.930615724615552,
11.6124122110264));
#24607=CARTESIAN_POINT('Ctrl Pts',(-1.01407549332128,-0.422751809620052,
11.401478347902));
#24608=CARTESIAN_POINT('Ctrl Pts',(-0.967442477390011,0.255047337510375,
11.3357788746702));
#24609=CARTESIAN_POINT('Ctrl Pts',(-0.903628876505371,1.10117161573409,
11.6633623053098));
#24610=CARTESIAN_POINT('Ctrl Pts',(-0.854541491260921,1.62917228431376,
12.1184272880757));
#24611=CARTESIAN_POINT('Ctrl Pts',(-0.822634690930238,1.86128789168044,
12.5059830549408));
#24612=CARTESIAN_POINT('Ctrl Pts',(-0.793182259963081,2.01908443269519,
12.8869038770426));
#24613=CARTESIAN_POINT('Ctrl Pts',(-0.768638567346796,2.10343921024085,
13.2238525787215));
#24614=CARTESIAN_POINT('Ctrl Pts',(-0.739186136138703,2.10336168670159,
13.6381929904004));
#24615=CARTESIAN_POINT('Ctrl Pts',(-0.714642443531089,2.05289016857552,
13.9784952079289));
#24616=CARTESIAN_POINT('Ctrl Pts',(-0.699916227976207,1.99276910397954,
14.1767486226491));
#24617=CARTESIAN_POINT('Ctrl Pts',(-0.68764438159213,1.92702056606835,14.3354776334837));
#24618=CARTESIAN_POINT('Ctrl Pts',(-0.682735642990384,1.89916394265223,
14.3983244956345));
#24619=CARTESIAN_POINT('Ctrl Pts',(-0.67291816619067,1.83734521207404,14.5211284832248));
#24620=CARTESIAN_POINT('Ctrl Pts',(-0.65573758121835,1.71356255861117,14.7277085610067));
#24621=CARTESIAN_POINT('Ctrl Pts',(-0.641011365708785,1.58211586986789,
14.8878311897117));
#24622=CARTESIAN_POINT('Ctrl Pts',(-0.604195826825868,1.2178943102614,15.2525444759611));
#24623=CARTESIAN_POINT('Ctrl Pts',(-0.550199703191467,0.535652337781153,
15.6386395941889));
#24624=CARTESIAN_POINT('Ctrl Pts',(-0.466751148317924,-0.675589555932738,
15.6090796029729));
#24625=CARTESIAN_POINT('Ctrl Pts',(-0.375939485509005,-1.78074537880574,
14.8720103239888));
#24626=CARTESIAN_POINT('Ctrl Pts',(-0.31212588471795,-2.10079056737381,
13.9811305159176));
#24627=CARTESIAN_POINT('Ctrl Pts',(-0.243403545594093,-2.10078562864891,
13.018848186645));
#24628=CARTESIAN_POINT('Ctrl Pts',(-0.179589944819259,-1.78073157198358,
12.127971971317));
#24629=CARTESIAN_POINT('Ctrl Pts',(-0.088778281974919,-0.67556819871279,
11.390914473911));
#24630=CARTESIAN_POINT('Ctrl Pts',(-0.00532972714761881,0.535672614096381,
11.3613685959817));
#24631=CARTESIAN_POINT('Ctrl Pts',(0.0486663965009476,1.21791025677753,
11.7474715171088));
#24632=CARTESIAN_POINT('Ctrl Pts',(0.0854819354387522,1.58212638175774,
12.1121899932069));
#24633=CARTESIAN_POINT('Ctrl Pts',(0.097753781741119,1.69166779517795,12.2456248179755));
#24634=CARTESIAN_POINT('Ctrl Pts',(0.112479997058482,1.80198648889417,12.4198709638171));
#24635=CARTESIAN_POINT('Ctrl Pts',(0.122297474396219,1.86975565182069,12.5394944142019));
#24636=CARTESIAN_POINT('Ctrl Pts',(0.129660582129661,1.91388041275862,12.6327972171707));
#24637=CARTESIAN_POINT('Ctrl Pts',(0.139478059239116,1.96647595649454,12.7597813000298));
#24638=CARTESIAN_POINT('Ctrl Pts',(0.154204274747277,2.0360323180508,12.9541311597142));
#24639=CARTESIAN_POINT('Ctrl Pts',(0.178747967319465,2.10337129653229,13.2927675044316));
#24640=CARTESIAN_POINT('Ctrl Pts',(0.213109137046184,2.1034231236121,13.7761670489127));
#24641=CARTESIAN_POINT('Ctrl Pts',(0.23765282965073,2.01908141283192,14.1131151470859));
#24642=CARTESIAN_POINT('Ctrl Pts',(0.267105260612252,1.86127952720513,14.4940286406423));
#24643=CARTESIAN_POINT('Ctrl Pts',(0.299012060947521,1.62915204416609,14.8816443196594));
#24644=CARTESIAN_POINT('Ctrl Pts',(0.34809944619367,1.10116811030529,15.3365326588097));
#24645=CARTESIAN_POINT('Ctrl Pts',(0.4119130470771,0.25498438275294,15.6645386602339));
#24646=CARTESIAN_POINT('Ctrl Pts',(0.468363540031971,-0.565395398106497,
15.5841234654303));
#24647=CARTESIAN_POINT('Ctrl Pts',(0.517450925279634,-1.17419426258121,
15.2570553788871));
#24648=CARTESIAN_POINT('Ctrl Pts',(0.537085879399974,-1.38776232212866,
15.0821953602152));
#24649=CARTESIAN_POINT('Ctrl Pts',(0.551812094985311,-1.53353616354587,
14.9363798480822));
#24650=CARTESIAN_POINT('Ctrl Pts',(0.56653831042067,-1.67218751851079,14.7834497214876));
#24651=CARTESIAN_POINT('Ctrl Pts',(0.591082003185787,-1.86392776386923,
14.4963483191671));
#24652=CARTESIAN_POINT('Ctrl Pts',(0.630351911313134,-2.07557876402105,
13.9859823368843));
#24653=CARTESIAN_POINT('Ctrl Pts',(0.667167450496672,-2.12713326926079,
13.4631750627901));
#24654=CARTESIAN_POINT('Ctrl Pts',(0.696619881116207,-2.05621705239711,
13.0557908206335));
#24655=CARTESIAN_POINT('Ctrl Pts',(0.711346096893909,-2.00123395135074,
12.8570343458293));
#24656=CARTESIAN_POINT('Ctrl Pts',(0.718709204639899,-1.96645584370435,
12.7598580832961));
#24657=CARTESIAN_POINT('Ctrl Pts',(0.743252897157858,-1.83496296645056,
12.4424009859059));
#24658=CARTESIAN_POINT('Ctrl Pts',(0.762887851352057,-1.67930691067268,
12.2094552167024));
#24659=CARTESIAN_POINT('Ctrl Pts',(0.797249020948654,-1.33914175837502,
11.8692487912752));
#24660=CARTESIAN_POINT('Ctrl Pts',(0.826701451963186,-1.00439099503339,
11.6213731861561));
#24661=CARTESIAN_POINT('Ctrl Pts',(0.885606314342979,-0.219289089925647,
11.3391532699561));
#24662=CARTESIAN_POINT('Ctrl Pts',(0.929784961094886,0.422763330259709,
11.4014657923317));
#24663=CARTESIAN_POINT('Ctrl Pts',(0.976417976987453,1.02594079413025,11.6518990716162));
#24664=CARTESIAN_POINT('Ctrl Pts',(1.01077914654152,1.43773667048348,11.9130983208989));
#24665=CARTESIAN_POINT('Ctrl Pts',(1.07459274734868,1.99758038283143,12.6276028268694));
#24666=CARTESIAN_POINT('Ctrl Pts',(1.13840634832269,2.17939105116197,13.5415808892922));
#24667=CARTESIAN_POINT('Ctrl Pts',(1.20221994910475,1.93555834646513,14.4158948734873));
#24668=CARTESIAN_POINT('Ctrl Pts',(1.23658111866385,1.65512811680158,14.8148955611299));
#24669=CARTESIAN_POINT('Ctrl Pts',(1.27830539612885,1.24203089999581,15.2279923390823));
#24670=CARTESIAN_POINT('Ctrl Pts',(1.32248404294974,0.695388194198749,15.5552267722387));
#24671=CARTESIAN_POINT('Ctrl Pts',(1.38629764376216,-0.211325253897595,
15.6442844608611));
#24672=CARTESIAN_POINT('Ctrl Pts',(1.43538502881776,-0.881565217530111,
15.4409132406642));
#24673=CARTESIAN_POINT('Ctrl Pts',(1.469746198404,-1.28339877368803,15.1721055678425));
#24674=CARTESIAN_POINT('Ctrl Pts',(1.48447241397496,-1.43634530247318,15.0335152116947));
#24675=CARTESIAN_POINT('Ctrl Pts',(1.49183552182448,-1.50923396733164,14.9606221453972));
#24676=CARTESIAN_POINT('Ctrl Pts',(1.5016529988035,-1.60405513865477,14.8610478851651));
#24677=CARTESIAN_POINT('Ctrl Pts',(1.52619669148426,-1.81589456446389,14.5894494037982));
#24678=CARTESIAN_POINT('Ctrl Pts',(1.57282970752259,-2.09906357467187,13.9929436636473));
#24679=CARTESIAN_POINT('Ctrl Pts',(1.63173456960926,-2.14067317084883,13.1444052710657));
#24680=CARTESIAN_POINT('Ctrl Pts',(1.69554817037887,-1.79134013475203,12.3028962855908));
#24681=CARTESIAN_POINT('Ctrl Pts',(1.75690740192841,-1.17249323607165,11.6835179627534));
#24682=CARTESIAN_POINT('Ctrl Pts',(1.82072100251162,-0.318311078103806,
11.3539021405768));
#24683=CARTESIAN_POINT('Ctrl Pts',(1.88698897246334,0.629770454452938,11.4238983246291));
#24684=CARTESIAN_POINT('Ctrl Pts',(1.95325694285639,1.45697792616486,11.8925228356508));
#24685=CARTESIAN_POINT('Ctrl Pts',(1.9974355894301,1.82186738996764,12.4106698060297));
#24686=CARTESIAN_POINT('Ctrl Pts',(2.02279740479054,1.95773041642441,12.738702209394));
#24687=CARTESIAN_POINT('Ctrl Pts',(2.02647895866097,1.97589573262478,12.7869670789265));
#24688=CARTESIAN_POINT('Ctrl Pts',(2.03138769943745,1.99771908858928,12.8521328519387));
#24689=CARTESIAN_POINT('Ctrl Pts',(2.03793266712948,2.02539387364681,12.9394905444958));
#24690=CARTESIAN_POINT('Ctrl Pts',(2.0489773799644,2.06300943248826,13.0896641864174));
#24691=CARTESIAN_POINT('Ctrl Pts',(2.06370350644596,2.09329599720291,13.2938453553922));
#24692=CARTESIAN_POINT('Ctrl Pts',(2.07352105213382,2.10004815600896,13.4312913837394));
#24693=CARTESIAN_POINT('Ctrl Pts',(2.09806481038409,2.10004987360911,13.7749062346504));
#24694=CARTESIAN_POINT('Ctrl Pts',(2.11769947764844,2.04540797017558,14.0497021502391));
#24695=CARTESIAN_POINT('Ctrl Pts',(2.13978901540921,1.92705294342672,14.3354096916135));
#24696=CARTESIAN_POINT('Ctrl Pts',(2.16433302087232,1.78786096674117,14.6497084864173));
#24697=CARTESIAN_POINT('Ctrl Pts',(2.20851071473805,1.39795979608125,15.1490528441138));
#24698=CARTESIAN_POINT('Ctrl Pts',(2.27232565778123,0.594482403270171,15.5786060645117));
#24699=CARTESIAN_POINT('Ctrl Pts',(2.33613807362933,-0.318123399654151,
15.6459799188749));
#24700=CARTESIAN_POINT('Ctrl Pts',(2.40486001819769,-1.23852912499723,15.2913795806851));
#24701=CARTESIAN_POINT('Ctrl Pts',(2.46408258363523,-1.81213280646108,14.6585380478362));
#24702=CARTESIAN_POINT('Ctrl Pts',(2.50120704267464,-1.99848332383328,14.1686604525656));
#24703=CARTESIAN_POINT('Ctrl Pts',(2.51379208367573,-2.04022249312054,13.9974847383588));
#24704=CARTESIAN_POINT('Ctrl Pts',(-2.68241784846308,2.04036009562041,13.9969211964378));
#24705=CARTESIAN_POINT('Ctrl Pts',(-2.67963559222238,2.03114301402161,14.0347665568773));
#24706=CARTESIAN_POINT('Ctrl Pts',(-2.6756261478943,2.01634357010855,14.0889351618321));
#24707=CARTESIAN_POINT('Ctrl Pts',(-2.67120766202956,1.99765948037072,14.1479096957282));
#24708=CARTESIAN_POINT('Ctrl Pts',(-2.66629892125314,1.97583479932944,14.2130750039397));
#24709=CARTESIAN_POINT('Ctrl Pts',(-2.66261736738221,1.95766877864201,14.2613394927813));
#24710=CARTESIAN_POINT('Ctrl Pts',(-2.63725555201859,1.82180227146093,14.5893689939159));
#24711=CARTESIAN_POINT('Ctrl Pts',(-2.59307690544293,1.45691799629554,15.1075080891233));
#24712=CARTESIAN_POINT('Ctrl Pts',(-2.52680893505306,0.629708180153284,
15.5761151466503));
#24713=CARTESIAN_POINT('Ctrl Pts',(-2.46054096510122,-0.31836669953251,
15.6460913378045));
#24714=CARTESIAN_POINT('Ctrl Pts',(-2.39672736451656,-1.17253806269356,
15.3164575498808));
#24715=CARTESIAN_POINT('Ctrl Pts',(-2.33536813297043,-1.79136934397512,
14.6970662152686));
#24716=CARTESIAN_POINT('Ctrl Pts',(-2.27155453219758,-2.14068267584376,
13.8555498749489));
#24717=CARTESIAN_POINT('Ctrl Pts',(-2.21264967011264,-2.09905482938455,
13.0070123510517));
#24718=CARTESIAN_POINT('Ctrl Pts',(-2.16601665407342,-1.81587263790155,
12.4105125373456));
#24719=CARTESIAN_POINT('Ctrl Pts',(-2.141472961394,-1.60402741906879,12.1389185008737));
#24720=CARTESIAN_POINT('Ctrl Pts',(-2.13165548441485,-1.50920414313901,
12.0393462263728));
#24721=CARTESIAN_POINT('Ctrl Pts',(-2.12429237656559,-1.43631394153121,
11.9664546891318));
#24722=CARTESIAN_POINT('Ctrl Pts',(-2.10956616099448,-1.28336447129704,
11.8278675391811));
#24723=CARTESIAN_POINT('Ctrl Pts',(-2.07520499140651,-0.881525189703381,
11.5590682920204));
#24724=CARTESIAN_POINT('Ctrl Pts',(-2.02611760635007,-0.21128072612125,
11.3557111299893));
#24725=CARTESIAN_POINT('Ctrl Pts',(-1.96230400553883,0.695430964275577,
11.4447878333271));
#24726=CARTESIAN_POINT('Ctrl Pts',(-1.9181253587197,1.2420669368066,11.7720337446871));
#24727=CARTESIAN_POINT('Ctrl Pts',(-1.87640108125549,1.65515554506745,12.1851391918979));
#24728=CARTESIAN_POINT('Ctrl Pts',(-1.84203991169527,1.93557744600219,12.5841457735168));
#24729=CARTESIAN_POINT('Ctrl Pts',(-1.77822631091218,2.17939186443456,13.4584648940827));
#24730=CARTESIAN_POINT('Ctrl Pts',(-1.71441270993811,1.99756205602226,14.3724391841198));
#24731=CARTESIAN_POINT('Ctrl Pts',(-1.65059910913218,1.43770338803263,15.0869320243634));
#24732=CARTESIAN_POINT('Ctrl Pts',(-1.61623793957698,1.02590204601976,15.3481227122834));
#24733=CARTESIAN_POINT('Ctrl Pts',(-1.56960492368374,0.422719351307122,
15.5985434215348));
#24734=CARTESIAN_POINT('Ctrl Pts',(-1.52542627693254,-0.21933436016509,
15.6608426107993));
#24735=CARTESIAN_POINT('Ctrl Pts',(-1.46652141455263,-1.00443032586176,
15.3786064369457));
#24736=CARTESIAN_POINT('Ctrl Pts',(-1.43706898353883,-1.3391758656156,15.130724017744));
#24737=CARTESIAN_POINT('Ctrl Pts',(-1.40270781394105,-1.67933387158251,
14.7905106458097));
#24738=CARTESIAN_POINT('Ctrl Pts',(-1.38307285974375,-1.83498498830578,
14.5575620473403));
#24739=CARTESIAN_POINT('Ctrl Pts',(-1.35852916723187,-1.96647120197112,
14.2401023217195));
#24740=CARTESIAN_POINT('Ctrl Pts',(-1.35116605948868,-2.00124727019645,
14.1429253408249));
#24741=CARTESIAN_POINT('Ctrl Pts',(-1.33643984369878,-2.05622619377765,
13.9441678042319));
#24742=CARTESIAN_POINT('Ctrl Pts',(-1.30698741311203,-2.12713390717972,
13.5367818097343));
#24743=CARTESIAN_POINT('Ctrl Pts',(-1.2701718738608,-2.07556802630583,13.0139792232064));
#24744=CARTESIAN_POINT('Ctrl Pts',(-1.2309019658067,-1.86390662077551,12.5036154832002));
#24745=CARTESIAN_POINT('Ctrl Pts',(-1.20635827300629,-1.67215967038646,
12.2165236002323));
#24746=CARTESIAN_POINT('Ctrl Pts',(-1.1916320575744,-1.53350596005819,12.0635898258973));
#24747=CARTESIAN_POINT('Ctrl Pts',(-1.1769058419914,-1.38772506180105,11.917808398972));
#24748=CARTESIAN_POINT('Ctrl Pts',(-1.15727088786955,-1.17420816235846,
11.7425292554681));
#24749=CARTESIAN_POINT('Ctrl Pts',(-1.13763593377401,-0.930595939981174,
11.6124024551505));
#24750=CARTESIAN_POINT('Ctrl Pts',(-1.09836602559671,-0.42272980236694,
11.4014739149307));
#24751=CARTESIAN_POINT('Ctrl Pts',(-1.05173300966544,0.25507002373376,11.3357815487481));
#24752=CARTESIAN_POINT('Ctrl Pts',(-0.987919408780793,1.10119087219249,
11.6633738492646));
#24753=CARTESIAN_POINT('Ctrl Pts',(-0.93883202353635,1.62918676932283,12.1184443677113));
#24754=CARTESIAN_POINT('Ctrl Pts',(-0.90692522320566,1.86129831265145,12.5060025676873));
#24755=CARTESIAN_POINT('Ctrl Pts',(-0.877472792238505,2.0190908616159,12.8869250445196));
#24756=CARTESIAN_POINT('Ctrl Pts',(-0.852929099622222,2.10344210570215,
13.2238746302206));
#24757=CARTESIAN_POINT('Ctrl Pts',(-0.823476668414125,2.10336023894075,
13.6382150411795));
#24758=CARTESIAN_POINT('Ctrl Pts',(-0.798932975806517,2.05288515301006,
13.9785167295123));
#24759=CARTESIAN_POINT('Ctrl Pts',(-0.784206760251632,1.99276201009388,
14.1767695142279));
#24760=CARTESIAN_POINT('Ctrl Pts',(-0.771934913867553,1.92701180829326,
14.335497835394));
#24761=CARTESIAN_POINT('Ctrl Pts',(-0.767026175265813,1.89915452564541,
14.3983444059853));
#24762=CARTESIAN_POINT('Ctrl Pts',(-0.757208698466093,1.83733450842296,
14.5211477444828));
#24763=CARTESIAN_POINT('Ctrl Pts',(-0.740028113493781,1.71354968754401,
14.7277265266632));
#24764=CARTESIAN_POINT('Ctrl Pts',(-0.725301897984208,1.58210132293516,
14.8878477742055));
#24765=CARTESIAN_POINT('Ctrl Pts',(-0.688486359101292,1.21787593530857,
15.2525572470515));
#24766=CARTESIAN_POINT('Ctrl Pts',(-0.634490235466891,0.535629921433265,
15.638645208084));
#24767=CARTESIAN_POINT('Ctrl Pts',(-0.551041680593352,-0.67561167141616,
15.6090725224069));
#24768=CARTESIAN_POINT('Ctrl Pts',(-0.460230017784431,-1.78075976153375,
14.8719916548044));
#24769=CARTESIAN_POINT('Ctrl Pts',(-0.396416416993376,-2.10079561310753,
13.9811084913171));
#24770=CARTESIAN_POINT('Ctrl Pts',(-0.327694077869519,-2.10078058291197,
13.0188261620575));
#24771=CARTESIAN_POINT('Ctrl Pts',(-0.263880477094685,-1.78071718927376,
12.1279533021069));
#24772=CARTESIAN_POINT('Ctrl Pts',(-0.173068814250347,-0.675546083201514,
11.3909073933772));
#24773=CARTESIAN_POINT('Ctrl Pts',(-0.0896202594230419,0.535695030379752,
11.3613742098035));
#24774=CARTESIAN_POINT('Ctrl Pts',(-0.0356241357744778,1.21792863182134,
11.7474842883091));
#24775=CARTESIAN_POINT('Ctrl Pts',(0.00119140316332885,1.58214092853682,
12.1122065775076));
#24776=CARTESIAN_POINT('Ctrl Pts',(0.0134632494656868,1.69168094619521,
12.2456425541522));
#24777=CARTESIAN_POINT('Ctrl Pts',(0.0281894647830582,1.80199781130694,
12.4198898544029));
#24778=CARTESIAN_POINT('Ctrl Pts',(0.0380069421207919,1.86976572107786,
12.539514016255));
#24779=CARTESIAN_POINT('Ctrl Pts',(0.0453700498542355,1.91388950332719,
12.6328172811942));
#24780=CARTESIAN_POINT('Ctrl Pts',(0.0551875269636911,1.96648371591656,
12.7598019155958));
#24781=CARTESIAN_POINT('Ctrl Pts',(0.0699137424718479,2.03603804019403,
12.9541525045977));
#24782=CARTESIAN_POINT('Ctrl Pts',(0.0944574350440407,2.10337346807658,
13.2927895552418));
#24783=CARTESIAN_POINT('Ctrl Pts',(0.128818604770759,2.10342022840744,13.7761891003219));
#24784=CARTESIAN_POINT('Ctrl Pts',(0.153362297375304,2.01907498345824,14.1131363145558));
#24785=CARTESIAN_POINT('Ctrl Pts',(0.182814728336829,1.86126910700408,14.4940481534565));
#24786=CARTESIAN_POINT('Ctrl Pts',(0.214721528672091,1.62913755730854,14.8816613990925));
#24787=CARTESIAN_POINT('Ctrl Pts',(0.263808913918248,1.10114885647858,15.3365442030697));
#24788=CARTESIAN_POINT('Ctrl Pts',(0.327622514801669,0.254961691253659,
15.6645413336943));
#24789=CARTESIAN_POINT('Ctrl Pts',(0.38407300775655,-0.565417252986099,
15.5841175373479));
#24790=CARTESIAN_POINT('Ctrl Pts',(0.433160393004205,-1.17421267765378,
15.2570430698972));
#24791=CARTESIAN_POINT('Ctrl Pts',(0.452795347124548,-1.38777891298425,
15.082180810866));
#24792=CARTESIAN_POINT('Ctrl Pts',(0.467521562709886,-1.53355122022996,
14.9363637715519));
#24793=CARTESIAN_POINT('Ctrl Pts',(0.482247778145241,-1.67220097442926,
14.7834321904053));
#24794=CARTESIAN_POINT('Ctrl Pts',(0.506791470910362,-1.86393820824105,
14.4963287788814));
#24795=CARTESIAN_POINT('Ctrl Pts',(0.546061379037708,-2.07558385917854,
13.9859605770456));
#24796=CARTESIAN_POINT('Ctrl Pts',(0.582876918221244,-2.12713288283513,
13.4631527608566));
#24797=CARTESIAN_POINT('Ctrl Pts',(0.612329348840782,-2.05621239560423,
13.0557692652354));
#24798=CARTESIAN_POINT('Ctrl Pts',(0.627055564618482,-2.00122721031883,
12.8570133647833));
#24799=CARTESIAN_POINT('Ctrl Pts',(0.634418672364474,-1.96644808531056,
12.7598374683271));
#24800=CARTESIAN_POINT('Ctrl Pts',(0.65896236488243,-1.83495187331109,12.4423817463518));
#24801=CARTESIAN_POINT('Ctrl Pts',(0.67859731907663,-1.67929338500544,12.2094376109722));
#24802=CARTESIAN_POINT('Ctrl Pts',(0.712958488673231,-1.33912465941359,
11.8692347524568));
#24803=CARTESIAN_POINT('Ctrl Pts',(0.74241091968776,-1.00437130130585,11.6213626555605));
#24804=CARTESIAN_POINT('Ctrl Pts',(0.801315782067549,-0.219266436289686,
11.3391509719678));
#24805=CARTESIAN_POINT('Ctrl Pts',(0.845494428819463,0.422785334321912,
11.4014702228365));
#24806=CARTESIAN_POINT('Ctrl Pts',(0.892127444712026,1.02596016603173,11.6519098290087));
#24807=CARTESIAN_POINT('Ctrl Pts',(0.926488614266094,1.43775330839738,11.913113391599));
#24808=CARTESIAN_POINT('Ctrl Pts',(0.990302215073251,1.99758952761244,12.6276237695603));
#24809=CARTESIAN_POINT('Ctrl Pts',(1.05411581604726,2.17939061672641,13.5416037377489));
#24810=CARTESIAN_POINT('Ctrl Pts',(1.11792941682932,1.93554874310097,14.4159151634498));
#24811=CARTESIAN_POINT('Ctrl Pts',(1.15229058638842,1.65511433454093,14.8149129139855));
#24812=CARTESIAN_POINT('Ctrl Pts',(1.19401486385342,1.24201278036798,15.2280053601908));
#24813=CARTESIAN_POINT('Ctrl Pts',(1.23819351067431,0.695366649175583,15.5552340629608));
#24814=CARTESIAN_POINT('Ctrl Pts',(1.30200711148673,-0.211347734732747,
15.6442822453488));
#24815=CARTESIAN_POINT('Ctrl Pts',(1.35109449654233,-0.881585566213743,
15.4409039986746));
#24816=CARTESIAN_POINT('Ctrl Pts',(1.38545566612857,-1.28341630268856,15.1720921135398));
#24817=CARTESIAN_POINT('Ctrl Pts',(1.40018188169953,-1.43636137989527,15.0335001533614));
#24818=CARTESIAN_POINT('Ctrl Pts',(1.40754498954905,-1.5092492799557,14.9606063237254));
#24819=CARTESIAN_POINT('Ctrl Pts',(1.41736246652807,-1.60406940764737,14.8610310671509));
#24820=CARTESIAN_POINT('Ctrl Pts',(1.44190615920883,-1.81590598576995,14.589430368968));
#24821=CARTESIAN_POINT('Ctrl Pts',(1.48853917524716,-2.0990687428701,13.9929216570987));
#24822=CARTESIAN_POINT('Ctrl Pts',(1.54744403733383,-2.14066944281984,13.1443828301699));
#24823=CARTESIAN_POINT('Ctrl Pts',(1.61125763810345,-1.79132758490686,12.3028775051611));
#24824=CARTESIAN_POINT('Ctrl Pts',(1.67261686965298,-1.17247419267079,11.6835056707651));
#24825=CARTESIAN_POINT('Ctrl Pts',(1.73643047023619,-0.318288579061762,
11.3538988030757));
#24826=CARTESIAN_POINT('Ctrl Pts',(1.80269844018791,0.629792219857265,11.4239049276112));
#24827=CARTESIAN_POINT('Ctrl Pts',(1.86896641058096,1.45699477846171,11.892538108919));
#24828=CARTESIAN_POINT('Ctrl Pts',(1.91314505715466,1.82187881123711,12.4106889083354));
#24829=CARTESIAN_POINT('Ctrl Pts',(1.93850687251511,1.95773839753758,12.7387227328106));
#24830=CARTESIAN_POINT('Ctrl Pts',(1.94218842638554,1.97590320811804,12.7869877928638));
#24831=CARTESIAN_POINT('Ctrl Pts',(1.94709716716202,1.99772588093429,12.8521537949592));
#24832=CARTESIAN_POINT('Ctrl Pts',(1.95364213485405,2.02539974752619,12.9395117773037));
#24833=CARTESIAN_POINT('Ctrl Pts',(1.96468684768897,2.06301374064072,13.089685814159));
#24834=CARTESIAN_POINT('Ctrl Pts',(1.97941297417053,2.09329814961718,13.293867299342));
#24835=CARTESIAN_POINT('Ctrl Pts',(1.98923051985839,2.10004887700028,13.4313134021794));
#24836=CARTESIAN_POINT('Ctrl Pts',(2.01377427810869,2.10004702393194,13.7749282344788));
#24837=CARTESIAN_POINT('Ctrl Pts',(2.03340894537298,2.04540214750026,14.0497236098048));
#24838=CARTESIAN_POINT('Ctrl Pts',(2.05549848313379,1.92704419097465,14.335429888756));
#24839=CARTESIAN_POINT('Ctrl Pts',(2.08004248859686,1.78784894384282,14.6497273032214));
#24840=CARTESIAN_POINT('Ctrl Pts',(2.12422018246268,1.39794244392195,15.1490673646013));
#24841=CARTESIAN_POINT('Ctrl Pts',(2.18803512550574,0.594460673229926,15.5786124601074));
#24842=CARTESIAN_POINT('Ctrl Pts',(2.25184754135404,-0.318145960249626,
15.645976444991));
#24843=CARTESIAN_POINT('Ctrl Pts',(2.3205694859221,-1.23854770711973,15.2913665209294));
#24844=CARTESIAN_POINT('Ctrl Pts',(2.37979205136044,-1.81214548705499,14.6585194070205));
#24845=CARTESIAN_POINT('Ctrl Pts',(2.41691651039905,-1.99848999267705,14.1686392952167));
#24846=CARTESIAN_POINT('Ctrl Pts',(2.42950155140196,-2.04022719697688,13.9974632245214));
#24847=CARTESIAN_POINT('Ctrl Pts',(-2.42950802845431,-0.728165094212968,
15.4695758861306));
#24848=CARTESIAN_POINT('Ctrl Pts',(-2.41776054273089,-0.882441814565159,
15.4125097574631));
#24849=CARTESIAN_POINT('Ctrl Pts',(-2.38637810294572,-1.27683944237258,
15.2120617751923));
#24850=CARTESIAN_POINT('Ctrl Pts',(-2.33536070898422,-1.79136934286978,
14.6970662169227));
#24851=CARTESIAN_POINT('Ctrl Pts',(-2.27154710821138,-2.14068267551541,
13.8555498769254));
#24852=CARTESIAN_POINT('Ctrl Pts',(-2.21264224612643,-2.09905482983975,
13.00701235299));
#24853=CARTESIAN_POINT('Ctrl Pts',(-2.16600923008721,-1.8158726389075,12.4105125390221));
#24854=CARTESIAN_POINT('Ctrl Pts',(-2.14146553740779,-1.60402742032555,
12.138918502355));
#24855=CARTESIAN_POINT('Ctrl Pts',(-2.13164806042864,-1.50920414448769,
12.0393462277663));
#24856=CARTESIAN_POINT('Ctrl Pts',(-2.12428495257939,-1.43631394294725,
11.9664546904581));
#24857=CARTESIAN_POINT('Ctrl Pts',(-2.10955873700828,-1.28336447284093,
11.8278675403661));
#24858=CARTESIAN_POINT('Ctrl Pts',(-2.0751975674203,-0.881525191495615,
11.5590682928344));
#24859=CARTESIAN_POINT('Ctrl Pts',(-2.02611018236387,-0.211280728101276,
11.3557111301844));
#24860=CARTESIAN_POINT('Ctrl Pts',(-1.96229658155262,0.695430962377974,
11.444787832685));
#24861=CARTESIAN_POINT('Ctrl Pts',(-1.91811793473349,1.24206693521069,11.7720337435403));
#24862=CARTESIAN_POINT('Ctrl Pts',(-1.87639365726928,1.65515554385356,12.1851391903695));
#24863=CARTESIAN_POINT('Ctrl Pts',(-1.84203248770906,1.93557744515636,12.5841457717297));
#24864=CARTESIAN_POINT('Ctrl Pts',(-1.77821888692597,2.1793918643963,13.4584648920703));
#24865=CARTESIAN_POINT('Ctrl Pts',(-1.7144052859519,1.9975620568277,14.3724391822753));
#24866=CARTESIAN_POINT('Ctrl Pts',(-1.65059168514597,1.43770338949803,15.086932023036));
#24867=CARTESIAN_POINT('Ctrl Pts',(-1.61623051559077,1.02590204772596,15.3481227113359));
#24868=CARTESIAN_POINT('Ctrl Pts',(-1.56959749969753,0.422719353245155,
15.5985434211446));
#24869=CARTESIAN_POINT('Ctrl Pts',(-1.52541885294633,-0.219334358169845,
15.6608426110017));
#24870=CARTESIAN_POINT('Ctrl Pts',(-1.46651399056642,-1.00443032412721,
15.3786064378732));
#24871=CARTESIAN_POINT('Ctrl Pts',(-1.43706155955262,-1.33917586410959,
15.1307240189805));
#24872=CARTESIAN_POINT('Ctrl Pts',(-1.40270038995484,-1.67933387039122,
14.7905106473604));
#24873=CARTESIAN_POINT('Ctrl Pts',(-1.38306543575754,-1.83498498732874,
14.5575620490349));
#24874=CARTESIAN_POINT('Ctrl Pts',(-1.35852174324566,-1.96647120128779,
14.2401023235352));
#24875=CARTESIAN_POINT('Ctrl Pts',(-1.35115863550247,-2.00124726960273,
14.1429253426728));
#24876=CARTESIAN_POINT('Ctrl Pts',(-1.33643241971257,-2.05622619336749,
13.9441678061304));
#24877=CARTESIAN_POINT('Ctrl Pts',(-1.30697998912582,-2.12713390714572,
13.5367818116986));
#24878=CARTESIAN_POINT('Ctrl Pts',(-1.27016444987459,-2.07556802675454,
13.0139792251229));
#24879=CARTESIAN_POINT('Ctrl Pts',(-1.23089454182049,-1.86390662169548,
12.5036154849212));
#24880=CARTESIAN_POINT('Ctrl Pts',(-1.20635084902008,-1.67215967157148,
12.2165236017764));
#24881=CARTESIAN_POINT('Ctrl Pts',(-1.19162463358819,-1.53350596138448,
12.0635898273133));
#24882=CARTESIAN_POINT('Ctrl Pts',(-1.17689841800519,-1.38772506326178,
11.9178084002534));
#24883=CARTESIAN_POINT('Ctrl Pts',(-1.15726346388334,-1.17420816398148,
11.7425292565524));
#24884=CARTESIAN_POINT('Ctrl Pts',(-1.1376285097878,-0.930595941723729,
11.6124024560098));
#24885=CARTESIAN_POINT('Ctrl Pts',(-1.0983586016105,-0.422729804305254,
11.4014739153211));
#24886=CARTESIAN_POINT('Ctrl Pts',(-1.05172558567923,0.255070021735645,
11.3357815485126));
#24887=CARTESIAN_POINT('Ctrl Pts',(-0.987911984794588,1.10119087049646,
11.6633738482479));
#24888=CARTESIAN_POINT('Ctrl Pts',(-0.938824599550145,1.62918676804705,
12.118444366207));
#24889=CARTESIAN_POINT('Ctrl Pts',(-0.906917799219455,1.86129831173361,
12.5060025659687));
#24890=CARTESIAN_POINT('Ctrl Pts',(-0.8774653682523,2.01909086104967,12.8869250426553));
#24891=CARTESIAN_POINT('Ctrl Pts',(-0.852921675636017,2.10344210544713,
13.2238746282784));
#24892=CARTESIAN_POINT('Ctrl Pts',(-0.82346924442792,2.10336023906826,13.6382150392374));
#24893=CARTESIAN_POINT('Ctrl Pts',(-0.798925551820312,2.05288515345181,
13.9785167276168));
#24894=CARTESIAN_POINT('Ctrl Pts',(-0.784199336265427,1.99276201071868,
14.1767695123879));
#24895=CARTESIAN_POINT('Ctrl Pts',(-0.771927489881348,1.92701180906461,
14.3354978336147));
#24896=CARTESIAN_POINT('Ctrl Pts',(-0.767018751279608,1.89915452647482,
14.3983444042317));
#24897=CARTESIAN_POINT('Ctrl Pts',(-0.757201274479887,1.8373345093657,14.5211477427863));
#24898=CARTESIAN_POINT('Ctrl Pts',(-0.740020689507575,1.71354968867764,
14.7277265250809));
#24899=CARTESIAN_POINT('Ctrl Pts',(-0.725294473998003,1.5821013242164,14.8878477727448));
#24900=CARTESIAN_POINT('Ctrl Pts',(-0.688478935115087,1.21787593692697,
15.2525572459267));
#24901=CARTESIAN_POINT('Ctrl Pts',(-0.634482811480685,0.535629923407611,
15.6386452075896));
#24902=CARTESIAN_POINT('Ctrl Pts',(-0.551034256607146,-0.675611669468313,
15.6090725230305));
#24903=CARTESIAN_POINT('Ctrl Pts',(-0.460222593798225,-1.78075976026697,
14.8719916564487));
#24904=CARTESIAN_POINT('Ctrl Pts',(-0.39640899300717,-2.10079561266312,
13.9811084932569));
#24905=CARTESIAN_POINT('Ctrl Pts',(-0.327686653883313,-2.10078058335638,
13.0188261639973));
#24906=CARTESIAN_POINT('Ctrl Pts',(-0.263873053108479,-1.78071719054053,
12.1279533037512));
#24907=CARTESIAN_POINT('Ctrl Pts',(-0.173061390264141,-0.675546085149363,
11.3909073940008));
#24908=CARTESIAN_POINT('Ctrl Pts',(-0.0896128354368363,0.535695028405412,
11.3613742093091));
#24909=CARTESIAN_POINT('Ctrl Pts',(-0.0356167117882722,1.21792863020294,
11.7474842871843));
#24910=CARTESIAN_POINT('Ctrl Pts',(0.00119882714953449,1.5821409272556,
12.1122065760469));
#24911=CARTESIAN_POINT('Ctrl Pts',(0.0134706734518924,1.69168094503692,
12.2456425525901));
#24912=CARTESIAN_POINT('Ctrl Pts',(0.0281968887692638,1.80199781030971,
12.4198898527391));
#24913=CARTESIAN_POINT('Ctrl Pts',(0.0380143661069976,1.869765720191,12.5395140145285));
#24914=CARTESIAN_POINT('Ctrl Pts',(0.0453774738404411,1.91388950252653,
12.632817279427));
#24915=CARTESIAN_POINT('Ctrl Pts',(0.0551949509498967,1.96648371523314,
12.7598019137801));
#24916=CARTESIAN_POINT('Ctrl Pts',(0.0699211664580535,2.03603803969005,
12.9541525027177));
#24917=CARTESIAN_POINT('Ctrl Pts',(0.0944648590302464,2.10337346788532,
13.2927895532997));
#24918=CARTESIAN_POINT('Ctrl Pts',(0.128826028756965,2.10342022866244,13.7761890983797));
#24919=CARTESIAN_POINT('Ctrl Pts',(0.15336972136151,2.01907498402452,14.1131363126915));
#24920=CARTESIAN_POINT('Ctrl Pts',(0.182822152323035,1.86126910792185,14.4940481517379));
#24921=CARTESIAN_POINT('Ctrl Pts',(0.214728952658297,1.62913755858449,14.8816613975882));
#24922=CARTESIAN_POINT('Ctrl Pts',(0.263816337904454,1.10114885817438,15.3365442020529));
#24923=CARTESIAN_POINT('Ctrl Pts',(0.327629938787875,0.254961693252239,
15.6645413334588));
#24924=CARTESIAN_POINT('Ctrl Pts',(0.384080431742756,-0.565417251061205,
15.58411753787));
#24925=CARTESIAN_POINT('Ctrl Pts',(0.433167816990411,-1.17421267603185,
15.2570430709813));
#24926=CARTESIAN_POINT('Ctrl Pts',(0.452802771110754,-1.38777891152299,
15.0821808121475));
#24927=CARTESIAN_POINT('Ctrl Pts',(0.467528986696092,-1.53355121890383,
14.9363637729679));
#24928=CARTESIAN_POINT('Ctrl Pts',(0.482255202131447,-1.67220097324411,
14.7834321919494));
#24929=CARTESIAN_POINT('Ctrl Pts',(0.506798894896568,-1.86393820732115,
14.4963287806024));
#24930=CARTESIAN_POINT('Ctrl Pts',(0.546068803023914,-2.07558385872978,
13.9859605789621));
#24931=CARTESIAN_POINT('Ctrl Pts',(0.58288434220745,-2.12713288286917,13.4631527628209));
#24932=CARTESIAN_POINT('Ctrl Pts',(0.612336772826988,-2.05621239601438,
13.0557692671339));
#24933=CARTESIAN_POINT('Ctrl Pts',(0.627062988604688,-2.00122721091256,
12.8570133666312));
#24934=CARTESIAN_POINT('Ctrl Pts',(0.63442609635068,-1.96644808599389,12.7598374701428));
#24935=CARTESIAN_POINT('Ctrl Pts',(0.658969788868636,-1.83495187428813,
12.4423817480464));
#24936=CARTESIAN_POINT('Ctrl Pts',(0.678604743062836,-1.67929338619673,
12.2094376125229));
#24937=CARTESIAN_POINT('Ctrl Pts',(0.712965912659437,-1.3391246609196,11.8692347536933));
#24938=CARTESIAN_POINT('Ctrl Pts',(0.742418343673966,-1.0043713030404,11.621362656488));
#24939=CARTESIAN_POINT('Ctrl Pts',(0.801323206053755,-0.219266438284931,
11.3391509721702));
#24940=CARTESIAN_POINT('Ctrl Pts',(0.845501852805669,0.422785332383879,
11.4014702224463));
#24941=CARTESIAN_POINT('Ctrl Pts',(0.892134868698232,1.02596016432553,11.6519098280612));
#24942=CARTESIAN_POINT('Ctrl Pts',(0.9264960382523,1.43775330693198,11.9131133902716));
#24943=CARTESIAN_POINT('Ctrl Pts',(0.990309639059457,1.997589526807,12.6276237677157));
#24944=CARTESIAN_POINT('Ctrl Pts',(1.05412324003347,2.17939061676467,13.5416037357365));
#24945=CARTESIAN_POINT('Ctrl Pts',(1.11793684081553,1.9355487439468,14.4159151616627));
#24946=CARTESIAN_POINT('Ctrl Pts',(1.15229801037463,1.65511433575482,14.8149129124571));
#24947=CARTESIAN_POINT('Ctrl Pts',(1.19402228783963,1.24201278196389,15.228005359044));
#24948=CARTESIAN_POINT('Ctrl Pts',(1.23820093466052,0.695366651073186,15.5552340623187));
#24949=CARTESIAN_POINT('Ctrl Pts',(1.30201453547294,-0.211347732752721,
15.6442822455439));
#24950=CARTESIAN_POINT('Ctrl Pts',(1.35110192052854,-0.881585564421509,
15.4409039994886));
#24951=CARTESIAN_POINT('Ctrl Pts',(1.38546309011478,-1.28341630114467,15.1720921147248));
#24952=CARTESIAN_POINT('Ctrl Pts',(1.40018930568574,-1.43636137847923,15.0335001546877));
#24953=CARTESIAN_POINT('Ctrl Pts',(1.40755241353526,-1.50924927860702,14.9606063251189));
#24954=CARTESIAN_POINT('Ctrl Pts',(1.41736989051428,-1.60406940639061,14.8610310686322));
#24955=CARTESIAN_POINT('Ctrl Pts',(1.44191358319504,-1.81590598476401,14.5894303706445));
#24956=CARTESIAN_POINT('Ctrl Pts',(1.48854659923337,-2.09906874241491,13.992921659037));
#24957=CARTESIAN_POINT('Ctrl Pts',(1.54745146132004,-2.14066944314819,13.1443828321464));
#24958=CARTESIAN_POINT('Ctrl Pts',(1.61126506208966,-1.7913275860122,12.3028775068152));
#24959=CARTESIAN_POINT('Ctrl Pts',(1.67262429363919,-1.17247419434806,11.6835056718477));
#24960=CARTESIAN_POINT('Ctrl Pts',(1.7364378942224,-0.318288581043391,11.3538988033697));
#24961=CARTESIAN_POINT('Ctrl Pts',(1.80270586417412,0.629792217940252,11.4239049270296));
#24962=CARTESIAN_POINT('Ctrl Pts',(1.86897383456717,1.45699477697742,11.8925381075738));
#24963=CARTESIAN_POINT('Ctrl Pts',(1.91315248114087,1.82187881023117,12.4106889066529));
#24964=CARTESIAN_POINT('Ctrl Pts',(1.93851429650132,1.95773839683463,12.738722731003));
#24965=CARTESIAN_POINT('Ctrl Pts',(1.94219585037175,1.97590320745963,12.7869877910394));
#24966=CARTESIAN_POINT('Ctrl Pts',(1.94710459114823,1.99772588033605,12.8521537931146));
#24967=CARTESIAN_POINT('Ctrl Pts',(1.95364955884026,2.02539974700884,12.9395117754336));
#24968=CARTESIAN_POINT('Ctrl Pts',(1.96469427167518,2.06301374026127,13.0896858122541));
#24969=CARTESIAN_POINT('Ctrl Pts',(1.97942039815674,2.0932981494276,13.2938672974093));
#24970=CARTESIAN_POINT('Ctrl Pts',(1.9892379438446,2.10004887693678,13.4313134002401));
#24971=CARTESIAN_POINT('Ctrl Pts',(2.0137817020949,2.10004702418293,13.7749282325411));
#24972=CARTESIAN_POINT('Ctrl Pts',(2.03341636935919,2.0454021480131,14.0497236079147));
#24973=CARTESIAN_POINT('Ctrl Pts',(2.05550590712,1.92704419174553,14.3354298869771));
#24974=CARTESIAN_POINT('Ctrl Pts',(2.08004991258307,1.78784894490175,14.6497273015641));
#24975=CARTESIAN_POINT('Ctrl Pts',(2.12422760644889,1.39794244545026,15.1490673633224));
#24976=CARTESIAN_POINT('Ctrl Pts',(2.18804254949195,0.594460675143825,15.5786124595441));
#24977=CARTESIAN_POINT('Ctrl Pts',(2.25185496534025,-0.318145958262575,
15.645976445297));
#24978=CARTESIAN_POINT('Ctrl Pts',(2.32057690990831,-1.23854770548309,15.2913665220797));
#24979=CARTESIAN_POINT('Ctrl Pts',(2.37979947534665,-1.81214548593813,14.6585194086623));
#24980=CARTESIAN_POINT('Ctrl Pts',(2.41692393438526,-1.99848999208968,14.1686392970802));
#24981=CARTESIAN_POINT('Ctrl Pts',(2.42950897538817,-2.04022719656258,13.9974632264163));
#24982=CARTESIAN_POINT('Ctrl Pts',(-2.42950819541373,2.04022498371351,13.9974756490669));
#24983=CARTESIAN_POINT('Ctrl Pts',(-2.42674114460071,2.03104804718875,14.0351116867474));
#24984=CARTESIAN_POINT('Ctrl Pts',(-2.42397402178904,2.02082976629947,14.0724948353366));
#24985=CARTESIAN_POINT('Ctrl Pts',(-2.42120691438128,2.00958510169509,14.1095664735261));
#24986=CARTESIAN_POINT('Ctrl Pts',(-2.41997973024847,2.00459820673664,14.126007369906));
#24987=CARTESIAN_POINT('Ctrl Pts',(-2.41875254898007,1.99940944248508,14.1423870005916));
#24988=CARTESIAN_POINT('Ctrl Pts',(-2.41752536541593,1.99402051067355,14.158700523574));
#24989=CARTESIAN_POINT('Ctrl Pts',(-2.41711630398564,1.99222419900596,14.1641383677883));
#24990=CARTESIAN_POINT('Ctrl Pts',(-2.41670724230984,1.99040564651285,14.1695688665664));
#24991=CARTESIAN_POINT('Ctrl Pts',(-2.41629818055378,1.98856490186073,14.1749918427932));
#24992=CARTESIAN_POINT('Ctrl Pts',(-2.41302569401814,1.97383897845102,14.2183755530088));
#24993=CARTESIAN_POINT('Ctrl Pts',(-2.40975320191403,1.95769276117011,14.2612778280205));
#24994=CARTESIAN_POINT('Ctrl Pts',(-2.40648070220672,1.94016289051323,14.3036048623514));
#24995=CARTESIAN_POINT('Ctrl Pts',(-2.38439162460657,1.82183784608482,14.5893085230205));
#24996=CARTESIAN_POINT('Ctrl Pts',(-2.3623022032065,1.63940406945196,14.8483855979339));
#24997=CARTESIAN_POINT('Ctrl Pts',(-2.34021273250533,1.41031970034931,15.0560301376478));
#24998=CARTESIAN_POINT('Ctrl Pts',(-2.31812341576338,1.18123692791921,15.2636732301204));
#24999=CARTESIAN_POINT('Ctrl Pts',(-2.29603411303243,0.905505533036176,
15.4198842057763));
#25000=CARTESIAN_POINT('Ctrl Pts',(-2.27394476221729,0.609627206226399,
15.5096574973231));
#25001=CARTESIAN_POINT('Ctrl Pts',(-2.25185547180329,0.313749688466697,
15.5994305433937));
#25002=CARTESIAN_POINT('Ctrl Pts',(-2.22976611622983,-0.00227496943738387,
15.6227660146606));
#25003=CARTESIAN_POINT('Ctrl Pts',(-2.20767679227486,-0.308126237136206,
15.5773863291275));
#25004=CARTESIAN_POINT('Ctrl Pts',(-2.18558744186399,-0.613977871146414,
15.5320065892441));
#25005=CARTESIAN_POINT('Ctrl Pts',(-2.16349812250749,-0.909656056643092,
15.4179117602001));
#25006=CARTESIAN_POINT('Ctrl Pts',(-2.14140882241474,-1.16674418597445,
15.2461753231618));
#25007=CARTESIAN_POINT('Ctrl Pts',(-2.12177391930598,-1.39526661487161,
15.0935209480874));
#25008=CARTESIAN_POINT('Ctrl Pts',(-2.10213903478246,-1.59329820329036,
14.8953227476681));
#25009=CARTESIAN_POINT('Ctrl Pts',(-2.0825041621263,-1.74605858618704,14.6667620421749));
#25010=CARTESIAN_POINT('Ctrl Pts',(-2.08250409479468,-1.74605911003076,
14.6667612583978));
#25011=CARTESIAN_POINT('Ctrl Pts',(-2.08250402746306,-1.74605963387394,
14.6667604746204));
#25012=CARTESIAN_POINT('Ctrl Pts',(-2.08250396013143,-1.7460601577166,14.6667596908426));
#25013=CARTESIAN_POINT('Ctrl Pts',(-2.06286901262028,-1.89882081250176,
14.4381979057571));
#25014=CARTESIAN_POINT('Ctrl Pts',(-2.04323407886215,-2.00630986779613,
14.1792734563894));
#25015=CARTESIAN_POINT('Ctrl Pts',(-2.02359915022586,-2.05986296659802,
13.9097172614467));
#25016=CARTESIAN_POINT('Ctrl Pts',(-1.99905543479842,-2.12680448910616,
13.5727712677571));
#25017=CARTESIAN_POINT('Ctrl Pts',(-1.97451177180188,-2.10947063979331,
13.2192131314304));
#25018=CARTESIAN_POINT('Ctrl Pts',(-1.94996810871334,-2.00982457650015,
12.8904089102543));
#25019=CARTESIAN_POINT('Ctrl Pts',(-1.94996807924008,-2.00982445684016,
12.8904085154097));
#25020=CARTESIAN_POINT('Ctrl Pts',(-1.94996804976682,-2.00982433718006,
12.8904081205652));
#25021=CARTESIAN_POINT('Ctrl Pts',(-1.94996802029356,-2.00982421751983,
12.8904077257206));
#25022=CARTESIAN_POINT('Ctrl Pts',(-1.93524184625727,-1.95003655762578,
12.6931255477529));
#25023=CARTESIAN_POINT('Ctrl Pts',(-1.92051567219421,-1.86061663401723,
12.5047548108404));
#25024=CARTESIAN_POINT('Ctrl Pts',(-1.90578949814881,-1.7460755686484,12.3333245625983));
#25025=CARTESIAN_POINT('Ctrl Pts',(-1.90578945655368,-1.746075245119,12.3333240783814));
#25026=CARTESIAN_POINT('Ctrl Pts',(-1.90578941495855,-1.74607492158938,
12.3333235941645));
#25027=CARTESIAN_POINT('Ctrl Pts',(-1.90578937336342,-1.74607459805957,
12.3333231099478));
#25028=CARTESIAN_POINT('Ctrl Pts',(-1.89842630966666,-1.68880417584947,
12.2476083052181));
#25029=CARTESIAN_POINT('Ctrl Pts',(-1.8910632459746,-1.62525351353008,12.1661286004572));
#25030=CARTESIAN_POINT('Ctrl Pts',(-1.88370018232131,-1.55602981070863,
12.0897478844421));
#25031=CARTESIAN_POINT('Ctrl Pts',(-1.88370013825672,-1.55602939643622,
12.0897474273382));
#25032=CARTESIAN_POINT('Ctrl Pts',(-1.88370009419213,-1.55602898216361,
12.0897469702345));
#25033=CARTESIAN_POINT('Ctrl Pts',(-1.88370005012754,-1.5560285678908,12.089746513131));
#25034=CARTESIAN_POINT('Ctrl Pts',(-1.88124572632274,-1.53295426671103,
12.0642866137492));
#25035=CARTESIAN_POINT('Ctrl Pts',(-1.87879140252236,-1.50924964356994,
12.0393932550014));
#25036=CARTESIAN_POINT('Ctrl Pts',(-1.87633707871304,-1.4849541104208,12.0150957483871));
#25037=CARTESIAN_POINT('Ctrl Pts',(-1.8763370332392,-1.48495366027189,12.0150952982016));
#25038=CARTESIAN_POINT('Ctrl Pts',(-1.87633698776536,-1.48495321012277,
12.0150948480164));
#25039=CARTESIAN_POINT('Ctrl Pts',(-1.87633694229152,-1.48495275997345,
12.0150943978313));
#25040=CARTESIAN_POINT('Ctrl Pts',(-1.87142825123432,-1.43636121939717,
11.9664989990058));
#25041=CARTESIAN_POINT('Ctrl Pts',(-1.86651956014098,-1.38537997155816,
11.9203021351265));
#25042=CARTESIAN_POINT('Ctrl Pts',(-1.86161086905512,-1.33225786159872,
11.8767037612623));
#25043=CARTESIAN_POINT('Ctrl Pts',(-1.86161082154616,-1.33225734745437,
11.8767033392938));
#25044=CARTESIAN_POINT('Ctrl Pts',(-1.86161077403721,-1.33225683330981,
11.8767029173255));
#25045=CARTESIAN_POINT('Ctrl Pts',(-1.86161072652826,-1.33225631916505,
11.8767024953575));
#25046=CARTESIAN_POINT('Ctrl Pts',(-1.85179329949156,-1.22601153083311,
11.7895054497431));
#25047=CARTESIAN_POINT('Ctrl Pts',(-1.84197587248468,-1.11120322439108,
11.7127024754497));
#25048=CARTESIAN_POINT('Ctrl Pts',(-1.83215844548016,-0.989982106116297,
11.6479419959326));
#25049=CARTESIAN_POINT('Ctrl Pts',(-1.83215839556304,-0.989981489762385,
11.6479416666551));
#25050=CARTESIAN_POINT('Ctrl Pts',(-1.83215834564591,-0.989980873408307,
11.6479413373781));
#25051=CARTESIAN_POINT('Ctrl Pts',(-1.83215829572879,-0.989980257054064,
11.6479410081013));
#25052=CARTESIAN_POINT('Ctrl Pts',(-1.81252337676606,-0.747537088060934,
11.5184198655243));
#25053=CARTESIAN_POINT('Ctrl Pts',(-1.79288845781252,-0.479442595783242,
11.4370689939149));
#25054=CARTESIAN_POINT('Ctrl Pts',(-1.77325353885603,-0.205901241008463,
11.4100931451571));
#25055=CARTESIAN_POINT('Ctrl Pts',(-1.77325350373935,-0.20590075178484,
11.4100930969113));
#25056=CARTESIAN_POINT('Ctrl Pts',(-1.77325346862266,-0.2059002625612,11.4100930486656));
#25057=CARTESIAN_POINT('Ctrl Pts',(-1.77325343350597,-0.205899773337542,
11.4100930004202));
#25058=CARTESIAN_POINT('Ctrl Pts',(-1.75361847943279,0.0676420901441113,
11.3831172979145));
#25059=CARTESIAN_POINT('Ctrl Pts',(-1.7339835253537,0.346630828755626,11.4105168521258));
#25060=CARTESIAN_POINT('Ctrl Pts',(-1.71434857242285,0.609603866520623,
11.4903764787249));
#25061=CARTESIAN_POINT('Ctrl Pts',(-1.68980486892179,0.938320328964335,
11.5902010621531));
#25062=CARTESIAN_POINT('Ctrl Pts',(-1.6652612051415,1.24201240084444,11.7719944916856));
#25063=CARTESIAN_POINT('Ctrl Pts',(-1.64071749321192,1.48501353328398,12.0149902447657));
#25064=CARTESIAN_POINT('Ctrl Pts',(-1.62353691580565,1.65511411862609,12.1850870645608));
#25065=CARTESIAN_POINT('Ctrl Pts',(-1.60635635576066,1.79533116747464,12.3845856394649));
#25066=CARTESIAN_POINT('Ctrl Pts',(-1.58917577804077,1.89826466745226,12.6020307354384));
#25067=CARTESIAN_POINT('Ctrl Pts',(-1.5719951880423,2.00119824099418,12.8194759868151));
#25068=CARTESIAN_POINT('Ctrl Pts',(-1.55481458653507,2.06684809797279,13.0548677492271));
#25069=CARTESIAN_POINT('Ctrl Pts',(-1.53763399538281,2.09027822246632,13.2941941600668));
#25070=CARTESIAN_POINT('Ctrl Pts',(-1.50818155323899,2.13044415039933,13.7044680095681));
#25071=CARTESIAN_POINT('Ctrl Pts',(-1.4787291219308,2.04653592497719,14.1263049840991));
#25072=CARTESIAN_POINT('Ctrl Pts',(-1.4492766906698,1.8524311106118,14.489997079784));
#25073=CARTESIAN_POINT('Ctrl Pts',(-1.43209610586582,1.73920330287967,14.7021508010533));
#25074=CARTESIAN_POINT('Ctrl Pts',(-1.41491552107903,1.5884779921667,14.8945191155991));
#25075=CARTESIAN_POINT('Ctrl Pts',(-1.39773493629675,1.41016704340693,15.0560041043591));
#25076=CARTESIAN_POINT('Ctrl Pts',(-1.38055437088535,1.23185629569033,15.2174889110469));
#25077=CARTESIAN_POINT('Ctrl Pts',(-1.3633738054772,1.02596005906369,15.3480904923515));
#25078=CARTESIAN_POINT('Ctrl Pts',(-1.34619324006513,0.803737867906403,
15.4403576967632));
#25079=CARTESIAN_POINT('Ctrl Pts',(-1.31674078958715,0.4227848594816,15.5985303298225));
#25080=CARTESIAN_POINT('Ctrl Pts',(-1.28728833908306,-0.00524924459700965,
15.6400763386564));
#25081=CARTESIAN_POINT('Ctrl Pts',(-1.25783590545734,-0.409628820444091,
15.5598546599255));
#25082=CARTESIAN_POINT('Ctrl Pts',(-1.24310969827096,-0.611818476196675,
15.5197438467804));
#25083=CARTESIAN_POINT('Ctrl Pts',(-1.22838349533185,-0.808094526764447,
15.4491910797825));
#25084=CARTESIAN_POINT('Ctrl Pts',(-1.21365729740076,-0.989920784653124,
15.3519468553259));
#25085=CARTESIAN_POINT('Ctrl Pts',(-1.19893106332822,-1.17174748878488,
15.2547023922097));
#25086=CARTESIAN_POINT('Ctrl Pts',(-1.18420483651807,-1.33912432283608,
15.1307663898753));
#25087=CARTESIAN_POINT('Ctrl Pts',(-1.16947859519051,-1.48491116620748,
14.984964988673));
#25088=CARTESIAN_POINT('Ctrl Pts',(-1.14984364421075,-1.6792932532193,14.7905634912569));
#25089=CARTESIAN_POINT('Ctrl Pts',(-1.13020869301272,-1.83495169412861,
14.5576198363276));
#25090=CARTESIAN_POINT('Ctrl Pts',(-1.11057373294137,-1.94014868488491,
14.3036552857682));
#25091=CARTESIAN_POINT('Ctrl Pts',(-1.10566499452238,-1.96644792400799,
14.2401641688082));
#25092=CARTESIAN_POINT('Ctrl Pts',(-1.10075625582403,-1.98963400801686,
14.175380241394));
#25093=CARTESIAN_POINT('Ctrl Pts',(-1.09584751722856,-2.00958163007088,
14.1096176421577));
#25094=CARTESIAN_POINT('Ctrl Pts',(-1.09339314802592,-2.01955544071146,
14.0767363438136));
#25095=CARTESIAN_POINT('Ctrl Pts',(-1.09093877881162,-2.02871963617376,
14.0436103770613));
#25096=CARTESIAN_POINT('Ctrl Pts',(-1.08848440943675,-2.03707029425241,
14.0102787380594));
#25097=CARTESIAN_POINT('Ctrl Pts',(-1.08112130266013,-2.06212226390212,
13.9102838393599));
#25098=CARTESIAN_POINT('Ctrl Pts',(-1.073758194709,-2.07985239778025,13.8084378943978));
#25099=CARTESIAN_POINT('Ctrl Pts',(-1.06639508644147,-2.08993525216245,
13.7058515180497));
#25100=CARTESIAN_POINT('Ctrl Pts',(-1.04676013622054,-2.11682285678353,
13.4322879196678));
#25101=CARTESIAN_POINT('Ctrl Pts',(-1.02712518272871,-2.08932984595779,
13.1534590171884));
#25102=CARTESIAN_POINT('Ctrl Pts',(-1.0074902241626,-2.00961703191972,12.8903925215421));
#25103=CARTESIAN_POINT('Ctrl Pts',(-0.9976727489314,-1.96976064135018,12.7588593280053));
#25104=CARTESIAN_POINT('Ctrl Pts',(-0.987855272123554,-1.91684930918749,
12.6312667292722));
#25105=CARTESIAN_POINT('Ctrl Pts',(-0.978037792689152,-1.85204603988445,
12.5100508178963));
#25106=CARTESIAN_POINT('Ctrl Pts',(-0.968220316533942,-1.78724279222673,
12.3888349470084));
#25107=CARTESIAN_POINT('Ctrl Pts',(-0.958402838465585,-1.71054761693102,
12.2739957704127));
#25108=CARTESIAN_POINT('Ctrl Pts',(-0.948585361863547,-1.62336083090999,
12.1677435485743));
#25109=CARTESIAN_POINT('Ctrl Pts',(-0.94367662333245,-1.5797674358562,12.1146174351651));
#25110=CARTESIAN_POINT('Ctrl Pts',(-0.938767885031536,-1.5335511375318,
12.0636380585001));
#25111=CARTESIAN_POINT('Ctrl Pts',(-0.933859146167239,-1.48495902976283,
12.0150427179392));
#25112=CARTESIAN_POINT('Ctrl Pts',(-0.924041681378216,-1.38777494231502,
11.9178521649162));
#25113=CARTESIAN_POINT('Ctrl Pts',(-0.914224210606306,-1.28101932887551,
11.8302092806163));
#25114=CARTESIAN_POINT('Ctrl Pts',(-0.904406743663767,-1.16673958206988,
11.753854257216));
#25115=CARTESIAN_POINT('Ctrl Pts',(-0.894589255603972,-1.05245958944984,
11.6774990695769));
#25116=CARTESIAN_POINT('Ctrl Pts',(-0.88477176938882,-0.930655414068331,
11.6124317688854));
#25117=CARTESIAN_POINT('Ctrl Pts',(-0.874954292095242,-0.803690428821663,
11.5596955953223));
#25118=CARTESIAN_POINT('Ctrl Pts',(-0.845501855242577,-0.422795408781944,
11.4014870479254));
#25119=CARTESIAN_POINT('Ctrl Pts',(-0.816049452022228,0.00528652468371188,
11.3599840213373));
#25120=CARTESIAN_POINT('Ctrl Pts',(-0.786597089225995,0.409645871011201,
11.4401775802091));
#25121=CARTESIAN_POINT('Ctrl Pts',(-0.786597056327444,0.409646322684179,
11.4401776697861));
#25122=CARTESIAN_POINT('Ctrl Pts',(-0.786597023428893,0.409646774357131,
11.4401777593631));
#25123=CARTESIAN_POINT('Ctrl Pts',(-0.786596990530342,0.409647226030055,
11.4401778489404));
#25124=CARTESIAN_POINT('Ctrl Pts',(-0.769416403546797,0.645524057364277,
11.4869576979523));
#25125=CARTESIAN_POINT('Ctrl Pts',(-0.752235817686795,0.87332860630921,
11.575148477315));
#25126=CARTESIAN_POINT('Ctrl Pts',(-0.735055235941776,1.07963262593515,
11.6988782710634));
#25127=CARTESIAN_POINT('Ctrl Pts',(-0.717874652738578,1.28593666307088,
11.8226080753131));
#25128=CARTESIAN_POINT('Ctrl Pts',(-0.700694074591393,1.47074018212349,
11.9818768663883));
#25129=CARTESIAN_POINT('Ctrl Pts',(-0.683513481359785,1.6233363607327,12.1677524954149));
#25130=CARTESIAN_POINT('Ctrl Pts',(-0.668787274631776,1.75413294277208,
12.3270742895953));
#25131=CARTESIAN_POINT('Ctrl Pts',(-0.654061054253819,1.86126702957128,
12.5059439796336));
#25132=CARTESIAN_POINT('Ctrl Pts',(-0.639334834882043,1.94016931490041,
12.696402786932));
#25133=CARTESIAN_POINT('Ctrl Pts',(-0.624608625535828,2.01907154651313,
12.8868614645667));
#25134=CARTESIAN_POINT('Ctrl Pts',(-0.609882413220272,2.06968867103886,
13.0890295728516));
#25135=CARTESIAN_POINT('Ctrl Pts',(-0.595156188405869,2.08991487504364,
13.294199089229));
#25136=CARTESIAN_POINT('Ctrl Pts',(-0.58533871587763,2.10339899637617,13.4309786179985));
#25137=CARTESIAN_POINT('Ctrl Pts',(-0.575521237900467,2.10337606278161,
13.5690921017574));
#25138=CARTESIAN_POINT('Ctrl Pts',(-0.565703756895726,2.08991123995878,
13.7058775206741));
#25139=CARTESIAN_POINT('Ctrl Pts',(-0.560795019318317,2.08317883255898,
13.7742701893794));
#25140=CARTESIAN_POINT('Ctrl Pts',(-0.555886280937762,2.07308595742924,
13.842330842726));
#25141=CARTESIAN_POINT('Ctrl Pts',(-0.550977541525792,2.05967771413265,
13.9097329223357));
#25142=CARTESIAN_POINT('Ctrl Pts',(-0.541160067288429,2.03286124006774,
14.0445370185767));
#25143=CARTESIAN_POINT('Ctrl Pts',(-0.531342589841728,1.9927833066971,14.1767068098724));
#25144=CARTESIAN_POINT('Ctrl Pts',(-0.5215251103279,1.94018712599076,14.3036911521357));
#25145=CARTESIAN_POINT('Ctrl Pts',(-0.519070741184284,1.92703808475101,
14.3354372281967));
#25146=CARTESIAN_POINT('Ctrl Pts',(-0.516616371956897,1.9131104322214,14.3668609506688));
#25147=CARTESIAN_POINT('Ctrl Pts',(-0.514162002461475,1.89841958485982,
14.3979234757846));
#25148=CARTESIAN_POINT('Ctrl Pts',(-0.51170763341165,1.88372874016539,14.428985995261));
#25149=CARTESIAN_POINT('Ctrl Pts',(-0.509253264130661,1.86827470105863,
14.4596873170088));
#25150=CARTESIAN_POINT('Ctrl Pts',(-0.506798894708835,1.8520778013819,14.4899921367648));
#25151=CARTESIAN_POINT('Ctrl Pts',(-0.501890157154438,1.81968401053648,
14.5506017603581));
#25152=CARTESIAN_POINT('Ctrl Pts',(-0.49698141893446,1.78431877874814,14.6096253783924));
#25153=CARTESIAN_POINT('Ctrl Pts',(-0.492072679301037,1.74613713236444,
14.6667661811286));
#25154=CARTESIAN_POINT('Ctrl Pts',(-0.482255202690933,1.66977386026196,
14.7810477556749));
#25155=CARTESIAN_POINT('Ctrl Pts',(-0.472437721954167,1.58214493861985,
14.8877980479252));
#25156=CARTESIAN_POINT('Ctrl Pts',(-0.462620248100799,1.48502125883098,
14.9850569304199));
#25157=CARTESIAN_POINT('Ctrl Pts',(-0.435622177181761,1.21793096309691,
15.2525190338407));
#25158=CARTESIAN_POINT('Ctrl Pts',(-0.408624102841353,0.876813824205406,
15.4455737261616));
#25159=CARTESIAN_POINT('Ctrl Pts',(-0.381626062624241,0.510319359615874,
15.5373233525677));
#25160=CARTESIAN_POINT('Ctrl Pts',(-0.354627945393328,0.143823849575187,
15.629073240696));
#25161=CARTESIAN_POINT('Ctrl Pts',(-0.327629911818704,-0.248048342260192,
15.6195176327191));
#25162=CARTESIAN_POINT('Ctrl Pts',(-0.300631877133074,-0.609642748411725,
15.509734974347));
#25163=CARTESIAN_POINT('Ctrl Pts',(-0.271179585708896,-1.00410789935089,
15.3899725218076));
#25164=CARTESIAN_POINT('Ctrl Pts',(-0.241727227064518,-1.36254128548648,
15.1509318358614));
#25165=CARTESIAN_POINT('Ctrl Pts',(-0.212274823799054,-1.62372373608068,
14.8324458723416));
#25166=CARTESIAN_POINT('Ctrl Pts',(-0.212274743641377,-1.62372444691498,
14.83244500555));
#25167=CARTESIAN_POINT('Ctrl Pts',(-0.212274663483701,-1.62372515774856,
14.8324441387578));
#25168=CARTESIAN_POINT('Ctrl Pts',(-0.212274583326024,-1.62372586858142,
14.8324432719651));
#25169=CARTESIAN_POINT('Ctrl Pts',(-0.177913437855339,-1.92843818387098,
14.4608757199683));
#25170=CARTESIAN_POINT('Ctrl Pts',(-0.143552266179561,-2.10078048114957,
13.9811748698202));
#25171=CARTESIAN_POINT('Ctrl Pts',(-0.109191126344327,-2.10078809799742,
13.5000333967581));
#25172=CARTESIAN_POINT('Ctrl Pts',(-0.0748299864062528,-2.10079571484529,
13.0188919222559));
#25173=CARTESIAN_POINT('Ctrl Pts',(-0.0404688972292225,-1.92846876156254,
12.5391857828251));
#25174=CARTESIAN_POINT('Ctrl Pts',(-0.00610780800733998,-1.6237682830356,
12.1676087467629));
#25175=CARTESIAN_POINT('Ctrl Pts',(-0.00610772729228924,-1.62376756728662,
12.1676078739192));
#25176=CARTESIAN_POINT('Ctrl Pts',(-0.00610764657723845,-1.62376685153691,
12.1676070010762));
#25177=CARTESIAN_POINT('Ctrl Pts',(-0.0061075658621877,-1.62376613578647,
12.1676061282337));
#25178=CARTESIAN_POINT('Ctrl Pts',(0.02334478860921,-1.36259383244188,11.8491120447897));
#25179=CARTESIAN_POINT('Ctrl Pts',(0.05279714312824,-1.00416802444854,11.61006015913));
#25180=CARTESIAN_POINT('Ctrl Pts',(0.0822494975908918,-0.609706932634201,
11.4902855935791));
#25181=CARTESIAN_POINT('Ctrl Pts',(0.0822495743794314,-0.609705904190406,
11.4902852813014));
#25182=CARTESIAN_POINT('Ctrl Pts',(0.0822496511679713,-0.609704875746364,
11.4902849690245));
#25183=CARTESIAN_POINT('Ctrl Pts',(0.0822497279565109,-0.60970384730208,
11.4902846567484));
#25184=CARTESIAN_POINT('Ctrl Pts',(0.109247743340253,-0.248114022230177,
11.3804917783663));
#25185=CARTESIAN_POINT('Ctrl Pts',(0.136245758689709,0.143756217175248,
11.3709246089638));
#25186=CARTESIAN_POINT('Ctrl Pts',(0.163243774048536,0.510253294332396,
11.4626631077541));
#25187=CARTESIAN_POINT('Ctrl Pts',(0.163243820507498,0.510253925011116,
11.4626632656204));
#25188=CARTESIAN_POINT('Ctrl Pts',(0.163243866966459,0.510254555689758,
11.4626634234869));
#25189=CARTESIAN_POINT('Ctrl Pts',(0.163243913425421,0.510255186368329,
11.4626635813538));
#25190=CARTESIAN_POINT('Ctrl Pts',(0.190241878204261,0.876751489577878,
11.5544022569341));
#25191=CARTESIAN_POINT('Ctrl Pts',(0.217239842989431,1.2178738606094,11.747446331933));
#25192=CARTESIAN_POINT('Ctrl Pts',(0.244237807829364,1.48497094349646,12.0149005971686));
#25193=CARTESIAN_POINT('Ctrl Pts',(0.244237904868314,1.48497190352514,12.0149015584811));
#25194=CARTESIAN_POINT('Ctrl Pts',(0.244238001907264,1.48497286355289,12.0149025197945));
#25195=CARTESIAN_POINT('Ctrl Pts',(0.244238098946214,1.48497382357971,12.0149034811088));
#25196=CARTESIAN_POINT('Ctrl Pts',(0.254055452352873,1.58209897381699,12.112158889888));
#25197=CARTESIAN_POINT('Ctrl Pts',(0.263872805766597,1.66973342405645,12.2189039991451));
#25198=CARTESIAN_POINT('Ctrl Pts',(0.273690159063131,1.74609831161928,12.3331820937207));
#25199=CARTESIAN_POINT('Ctrl Pts',(0.273690282714057,1.74609927344562,12.3331835330691));
#25200=CARTESIAN_POINT('Ctrl Pts',(0.273690406364982,1.74610023527018,12.3331849724187));
#25201=CARTESIAN_POINT('Ctrl Pts',(0.273690530015907,1.74610119709294,12.3331864117696));
#25202=CARTESIAN_POINT('Ctrl Pts',(0.276144769954554,1.76519158271812,12.3617548376027));
#25203=CARTESIAN_POINT('Ctrl Pts',(0.278599009885722,1.78357767573002,12.3907940324315));
#25204=CARTESIAN_POINT('Ctrl Pts',(0.281053249869367,1.80124177100558,12.4202656164393));
#25205=CARTESIAN_POINT('Ctrl Pts',(0.281053379138125,1.80124270140182,12.4202671687549));
#25206=CARTESIAN_POINT('Ctrl Pts',(0.281053508406883,1.80124363179606,12.4202687210717));
#25207=CARTESIAN_POINT('Ctrl Pts',(0.281053637675641,1.8012445621883,12.4202702733897));
#25208=CARTESIAN_POINT('Ctrl Pts',(0.283507872405506,1.8189085435929,12.4497418398569));
#25209=CARTESIAN_POINT('Ctrl Pts',(0.285962107187923,1.83585052932966,12.4796457923116));
#25210=CARTESIAN_POINT('Ctrl Pts',(0.288416341937125,1.85204792326276,12.5099480764146));
#25211=CARTESIAN_POINT('Ctrl Pts',(0.28841647645967,1.85204881108111,12.5099497373561));
#25212=CARTESIAN_POINT('Ctrl Pts',(0.288416610982214,1.85204969889722,12.5099513982988));
#25213=CARTESIAN_POINT('Ctrl Pts',(0.288416745504759,1.8520505867111,12.5099530592427));
#25214=CARTESIAN_POINT('Ctrl Pts',(0.293325339412051,1.88444603239207,12.5705592508536));
#25215=CARTESIAN_POINT('Ctrl Pts',(0.298233933186252,1.91386295584123,12.6327588437499));
#25216=CARTESIAN_POINT('Ctrl Pts',(0.303142526986869,1.94016133240765,12.6962485797819));
#25217=CARTESIAN_POINT('Ctrl Pts',(0.303142671740902,1.94016210794465,12.6962504520891));
#25218=CARTESIAN_POINT('Ctrl Pts',(0.303142816494935,1.94016288347893,12.6962523243973));
#25219=CARTESIAN_POINT('Ctrl Pts',(0.303142961248968,1.94016365901051,12.6962541967068));
#25220=CARTESIAN_POINT('Ctrl Pts',(0.308051545804713,1.96646180249381,12.7597438893171));
#25221=CARTESIAN_POINT('Ctrl Pts',(0.312960130387062,1.98964784013356,12.824524823218));
#25222=CARTESIAN_POINT('Ctrl Pts',(0.317868714962949,2.00959486168208,12.8902870681624));
#25223=CARTESIAN_POINT('Ctrl Pts',(0.317868868961942,2.00959548748799,12.8902891313476));
#25224=CARTESIAN_POINT('Ctrl Pts',(0.317869022960934,2.00959611329071,12.8902911945339));
#25225=CARTESIAN_POINT('Ctrl Pts',(0.317869176959927,2.00959673909024,12.8902932577211));
#25226=CARTESIAN_POINT('Ctrl Pts',(0.327686486540518,2.04949094636648,13.0218197521394));
#25227=CARTESIAN_POINT('Ctrl Pts',(0.337503796094336,2.07642872743024,13.1572715479576));
#25228=CARTESIAN_POINT('Ctrl Pts',(0.34732110568671,2.08990658617332,13.2940534921889));
#25229=CARTESIAN_POINT('Ctrl Pts',(0.347321273019919,2.08990681589953,13.2940558235977));
#25230=CARTESIAN_POINT('Ctrl Pts',(0.347321440353127,2.08990704562183,13.2940581550069));
#25231=CARTESIAN_POINT('Ctrl Pts',(0.347321607686336,2.08990727534022,13.2940604864164));
#25232=CARTESIAN_POINT('Ctrl Pts',(0.357138906642224,2.10338466063984,13.4308423277957));
#25233=CARTESIAN_POINT('Ctrl Pts',(0.366956205636128,2.10340210560045,13.5689542730069));
#25234=CARTESIAN_POINT('Ctrl Pts',(0.376773504604774,2.08991943609055,13.7057321885871));
#25235=CARTESIAN_POINT('Ctrl Pts',(0.37677368281039,2.08991919135038,13.7057346714078));
#25236=CARTESIAN_POINT('Ctrl Pts',(0.376773861016006,2.08991894660576,13.705737154228));
#25237=CARTESIAN_POINT('Ctrl Pts',(0.376774039221622,2.08991870185669,13.7057396370478));
#25238=CARTESIAN_POINT('Ctrl Pts',(0.391500037988321,2.06969389332211,13.9109071387579));
#25239=CARTESIAN_POINT('Ctrl Pts',(0.406226036698119,2.01909411423775,14.1130731793926));
#25240=CARTESIAN_POINT('Ctrl Pts',(0.420952035419789,1.94019731724951,14.303531214951));
#25241=CARTESIAN_POINT('Ctrl Pts',(0.420952252178541,1.94019615593125,14.3035340183905));
#25242=CARTESIAN_POINT('Ctrl Pts',(0.420952468937293,1.94019499460687,14.3035368218274));
#25243=CARTESIAN_POINT('Ctrl Pts',(0.420952685696044,1.94019383327638,14.3035396252619));
#25244=CARTESIAN_POINT('Ctrl Pts',(0.434481269190616,1.86771160838567,14.4785106329094));
#25245=CARTESIAN_POINT('Ctrl Pts',(0.448008986792176,1.77141272625529,14.6437074692471));
#25246=CARTESIAN_POINT('Ctrl Pts',(0.461537796611524,1.65482107705438,14.7929482633317));
#25247=CARTESIAN_POINT('Ctrl Pts',(0.462735448633046,1.64449967951663,14.8061599605257));
#25248=CARTESIAN_POINT('Ctrl Pts',(0.463933109214126,1.63401922235494,14.8192465934779));
#25249=CARTESIAN_POINT('Ctrl Pts',(0.465130779713237,1.62338213487436,14.8322038608054));
#25250=CARTESIAN_POINT('Ctrl Pts',(0.465130944545937,1.62338067091591,14.832205644085));
#25251=CARTESIAN_POINT('Ctrl Pts',(0.46513110937864,1.62337920695447,14.8322074273622));
#25252=CARTESIAN_POINT('Ctrl Pts',(0.465131274211341,1.62337774299007,14.8322092106369));
#25253=CARTESIAN_POINT('Ctrl Pts',(0.478955704393602,1.50059583489349,14.9817715028384));
#25254=CARTESIAN_POINT('Ctrl Pts',(0.492779776911533,1.35694827832357,15.1140870662735));
#25255=CARTESIAN_POINT('Ctrl Pts',(0.506603776941329,1.19804096667469,15.2245442356261));
#25256=CARTESIAN_POINT('Ctrl Pts',(0.509959725573088,1.15946423244761,15.251359092799));
#25257=CARTESIAN_POINT('Ctrl Pts',(0.513315669932859,1.11998833437995,15.2768859445942));
#25258=CARTESIAN_POINT('Ctrl Pts',(0.516671614100621,1.07969371213375,15.3010592167427));
#25259=CARTESIAN_POINT('Ctrl Pts',(0.516672103318057,1.07968783812906,15.3010627406351));
#25260=CARTESIAN_POINT('Ctrl Pts',(0.516672592535493,1.07968196410698,15.3010662644988));
#25261=CARTESIAN_POINT('Ctrl Pts',(0.516673081752929,1.07967609006749,15.3010697883337));
#25262=CARTESIAN_POINT('Ctrl Pts',(0.530551977098522,0.913032031030918,
15.4010395197798));
#25263=CARTESIAN_POINT('Ctrl Pts',(0.544428753882176,0.732367331110731,
15.4778744913662));
#25264=CARTESIAN_POINT('Ctrl Pts',(0.55830747106023,0.544729936753596,15.528371771255));
#25265=CARTESIAN_POINT('Ctrl Pts',(0.56160911318365,0.500092416067036,15.5403846932175));
#25266=CARTESIAN_POINT('Ctrl Pts',(0.564910865119463,0.455060225981205,
15.55090686959));
#25267=CARTESIAN_POINT('Ctrl Pts',(0.568212781513419,0.409728188158243,
15.559894738988));
#25268=CARTESIAN_POINT('Ctrl Pts',(0.568213447694807,0.409719042148382,
15.5598965523445));
#25269=CARTESIAN_POINT('Ctrl Pts',(0.56821411387619,0.409709896126496,15.5598983656384));
#25270=CARTESIAN_POINT('Ctrl Pts',(0.568214780057566,0.409700750092578,
15.5599001788699));
#25271=CARTESIAN_POINT('Ctrl Pts',(0.581928416503704,0.221425621908934,
15.5972263451643));
#25272=CARTESIAN_POINT('Ctrl Pts',(0.595639553657022,0.0280542714909028,
15.6080758169591));
#25273=CARTESIAN_POINT('Ctrl Pts',(0.609351027864107,-0.163321464899338,
15.5931068606506));
#25274=CARTESIAN_POINT('Ctrl Pts',(0.622795372555139,-0.3509687832454,15.5784295323608));
#25275=CARTESIAN_POINT('Ctrl Pts',(0.636240041294779,-0.53669963793286,
15.53892962429));
#25276=CARTESIAN_POINT('Ctrl Pts',(0.649687707863583,-0.713820511199585,
15.4751808339352));
#25277=CARTESIAN_POINT('Ctrl Pts',(0.651980844743659,-0.744023699584802,
15.4643101969012));
#25278=CARTESIAN_POINT('Ctrl Pts',(0.654274068794924,-0.773976462880374,
15.4527343431749));
#25279=CARTESIAN_POINT('Ctrl Pts',(0.656567393275285,-0.803645518258464,
15.4404559890673));
#25280=CARTESIAN_POINT('Ctrl Pts',(0.656568184580581,-0.80365575548431,
15.440451752455));
#25281=CARTESIAN_POINT('Ctrl Pts',(0.656568975885889,-0.803665992676384,
15.4404475157591));
#25282=CARTESIAN_POINT('Ctrl Pts',(0.656569767191209,-0.803676229834673,
15.4404432789796));
#25283=CARTESIAN_POINT('Ctrl Pts',(0.663812108772192,-0.897370781476111,
15.4016665844495));
#25284=CARTESIAN_POINT('Ctrl Pts',(0.671052677623533,-0.988141871459333,
15.3559275979264));
#25285=CARTESIAN_POINT('Ctrl Pts',(0.678292085188014,-1.07517040420396,
15.3039440676059));
#25286=CARTESIAN_POINT('Ctrl Pts',(0.680868544002631,-1.10614330196056,
15.285443461898));
#25287=CARTESIAN_POINT('Ctrl Pts',(0.683444855728359,-1.13664199148525,
15.2661514640664));
#25288=CARTESIAN_POINT('Ctrl Pts',(0.686021047927556,-1.16662883208436,
15.246099027821));
#25289=CARTESIAN_POINT('Ctrl Pts',(0.686022220568065,-1.16664248160322,
15.2460899002804));
#25290=CARTESIAN_POINT('Ctrl Pts',(0.6860233932087,-1.16665613101697,15.2460807725815));
#25291=CARTESIAN_POINT('Ctrl Pts',(0.686024565849459,-1.16666978032559,
15.2460716447245));
#25292=CARTESIAN_POINT('Ctrl Pts',(0.692997505214798,-1.24783342794592,
15.1917941575912));
#25293=CARTESIAN_POINT('Ctrl Pts',(0.699974870617991,-1.32527758889574,
15.1319195204613));
#25294=CARTESIAN_POINT('Ctrl Pts',(0.706951313639467,-1.39816345999789,
15.0669372185642));
#25295=CARTESIAN_POINT('Ctrl Pts',(0.709793278232913,-1.42785467433119,
15.0404656483637));
#25296=CARTESIAN_POINT('Ctrl Pts',(0.712635089759945,-1.45678979408922,
15.0131469672997));
#25297=CARTESIAN_POINT('Ctrl Pts',(0.715476386661461,-1.48491374763697,
14.9850161530564));
#25298=CARTESIAN_POINT('Ctrl Pts',(0.715476590101837,-1.48491576134687,
14.9850141388553));
#25299=CARTESIAN_POINT('Ctrl Pts',(0.71547679354221,-1.48491777505265,14.9850121246502));
#25300=CARTESIAN_POINT('Ctrl Pts',(0.715476996982581,-1.48491978875431,
14.985010110441));
#25301=CARTESIAN_POINT('Ctrl Pts',(0.720385621727778,-1.53350653583757,
14.9364111175307));
#25302=CARTESIAN_POINT('Ctrl Pts',(0.725294246463601,-1.57972464684981,
14.8854357575768));
#25303=CARTESIAN_POINT('Ctrl Pts',(0.730202871213679,-1.62331944447614,
14.832312607229));
#25304=CARTESIAN_POINT('Ctrl Pts',(0.730202985035305,-1.62332045535617,
14.8323113754047));
#25305=CARTESIAN_POINT('Ctrl Pts',(0.730203098856931,-1.62332146623479,
14.8323101435792));
#25306=CARTESIAN_POINT('Ctrl Pts',(0.730203212678557,-1.62332247711201,
14.8323089117526));
#25307=CARTESIAN_POINT('Ctrl Pts',(0.740020566846144,-1.71051275863889,
14.7260612791048));
#25308=CARTESIAN_POINT('Ctrl Pts',(0.749837921070188,-1.78720936133621,
14.6112244926074));
#25309=CARTESIAN_POINT('Ctrl Pts',(0.75965527526951,-1.8520153313365,14.490011685232));
#25310=CARTESIAN_POINT('Ctrl Pts',(0.759655398009369,-1.8520161415625,14.4900101697888));
#25311=CARTESIAN_POINT('Ctrl Pts',(0.759655520749229,-1.85201695178665,
14.4900086543445));
#25312=CARTESIAN_POINT('Ctrl Pts',(0.759655643489088,-1.85201776200893,
14.4900071388993));
#25313=CARTESIAN_POINT('Ctrl Pts',(0.769472986443132,-1.91682336045115,
14.3687943109336));
#25314=CARTESIAN_POINT('Ctrl Pts',(0.77929032937172,-1.96973820656263,14.2412050332778));
#25315=CARTESIAN_POINT('Ctrl Pts',(0.78910767232613,-2.00959827133535,14.1096747058508));
#25316=CARTESIAN_POINT('Ctrl Pts',(0.789107806547215,-2.00959881629554,
14.10967290759));
#25317=CARTESIAN_POINT('Ctrl Pts',(0.789107940768299,-2.0095993612533,14.1096711093284));
#25318=CARTESIAN_POINT('Ctrl Pts',(0.789108074989384,-2.00959990620861,
14.1096693110661));
#25319=CARTESIAN_POINT('Ctrl Pts',(0.808742936023748,-2.08932003286046,
13.846606094399));
#25320=CARTESIAN_POINT('Ctrl Pts',(0.82837779715767,-2.11682078260621,13.5677792192079));
#25321=CARTESIAN_POINT('Ctrl Pts',(0.84801265800844,-2.08994189988692,13.2942160069116));
#25322=CARTESIAN_POINT('Ctrl Pts',(0.848012751089102,-2.08994177246538,
13.2942147100629));
#25323=CARTESIAN_POINT('Ctrl Pts',(0.848012844169764,-2.08994164504261,
13.2942134132142));
#25324=CARTESIAN_POINT('Ctrl Pts',(0.848012937250426,-2.08994151761863,
13.2942121163657));
#25325=CARTESIAN_POINT('Ctrl Pts',(0.855375954735624,-2.07986181900396,
13.1916267014093));
#25326=CARTESIAN_POINT('Ctrl Pts',(0.862738972180859,-2.06213502104451,
13.089781475879));
#25327=CARTESIAN_POINT('Ctrl Pts',(0.870101989801644,-2.03708650871674,
12.989787025545));
#25328=CARTESIAN_POINT('Ctrl Pts',(0.870102079952299,-2.03708620203001,
12.9897858012419));
#25329=CARTESIAN_POINT('Ctrl Pts',(0.870102170102954,-2.03708589534218,
12.9897845769391));
#25330=CARTESIAN_POINT('Ctrl Pts',(0.870102260253609,-2.03708558865326,
12.9897833526366));
#25331=CARTESIAN_POINT('Ctrl Pts',(0.87255654094624,-2.02873622384413,12.9564526789597));
#25332=CARTESIAN_POINT('Ctrl Pts',(0.875010821658363,-2.01957337622892,
12.9233276386553));
#25333=CARTESIAN_POINT('Ctrl Pts',(0.877465102348043,-2.00960096503899,
12.890447224065));
#25334=CARTESIAN_POINT('Ctrl Pts',(0.87746519091255,-2.00960060517727,12.8904460375513));
#25335=CARTESIAN_POINT('Ctrl Pts',(0.877465279477059,-2.00960024531448,
12.8904448510379));
#25336=CARTESIAN_POINT('Ctrl Pts',(0.877465368041566,-2.00959988545065,
12.8904436645248));
#25337=CARTESIAN_POINT('Ctrl Pts',(0.882374021359468,-1.98965457264248,
12.8246816389388));
#25338=CARTESIAN_POINT('Ctrl Pts',(0.887282674587836,-1.96647088347394,
12.7598981571171));
#25339=CARTESIAN_POINT('Ctrl Pts',(0.892191327830066,-1.94017411668049,
12.6964073415817));
#25340=CARTESIAN_POINT('Ctrl Pts',(0.892191413138483,-1.94017365966399,
12.6964062381628));
#25341=CARTESIAN_POINT('Ctrl Pts',(0.892191498446901,-1.94017320264653,
12.6964051347442));
#25342=CARTESIAN_POINT('Ctrl Pts',(0.892191583755318,-1.94017274562812,
12.6964040313261));
#25343=CARTESIAN_POINT('Ctrl Pts',(0.911826482788449,-1.83498370745887,
12.4424372517412));
#25344=CARTESIAN_POINT('Ctrl Pts',(0.931461382050589,-1.67933317186298,
12.2094896248129));
#25345=CARTESIAN_POINT('Ctrl Pts',(0.951096281204927,-1.4849579573314,12.0150826785992));
#25346=CARTESIAN_POINT('Ctrl Pts',(0.951096336138496,-1.48495741351785,
12.0150821346969));
#25347=CARTESIAN_POINT('Ctrl Pts',(0.951096391072066,-1.48495686970399,
12.0150815907949));
#25348=CARTESIAN_POINT('Ctrl Pts',(0.951096446005635,-1.48495632588983,
12.0150810468931));
#25349=CARTESIAN_POINT('Ctrl Pts',(0.965822633066912,-1.33917462823082,
11.869275874655));
#25350=CARTESIAN_POINT('Ctrl Pts',(0.980548820070348,-1.17180250312542,
11.745335202403));
#25351=CARTESIAN_POINT('Ctrl Pts',(0.995275007116836,-0.989979777509019,
11.6480853541108));
#25352=CARTESIAN_POINT('Ctrl Pts',(0.995275035562517,-0.989979426293108,
11.6480851662591));
#25353=CARTESIAN_POINT('Ctrl Pts',(0.995275064008198,-0.989979075077144,
11.6480849784076));
#25354=CARTESIAN_POINT('Ctrl Pts',(0.995275092453878,-0.989978723861126,
11.6480847905562));
#25355=CARTESIAN_POINT('Ctrl Pts',(1.01000130806403,-0.808155589745198,
11.5508348567475));
#25356=CARTESIAN_POINT('Ctrl Pts',(1.02472752371917,-0.611881820252042,
11.4802759155044));
#25357=CARTESIAN_POINT('Ctrl Pts',(1.03945373105097,-0.409693485003987,
11.440158724781));
#25358=CARTESIAN_POINT('Ctrl Pts',(1.06890616740358,-0.00531651672141092,
11.3599242842489));
#25359=CARTESIAN_POINT('Ctrl Pts',(1.09835856480083,0.422718858224769,11.4014567292572));
#25360=CARTESIAN_POINT('Ctrl Pts',(1.12781103276819,0.803676834887431,11.5596173290528));
#25361=CARTESIAN_POINT('Ctrl Pts',(1.14499162521319,1.02590214187921,11.651877604455));
#25362=CARTESIAN_POINT('Ctrl Pts',(1.16217219918441,1.23180268872304,11.7824728394942));
#25363=CARTESIAN_POINT('Ctrl Pts',(1.17935278711131,1.41011865337131,11.9439522408167));
#25364=CARTESIAN_POINT('Ctrl Pts',(1.19653335546924,1.58843441491473,12.1054314582116));
#25365=CARTESIAN_POINT('Ctrl Pts',(1.2137139339289,1.73916557016386,12.2977947961871));
#25366=CARTESIAN_POINT('Ctrl Pts',(1.23089450663577,1.85239993741931,12.5099446821812));
#25367=CARTESIAN_POINT('Ctrl Pts',(1.26034695262402,2.04651623042694,12.8736306410409));
#25368=CARTESIAN_POINT('Ctrl Pts',(1.28979938757549,2.13043776648119,13.2954649769137));
#25369=CARTESIAN_POINT('Ctrl Pts',(1.31925182923742,2.09028477105871,13.7057401076938));
#25370=CARTESIAN_POINT('Ctrl Pts',(1.33643242010862,2.06686219052956,13.9450672659467));
#25371=CARTESIAN_POINT('Ctrl Pts',(1.35361300488886,2.001219748377,14.1804611088586));
#25372=CARTESIAN_POINT('Ctrl Pts',(1.37079358966893,1.89829301947601,14.3979096156095));
#25373=CARTESIAN_POINT('Ctrl Pts',(1.38797416029483,1.79536637537092,14.615357943216));
#25374=CARTESIAN_POINT('Ctrl Pts',(1.40515473092063,1.65515561944934,14.8148609281759));
#25375=CARTESIAN_POINT('Ctrl Pts',(1.42233530156288,1.4850603979144,14.9849630985979));
#25376=CARTESIAN_POINT('Ctrl Pts',(1.4468790083845,1.24206688296988,15.2279665405379));
#25377=CARTESIAN_POINT('Ctrl Pts',(1.4714227152453,0.938380485043318,15.4097695620104));
#25378=CARTESIAN_POINT('Ctrl Pts',(1.49596640169769,0.609667108510358,15.5096044609241));
#25379=CARTESIAN_POINT('Ctrl Pts',(1.51560133948904,0.346696559569775,15.5894723338038));
#25380=CARTESIAN_POINT('Ctrl Pts',(1.53523627501737,0.0677086654466856,
15.6168806170934));
#25381=CARTESIAN_POINT('Ctrl Pts',(1.55487121127339,-0.205834035211254,
15.5899134502986));
#25382=CARTESIAN_POINT('Ctrl Pts',(1.55487123562311,-0.205834374437557,
15.589913416856));
#25383=CARTESIAN_POINT('Ctrl Pts',(1.55487125997282,-0.205834713663856,
15.5899133834133));
#25384=CARTESIAN_POINT('Ctrl Pts',(1.55487128432254,-0.205835052890142,
15.5899133499706));
#25385=CARTESIAN_POINT('Ctrl Pts',(1.57450623185346,-0.479377897118042,
15.562946032826));
#25386=CARTESIAN_POINT('Ctrl Pts',(1.59414118117083,-0.747475540434009,
15.4816032311223));
#25387=CARTESIAN_POINT('Ctrl Pts',(1.61377614654412,-0.98992317360716,15.3520891539012));
#25388=CARTESIAN_POINT('Ctrl Pts',(1.62359362126025,-1.1111468917757,15.2873321678649));
#25389=CARTESIAN_POINT('Ctrl Pts',(1.63341109989897,-1.22595810977214,15.2105323735039));
#25390=CARTESIAN_POINT('Ctrl Pts',(1.64322857734255,-1.3322060403397,15.1233381527734));
#25391=CARTESIAN_POINT('Ctrl Pts',(1.64813731592424,-1.38533000410731,15.0797410436524));
#25392=CARTESIAN_POINT('Ctrl Pts',(1.65304605413425,-1.43631314634105,15.0335453301341));
#25393=CARTESIAN_POINT('Ctrl Pts',(1.65795479310598,-1.48490661205212,14.9849509679522));
#25394=CARTESIAN_POINT('Ctrl Pts',(1.66040916231399,-1.50920334215706,14.9606537896119));
#25395=CARTESIAN_POINT('Ctrl Pts',(1.66286353177777,-1.53290915910416,14.935760718772));
#25396=CARTESIAN_POINT('Ctrl Pts',(1.66531790094196,-1.55598464741419,14.91030106731));
#25397=CARTESIAN_POINT('Ctrl Pts',(1.67268100955675,-1.62521112289486,14.8339221012835));
#25398=CARTESIAN_POINT('Ctrl Pts',(1.68004411584012,-1.68876464552562,14.7524439070898));
#25399=CARTESIAN_POINT('Ctrl Pts',(1.68740722417849,-1.74603796406667,14.6667303670645));
#25400=CARTESIAN_POINT('Ctrl Pts',(1.70213341481545,-1.8605843986006,14.4953035901415));
#25401=CARTESIAN_POINT('Ctrl Pts',(1.71685961218156,-1.9500100817809,14.3069354949345));
#25402=CARTESIAN_POINT('Ctrl Pts',(1.73158581284833,-2.00980375572884,14.1096551008173));
#25403=CARTESIAN_POINT('Ctrl Pts',(1.75612952953808,-2.10946007757489,13.7808537887058));
#25404=CARTESIAN_POINT('Ctrl Pts',(1.78067325411209,-2.12680487991182,13.4272960132384));
#25405=CARTESIAN_POINT('Ctrl Pts',(1.80521694776939,-2.0598735121679,13.0903479751824));
#25406=CARTESIAN_POINT('Ctrl Pts',(1.82485190274241,-2.00632841784409,12.8207895440898));
#25407=CARTESIAN_POINT('Ctrl Pts',(1.84448685684207,-1.89884663042453,12.5618614060858));
#25408=CARTESIAN_POINT('Ctrl Pts',(1.86412181094562,-1.74609230897846,12.3332947925067));
#25409=CARTESIAN_POINT('Ctrl Pts',(1.8837567530877,-1.59333808058931,12.104728318169));
#25410=CARTESIAN_POINT('Ctrl Pts',(1.90339169523091,-1.3953113626414,11.9065233012212));
#25411=CARTESIAN_POINT('Ctrl Pts',(1.92302663734601,-1.16679229992759,11.7538614684367));
#25412=CARTESIAN_POINT('Ctrl Pts',(1.94511597261414,-0.909708058891522,
11.5821167091573));
#25413=CARTESIAN_POINT('Ctrl Pts',(1.967205307845,-0.614031857234684,11.4680127023866));
#25414=CARTESIAN_POINT('Ctrl Pts',(1.98929464309025,-0.308179898006852,
11.4226234687801));
#25415=CARTESIAN_POINT('Ctrl Pts',(2.01138396637403,-0.00232810439934122,
11.3772342597521));
#25416=CARTESIAN_POINT('Ctrl Pts',(2.0334732896713,0.313699460404102,11.4005597148878));
#25417=CARTESIAN_POINT('Ctrl Pts',(2.05556261303284,0.60958282695562,11.4903236518632));
#25418=CARTESIAN_POINT('Ctrl Pts',(2.07765193645337,0.905466194297148,11.5800875890782));
#25419=CARTESIAN_POINT('Ctrl Pts',(2.09974125993653,1.18120528463916,11.7362899754543));
#25420=CARTESIAN_POINT('Ctrl Pts',(2.12183058332263,1.410299996729,11.9439261381736));
#25421=CARTESIAN_POINT('Ctrl Pts',(2.14391987100573,1.63939433853275,12.1515619652902));
#25422=CARTESIAN_POINT('Ctrl Pts',(2.16600915858905,1.82184454727678,12.4106315915512));
#25423=CARTESIAN_POINT('Ctrl Pts',(2.18809844591148,1.9401828561742,12.6963347633748));
#25424=CARTESIAN_POINT('Ctrl Pts',(2.18809848161448,1.94018304744489,12.696335225158));
#25425=CARTESIAN_POINT('Ctrl Pts',(2.18809851731748,1.9401832387154,12.6963356869412));
#25426=CARTESIAN_POINT('Ctrl Pts',(2.18809855302049,1.94018342998576,12.6963361487246));
#25427=CARTESIAN_POINT('Ctrl Pts',(2.19137100463778,1.95771481149831,12.7386620993256));
#25428=CARTESIAN_POINT('Ctrl Pts',(2.19464345624932,1.97386246874068,12.7815634093583));
#25429=CARTESIAN_POINT('Ctrl Pts',(2.19791590921346,1.98858967767696,12.8249462719838));
#25430=CARTESIAN_POINT('Ctrl Pts',(2.1979159499312,1.98858986092135,12.8249468117783));
#25431=CARTESIAN_POINT('Ctrl Pts',(2.19791599064894,1.98859004416552,12.8249473515729));
#25432=CARTESIAN_POINT('Ctrl Pts',(2.19791603136667,1.98859022740948,12.8249478913675));
#25433=CARTESIAN_POINT('Ctrl Pts',(2.19832505183986,1.99043096143246,12.8303702714888));
#25434=CARTESIAN_POINT('Ctrl Pts',(2.19873407233418,1.99224950487864,12.8358001745293));
#25435=CARTESIAN_POINT('Ctrl Pts',(2.19914309251777,1.99404581840139,12.8412374204345));
#25436=CARTESIAN_POINT('Ctrl Pts',(2.1991431337548,1.99404599950401,12.8412379686124));
#25437=CARTESIAN_POINT('Ctrl Pts',(2.19914317499182,1.9940461806064,12.8412385167904));
#25438=CARTESIAN_POINT('Ctrl Pts',(2.19914321622885,1.99404636170857,12.8412390649686));
#25439=CARTESIAN_POINT('Ctrl Pts',(2.20037035749464,1.9994356433095,12.8575518801008));
#25440=CARTESIAN_POINT('Ctrl Pts',(2.20159749596331,2.00462482923011,12.8739307895866));
#25441=CARTESIAN_POINT('Ctrl Pts',(2.20282463620707,2.0096121270271,12.8903709813945));
#25442=CARTESIAN_POINT('Ctrl Pts',(2.20282467920292,2.00961230176922,12.8903715574166));
#25443=CARTESIAN_POINT('Ctrl Pts',(2.20282472219877,2.00961247651109,12.8903721334389));
#25444=CARTESIAN_POINT('Ctrl Pts',(2.20282476519461,2.00961265125272,12.8903727094612));
#25445=CARTESIAN_POINT('Ctrl Pts',(2.20773344473922,2.02956226773413,12.956135082359));
#25446=CARTESIAN_POINT('Ctrl Pts',(2.21264215268916,2.04628151524348,13.0228780180129));
#25447=CARTESIAN_POINT('Ctrl Pts',(2.21755083441069,2.05968958847734,13.0902792715416));
#25448=CARTESIAN_POINT('Ctrl Pts',(2.2175508877071,2.05968973405659,13.0902800033562));
#25449=CARTESIAN_POINT('Ctrl Pts',(2.21755094100351,2.05968987963544,13.0902807351709));
#25450=CARTESIAN_POINT('Ctrl Pts',(2.21755099429992,2.05969002521391,13.0902814669856));
#25451=CARTESIAN_POINT('Ctrl Pts',(2.22245966546082,2.07309799770043,13.1576825898092));
#25452=CARTESIAN_POINT('Ctrl Pts',(2.22736831039274,2.0831948122282,13.2257420223163));
#25453=CARTESIAN_POINT('Ctrl Pts',(2.23227698732179,2.08993197186516,13.294132840081));
#25454=CARTESIAN_POINT('Ctrl Pts',(2.23227705117833,2.08993205950827,13.294133729771));
#25455=CARTESIAN_POINT('Ctrl Pts',(2.23227711503487,2.0899321471508,13.2941346194611));
#25456=CARTESIAN_POINT('Ctrl Pts',(2.23227717889141,2.08993223479277,13.2941355091512));
#25457=CARTESIAN_POINT('Ctrl Pts',(2.23718584354925,2.09666929017565,13.3625261645558));
#25458=CARTESIAN_POINT('Ctrl Pts',(2.24209454020457,2.10004670853711,13.431248199927));
#25459=CARTESIAN_POINT('Ctrl Pts',(2.24700321565604,2.100048491072,13.4999703169702));
#25460=CARTESIAN_POINT('Ctrl Pts',(2.24700329190274,2.10004849109969,13.4999713844344));
#25461=CARTESIAN_POINT('Ctrl Pts',(2.24700336814945,2.10004849112656,13.4999724518985));
#25462=CARTESIAN_POINT('Ctrl Pts',(2.24700344439615,2.1000484911526,13.4999735193626));
#25463=CARTESIAN_POINT('Ctrl Pts',(2.26663826965199,2.10005519695717,13.7748637151604));
#25464=CARTESIAN_POINT('Ctrl Pts',(2.28627275562331,2.04541865167645,14.049661518633));
#25465=CARTESIAN_POINT('Ctrl Pts',(2.30590771896488,1.94022036581116,14.3036237190645));
#25466=CARTESIAN_POINT('Ctrl Pts',(2.30590790026447,1.94021939446198,14.3036260640264));
#25467=CARTESIAN_POINT('Ctrl Pts',(2.30590808156405,1.9402184231086,14.3036284089866));
#25468=CARTESIAN_POINT('Ctrl Pts',(2.30590826286364,1.94021745175103,14.3036307539451));
#25469=CARTESIAN_POINT('Ctrl Pts',(2.30836247613272,1.92706839443353,14.3353739497992));
#25470=CARTESIAN_POINT('Ctrl Pts',(2.31081669685968,1.91315083832213,14.3668017108966));
#25471=CARTESIAN_POINT('Ctrl Pts',(2.31327090916692,1.89845915781642,14.397860772894));
#25472=CARTESIAN_POINT('Ctrl Pts',(2.31327108900851,1.89845808122856,14.397863048863));
#25473=CARTESIAN_POINT('Ctrl Pts',(2.3132712688501,1.89845700463654,14.39786532483));
#25474=CARTESIAN_POINT('Ctrl Pts',(2.31327144869169,1.89845592804037,14.397867600795));
#25475=CARTESIAN_POINT('Ctrl Pts',(2.33536062905591,1.76622218206149,14.6774147398563));
#25476=CARTESIAN_POINT('Ctrl Pts',(2.3574491272971,1.5712727079731,14.9270944739197));
#25477=CARTESIAN_POINT('Ctrl Pts',(2.37953812370172,1.33229823339003,15.1233059771142));
#25478=CARTESIAN_POINT('Ctrl Pts',(2.37953847242699,1.33229446063208,15.1233090747609));
#25479=CARTESIAN_POINT('Ctrl Pts',(2.37953882115225,1.33229068786315,15.1233121723944));
#25480=CARTESIAN_POINT('Ctrl Pts',(2.37953916987752,1.33228691508325,15.1233152700145));
#25481=CARTESIAN_POINT('Ctrl Pts',(2.39619417790619,1.15210014392739,15.2712566242786));
#25482=CARTESIAN_POINT('Ctrl Pts',(2.41284942436104,0.946889344827322,15.3888028114828));
#25483=CARTESIAN_POINT('Ctrl Pts',(2.42950445771064,0.72822518719892,15.4697378980373));
#25484=CARTESIAN_POINT('Ctrl Pts',(-2.91746145426695,0.0017636091677427,
14.8994712573462));
#25485=CARTESIAN_POINT('Ctrl Pts',(-2.90019488125942,-0.159580608660099,
14.8996791954146));
#25486=CARTESIAN_POINT('Ctrl Pts',(-2.8657687140242,-0.480302096407746,
14.8438693373306));
#25487=CARTESIAN_POINT('Ctrl Pts',(-2.8019397152456,-1.00709100316185,14.5467293865288));
#25488=CARTESIAN_POINT('Ctrl Pts',(-2.73563696441919,-1.36578226769601,
14.010223019711));
#25489=CARTESIAN_POINT('Ctrl Pts',(-2.66693256929167,-1.42867373571422,
13.3592124992167));
#25490=CARTESIAN_POINT('Ctrl Pts',(-2.60311084828023,-1.25321990519817,
12.778393947455));
#25491=CARTESIAN_POINT('Ctrl Pts',(-2.53684614509442,-0.825318372599696,
12.3061946322186));
#25492=CARTESIAN_POINT('Ctrl Pts',(-2.4681235097376,-0.212191066831822,
12.069869359948));
#25493=CARTESIAN_POINT('Ctrl Pts',(-2.40430901915543,0.396119640741886,
12.114743545489));
#25494=CARTESIAN_POINT('Ctrl Pts',(-2.34049642694395,0.931518502467678,
12.4009672018237));
#25495=CARTESIAN_POINT('Ctrl Pts',(-2.29631706441142,1.19141144078301,12.7337364170638));
#25496=CARTESIAN_POINT('Ctrl Pts',(-2.27177360676358,1.2841798179601,12.9431797613183));
#25497=CARTESIAN_POINT('Ctrl Pts',(-2.24968444446761,1.36306447008945,13.1335712056504));
#25498=CARTESIAN_POINT('Ctrl Pts',(-2.23004927493927,1.3994922408639,13.3167047863868));
#25499=CARTESIAN_POINT('Ctrl Pts',(-2.20550563155682,1.39950586152936,13.5456943898369));
#25500=CARTESIAN_POINT('Ctrl Pts',(-2.1956882060897,1.39501224621372,13.6372896660342));
#25501=CARTESIAN_POINT('Ctrl Pts',(-2.1809619237048,1.37483761753456,13.7733623001193));
#25502=CARTESIAN_POINT('Ctrl Pts',(-2.16991730065325,1.34977676370599,13.8734411623136));
#25503=CARTESIAN_POINT('Ctrl Pts',(-2.16337230325175,1.33133763959568,13.9316592238358));
#25504=CARTESIAN_POINT('Ctrl Pts',(-2.15846356632158,1.31679708591878,13.9750876202867));
#25505=CARTESIAN_POINT('Ctrl Pts',(-2.15478201233856,1.30469358312819,14.0072528950141));
#25506=CARTESIAN_POINT('Ctrl Pts',(-2.12942019628186,1.21416701951389,14.2258649461565));
#25507=CARTESIAN_POINT('Ctrl Pts',(-2.08524154941588,0.971022892704046,
14.5711831154863));
#25508=CARTESIAN_POINT('Ctrl Pts',(-2.01897357959321,0.419779824527784,
14.8835182023753));
#25509=CARTESIAN_POINT('Ctrl Pts',(-1.95270560955346,-0.212032912475402,
14.930206696884));
#25510=CARTESIAN_POINT('Ctrl Pts',(-1.88889200873837,-0.781287448270816,
14.7105831133688));
#25511=CARTESIAN_POINT('Ctrl Pts',(-1.82753277730078,-1.19372337695382,
14.2978470446545));
#25512=CARTESIAN_POINT('Ctrl Pts',(-1.76371917662607,-1.42656061512116,
13.7370678108623));
#25513=CARTESIAN_POINT('Ctrl Pts',(-1.7048143142447,-1.39886856763557,13.1715868436166));
#25514=CARTESIAN_POINT('Ctrl Pts',(-1.65818129841028,-1.21018686470934,
12.7740536866313));
#25515=CARTESIAN_POINT('Ctrl Pts',(-1.63363760575663,-1.06902587007685,
12.5930469222915));
#25516=CARTESIAN_POINT('Ctrl Pts',(-1.62382012866622,-1.00584000033722,
12.5266849165902));
#25517=CARTESIAN_POINT('Ctrl Pts',(-1.61645702078024,-0.957269064068352,
12.4781046551932));
#25518=CARTESIAN_POINT('Ctrl Pts',(-1.60173080532553,-0.855349270287673,
12.3857391481269));
#25519=CARTESIAN_POINT('Ctrl Pts',(-1.56736963573534,-0.587573086682263,
12.2065836919316));
#25520=CARTESIAN_POINT('Ctrl Pts',(-1.51828225061532,-0.140924113539522,
12.0710241098653));
#25521=CARTESIAN_POINT('Ctrl Pts',(-1.45446864975801,0.463327639827352,
12.1303333085334));
#25522=CARTESIAN_POINT('Ctrl Pts',(-1.4102900030623,0.827632817053937,12.3483837391908));
#25523=CARTESIAN_POINT('Ctrl Pts',(-1.36856572560249,1.10294509845384,12.6236601489423));
#25524=CARTESIAN_POINT('Ctrl Pts',(-1.33420455599182,1.28984508344393,12.8895483365267));
#25525=CARTESIAN_POINT('Ctrl Pts',(-1.27039095511894,1.45237769519615,13.4721941418966));
#25526=CARTESIAN_POINT('Ctrl Pts',(-1.20657735438816,1.33125646100672,14.0812913187321));
#25527=CARTESIAN_POINT('Ctrl Pts',(-1.14276375353099,0.958199115373982,
14.5574728751379));
#25528=CARTESIAN_POINT('Ctrl Pts',(-1.10840258391648,0.683783826603428,
14.7315587417309));
#25529=CARTESIAN_POINT('Ctrl Pts',(-1.06176956797103,0.281828004010735,
14.8984788199422));
#25530=CARTESIAN_POINT('Ctrl Pts',(-1.01759092122265,-0.146042922087093,
14.9400333797164));
#25531=CARTESIAN_POINT('Ctrl Pts',(-0.958686059061629,-0.669259334769407,
14.7519920373476));
#25532=CARTESIAN_POINT('Ctrl Pts',(-0.929233627848142,-0.892353263312432,
14.5868188755852));
#25533=CARTESIAN_POINT('Ctrl Pts',(-0.894872458265258,-1.11905952818674,
14.3601151929184));
#25534=CARTESIAN_POINT('Ctrl Pts',(-0.875237504264326,-1.22280109179422,
14.2048833087194));
#25535=CARTESIAN_POINT('Ctrl Pts',(-0.850693811484429,-1.31044387511483,
13.9933309242246));
#25536=CARTESIAN_POINT('Ctrl Pts',(-0.843330703622131,-1.33362477081705,
13.9285726569875));
#25537=CARTESIAN_POINT('Ctrl Pts',(-0.828604488330937,-1.37027511219623,
13.796120759091));
#25538=CARTESIAN_POINT('Ctrl Pts',(-0.799152057004847,-1.41755272872254,
13.5246365146694));
#25539=CARTESIAN_POINT('Ctrl Pts',(-0.762336518301005,-1.38321876804832,
13.1762297382245));
#25540=CARTESIAN_POINT('Ctrl Pts',(-0.723066610044072,-1.24219377380554,
12.8361031544499));
#25541=CARTESIAN_POINT('Ctrl Pts',(-0.698522917480207,-1.11442727944758,
12.6447694003354));
#25542=CARTESIAN_POINT('Ctrl Pts',(-0.683796701920851,-1.022035166451,12.5428438921579));
#25543=CARTESIAN_POINT('Ctrl Pts',(-0.669070486267723,-0.924892975936484,
12.4456842991101));
#25544=CARTESIAN_POINT('Ctrl Pts',(-0.649435532212222,-0.782612198906497,
12.3288629646018));
#25545=CARTESIAN_POINT('Ctrl Pts',(-0.629800578134346,-0.620272858103612,
12.2421298000267));
#25546=CARTESIAN_POINT('Ctrl Pts',(-0.590530669970707,-0.281835429088842,
12.1015329289278));
#25547=CARTESIAN_POINT('Ctrl Pts',(-0.543897653950655,0.169856841999108,
12.057714018699));
#25548=CARTESIAN_POINT('Ctrl Pts',(-0.480084053153129,0.733743693002342,
12.2759770805796));
#25549=CARTESIAN_POINT('Ctrl Pts',(-0.430996667965097,1.08563450897863,
12.5792117928079));
#25550=CARTESIAN_POINT('Ctrl Pts',(-0.399089867586218,1.24033965540433,
12.8374730527932));
#25551=CARTESIAN_POINT('Ctrl Pts',(-0.369637436543767,1.34551709542376,
13.0913163915541));
#25552=CARTESIAN_POINT('Ctrl Pts',(-0.345093743843038,1.40174956442927,
13.3158597093218));
#25553=CARTESIAN_POINT('Ctrl Pts',(-0.315641312775735,1.4017190298085,13.5919825333234));
#25554=CARTESIAN_POINT('Ctrl Pts',(-0.291097620067433,1.36810137257278,
13.8187677293287));
#25555=CARTESIAN_POINT('Ctrl Pts',(-0.276371404600847,1.32804594187603,
13.9508899624769));
#25556=CARTESIAN_POINT('Ctrl Pts',(-0.264099558306616,1.28423821565556,
14.0566727881033));
#25557=CARTESIAN_POINT('Ctrl Pts',(-0.259190819742416,1.26567732595888,
14.0985563199077));
#25558=CARTESIAN_POINT('Ctrl Pts',(-0.249373342517745,1.2244866667904,14.1803979865844));
#25559=CARTESIAN_POINT('Ctrl Pts',(-0.232192757856559,1.14200653059235,
14.3180724570658));
#25560=CARTESIAN_POINT('Ctrl Pts',(-0.217466542354616,1.05441689387111,
14.4247877087319));
#25561=CARTESIAN_POINT('Ctrl Pts',(-0.180651003477795,0.811713222933898,
14.6678575357953));
#25562=CARTESIAN_POINT('Ctrl Pts',(-0.126654879772195,0.357076873077649,
14.9251932675087));
#25563=CARTESIAN_POINT('Ctrl Pts',(-0.0432063248173501,-0.45011407660554,
14.9055610385193));
#25564=CARTESIAN_POINT('Ctrl Pts',(0.0476053377514023,-1.1866456835083,
14.4144219839806));
#25565=CARTESIAN_POINT('Ctrl Pts',(0.111418938619706,-1.39997507961811,
13.8207407870374));
#25566=CARTESIAN_POINT('Ctrl Pts',(0.180141277840581,-1.40002079011879,
13.1794589876531));
#25567=CARTESIAN_POINT('Ctrl Pts',(0.243954878721026,-1.18677621847386,
12.5857475948577));
#25568=CARTESIAN_POINT('Ctrl Pts',(0.33476654126412,-0.450314644322968,
12.0945038436987));
#25569=CARTESIAN_POINT('Ctrl Pts',(0.418215096253102,0.356872553823869,
12.0747577299328));
#25570=CARTESIAN_POINT('Ctrl Pts',(0.472211219947981,0.81154531020039,12.3320292976198));
#25571=CARTESIAN_POINT('Ctrl Pts',(0.509026758783489,1.05428248464001,12.5750655439176));
#25572=CARTESIAN_POINT('Ctrl Pts',(0.521298605036259,1.12728903261987,12.6639834235209));
#25573=CARTESIAN_POINT('Ctrl Pts',(0.536024820681476,1.2008160076927,12.7800981181811));
#25574=CARTESIAN_POINT('Ctrl Pts',(0.545842297501875,1.24598447329656,12.8598136192458));
#25575=CARTESIAN_POINT('Ctrl Pts',(0.55320540537187,1.27539462490051,12.9219898354186));
#25576=CARTESIAN_POINT('Ctrl Pts',(0.563022882570486,1.31045155162959,13.0066113374631));
#25577=CARTESIAN_POINT('Ctrl Pts',(0.577749098072713,1.35681484657344,13.1361256281581));
#25578=CARTESIAN_POINT('Ctrl Pts',(0.602292790807561,1.40170777207648,13.3617946126849));
#25579=CARTESIAN_POINT('Ctrl Pts',(0.6366539602946,1.4017668435254,13.6839400854214));
#25580=CARTESIAN_POINT('Ctrl Pts',(0.661197653004655,1.3455774953339,13.9084907361462));
#25581=CARTESIAN_POINT('Ctrl Pts',(0.69065008405075,1.24043476680437,14.1623493334017));
#25582=CARTESIAN_POINT('Ctrl Pts',(0.722556884425975,1.08576652175257,14.420632835335));
#25583=CARTESIAN_POINT('Ctrl Pts',(0.771644269613912,0.733918423823554,
14.7239179023662));
#25584=CARTESIAN_POINT('Ctrl Pts',(0.835457870411991,0.170062504683883,
14.9422614843921));
#25585=CARTESIAN_POINT('Ctrl Pts',(0.882090886436469,-0.281636142740509,
14.8985069783426));
#25586=CARTESIAN_POINT('Ctrl Pts',(0.921360794598973,-0.620093629397158,
14.7579583436346));
#25587=CARTESIAN_POINT('Ctrl Pts',(0.940995748673728,-0.78244533749354,
14.6712483123915));
#25588=CARTESIAN_POINT('Ctrl Pts',(0.960630702731577,-0.924742763084939,
14.5544472535077));
#25589=CARTESIAN_POINT('Ctrl Pts',(0.975356918382398,-1.02189879158319,
14.4573014979626));
#25590=CARTESIAN_POINT('Ctrl Pts',(0.990083133939201,-1.11430541824352,
14.3553891484536));
#25591=CARTESIAN_POINT('Ctrl Pts',(1.01462682652934,-1.2420991675918,14.1640736023963));
#25592=CARTESIAN_POINT('Ctrl Pts',(1.05389673473115,-1.3831725908153,13.8239671087647));
#25593=CARTESIAN_POINT('Ctrl Pts',(1.09071227348601,-1.41755618749819,13.4755652595451));
#25594=CARTESIAN_POINT('Ctrl Pts',(1.12016470478803,-1.37031722480694,13.2040742906169));
#25595=CARTESIAN_POINT('Ctrl Pts',(1.13489092008799,-1.3336857405026,13.0716171771824));
#25596=CARTESIAN_POINT('Ctrl Pts',(1.14225402794831,-1.31051406497217,13.0068556110899));
#25597=CARTESIAN_POINT('Ctrl Pts',(1.16679772072381,-1.22290140273311,12.7952907540047));
#25598=CARTESIAN_POINT('Ctrl Pts',(1.1864326747268,-1.11918194748711,12.6400441106599));
#25599=CARTESIAN_POINT('Ctrl Pts',(1.2207938443113,-0.892507962849632,12.4133081589902));
#25600=CARTESIAN_POINT('Ctrl Pts',(1.25024627552374,-0.669437554782479,
12.2481032416591));
#25601=CARTESIAN_POINT('Ctrl Pts',(1.3091511376846,-0.146247920258923,12.0599874179223));
#25602=CARTESIAN_POINT('Ctrl Pts',(1.35332978443315,0.281628913559978,12.1014810662009));
#25603=CARTESIAN_POINT('Ctrl Pts',(1.39996280037785,0.683608494465903,12.268343919929));
#25604=CARTESIAN_POINT('Ctrl Pts',(1.43432396999435,0.958048563093325,12.442390719136));
#25605=CARTESIAN_POINT('Ctrl Pts',(1.4981375708502,1.33117369477561,12.9185191623767));
#25606=CARTESIAN_POINT('Ctrl Pts',(1.56195117158053,1.45238164110855,13.5275990903951));
#25607=CARTESIAN_POINT('Ctrl Pts',(1.62576477245543,1.28993197840348,14.1102680289494));
#25608=CARTESIAN_POINT('Ctrl Pts',(1.66012594206798,1.10306984876638,14.3761828219785));
#25609=CARTESIAN_POINT('Ctrl Pts',(1.70185021952445,0.827796759986248,14.6514984236658));
#25610=CARTESIAN_POINT('Ctrl Pts',(1.74602886622133,0.463522631126779,14.8696007159398));
#25611=CARTESIAN_POINT('Ctrl Pts',(1.80984246707339,-0.1407206716199,14.9289959381943));
#25612=CARTESIAN_POINT('Ctrl Pts',(1.85892985219695,-0.587388936191916,
14.7934999445719));
#25613=CARTESIAN_POINT('Ctrl Pts',(1.8932910217891,-0.855190621007161,14.6143826120952));
#25614=CARTESIAN_POINT('Ctrl Pts',(1.90801723724395,-0.95712356280611,14.5220316155655));
#25615=CARTESIAN_POINT('Ctrl Pts',(1.91538034513003,-1.00570141455371,14.4734582694652));
#25616=CARTESIAN_POINT('Ctrl Pts',(1.92519782222027,-1.06889673120442,14.4071052598134));
#25617=CARTESIAN_POINT('Ctrl Pts',(1.94974151487335,-1.21008349176762,14.2261185936406));
#25618=CARTESIAN_POINT('Ctrl Pts',(1.99637453070844,-1.39882177721573,13.8286123034665));
#25619=CARTESIAN_POINT('Ctrl Pts',(2.05527939308903,-1.42659432214954,13.2631352856935));
#25620=CARTESIAN_POINT('Ctrl Pts',(2.11909299376731,-1.19383689080884,12.7023229120511));
#25621=CARTESIAN_POINT('Ctrl Pts',(2.18045222520523,-0.781459684572717,
12.2895281354887));
#25622=CARTESIAN_POINT('Ctrl Pts',(2.24426582602376,-0.212236361467477,
12.0698235172568));
#25623=CARTESIAN_POINT('Ctrl Pts',(2.31053379607291,0.419583147593255,12.1164220761731));
#25624=CARTESIAN_POINT('Ctrl Pts',(2.37680176589273,0.970870796055125,12.4286786933557));
#25625=CARTESIAN_POINT('Ctrl Pts',(2.42098041277556,1.21406435463139,12.7739622687326));
#25626=CARTESIAN_POINT('Ctrl Pts',(2.44634222883891,1.30462209891747,12.9925614349691));
#25627=CARTESIAN_POINT('Ctrl Pts',(2.4500237828227,1.31673018620759,13.0247249870419));
#25628=CARTESIAN_POINT('Ctrl Pts',(2.45493251975282,1.33127691935092,13.0681513140835));
#25629=CARTESIAN_POINT('Ctrl Pts',(2.46147751715357,1.34972436758129,13.1263667423369));
#25630=CARTESIAN_POINT('Ctrl Pts',(2.47252214020686,1.37479942108684,13.2264420569245));
#25631=CARTESIAN_POINT('Ctrl Pts',(2.48724842259595,1.39499363824062,13.3625117988546));
#25632=CARTESIAN_POINT('Ctrl Pts',(2.49706584806392,1.39950021010734,13.4541064541347));
#25633=CARTESIAN_POINT('Ctrl Pts',(2.52160949145431,1.39951926866424,13.6830960638344));
#25634=CARTESIAN_POINT('Ctrl Pts',(2.54124466103345,1.3631190589702,13.8662350598753));
#25635=CARTESIAN_POINT('Ctrl Pts',(2.56333382333658,1.2842613255101,14.0566376252996));
#25636=CARTESIAN_POINT('Ctrl Pts',(2.58787728099126,1.19152225787391,14.2660936889693));
#25637=CARTESIAN_POINT('Ctrl Pts',(2.63205664366046,0.931682750775297,14.5989038479848));
#25638=CARTESIAN_POINT('Ctrl Pts',(2.69586923597156,0.396320608623301,14.8851965578387));
#25639=CARTESIAN_POINT('Ctrl Pts',(2.75968372689716,-0.211964411383521,
14.9301722674985));
#25640=CARTESIAN_POINT('Ctrl Pts',(2.82840636255072,-0.825146742340399,
14.6939085236109));
#25641=CARTESIAN_POINT('Ctrl Pts',(2.89467106680061,-1.25302913630202,14.221827888447));
#25642=CARTESIAN_POINT('Ctrl Pts',(2.95849278830799,-1.42868057472017,13.6409334123114));
#25643=CARTESIAN_POINT('Ctrl Pts',(3.02719718612572,-1.36551532321063,12.9901843349406));
#25644=CARTESIAN_POINT('Ctrl Pts',(3.0805160037115,-1.07762573723313,12.55826580189));
#25645=CARTESIAN_POINT('Ctrl Pts',(3.11415879661038,-0.826194988464377,
12.3697490786105));
#25646=CARTESIAN_POINT('Ctrl Pts',(3.11836033000717,-0.79392026024566,12.3475163248423));
#25647=CARTESIAN_POINT('Ctrl Pts',(-3.00252836970136,0.00205538494515771,
15.1331908023729));
#25648=CARTESIAN_POINT('Ctrl Pts',(-2.98527982013788,-0.185981147804069,
15.1334545181963));
#25649=CARTESIAN_POINT('Ctrl Pts',(-2.95085538393473,-0.560235514350509,
15.0684314612154));
#25650=CARTESIAN_POINT('Ctrl Pts',(-2.88698949839108,-1.17552199967255,
14.7213621162832));
#25651=CARTESIAN_POINT('Ctrl Pts',(-2.82071377950267,-1.59379469789951,
14.0955052168205));
#25652=CARTESIAN_POINT('Ctrl Pts',(-2.75199539264616,-1.66728946021813,
13.3356189189095));
#25653=CARTESIAN_POINT('Ctrl Pts',(-2.68817998979099,-1.46249020257107,
12.6578747738934));
#25654=CARTESIAN_POINT('Ctrl Pts',(-2.62191274641039,-0.963128682093589,
12.1067915533372));
#25655=CARTESIAN_POINT('Ctrl Pts',(-2.5531903417797,-0.247577521527219,
11.8310330526963));
#25656=CARTESIAN_POINT('Ctrl Pts',(-2.48937654342735,0.462308854742993,
11.8833961450926));
#25657=CARTESIAN_POINT('Ctrl Pts',(-2.42556316698634,1.08711300487288,12.2174675831258));
#25658=CARTESIAN_POINT('Ctrl Pts',(-2.38138436118434,1.39043544977562,12.6057667639547));
#25659=CARTESIAN_POINT('Ctrl Pts',(-2.3568407207863,1.49864818055694,12.8502306958011));
#25660=CARTESIAN_POINT('Ctrl Pts',(-2.33475143321486,1.59075305876895,13.072392949461));
#25661=CARTESIAN_POINT('Ctrl Pts',(-2.31511643129009,1.63320798368394,13.2861490673466));
#25662=CARTESIAN_POINT('Ctrl Pts',(-2.29057274957865,1.63322634504617,13.553361932451));
#25663=CARTESIAN_POINT('Ctrl Pts',(-2.28075528400572,1.62797785312041,13.660259932391));
#25664=CARTESIAN_POINT('Ctrl Pts',(-2.26602905363386,1.60443102075799,13.8190521615535));
#25665=CARTESIAN_POINT('Ctrl Pts',(-2.25498440062962,1.57518246629865,13.9358468917031));
#25666=CARTESIAN_POINT('Ctrl Pts',(-2.24843941314017,1.55366106765359,14.0037857560899));
#25667=CARTESIAN_POINT('Ctrl Pts',(-2.24353067492705,1.53669419003256,14.0544676889874));
#25668=CARTESIAN_POINT('Ctrl Pts',(-2.23984912098126,1.52256174880168,14.0920025777527));
#25669=CARTESIAN_POINT('Ctrl Pts',(-2.21448730515743,1.41694703492178,14.3471327348479));
#25670=CARTESIAN_POINT('Ctrl Pts',(-2.17030865839431,1.13314767767377,14.7501030896063));
#25671=CARTESIAN_POINT('Ctrl Pts',(-2.10404068838079,0.48985529256926,15.1145875274289));
#25672=CARTESIAN_POINT('Ctrl Pts',(-2.03777271837396,-0.247486882538813,
15.1690540813149));
#25673=CARTESIAN_POINT('Ctrl Pts',(-1.97395911763629,-0.911798832807848,
14.9127364048317));
#25674=CARTESIAN_POINT('Ctrl Pts',(-1.91259988616224,-1.39310996057585,
14.4310578285023));
#25675=CARTESIAN_POINT('Ctrl Pts',(-1.84878628545668,-1.66479795157223,
13.7766219771277));
#25676=CARTESIAN_POINT('Ctrl Pts',(-1.78988142317389,-1.63248593599747,
13.1166990702497));
#25677=CARTESIAN_POINT('Ctrl Pts',(-1.74324840727158,-1.41224995598874,
12.6527853330733));
#25678=CARTESIAN_POINT('Ctrl Pts',(-1.71870471460997,-1.24755228455272,
12.4415496621475));
#25679=CARTESIAN_POINT('Ctrl Pts',(-1.70888723755622,-1.17378817419318,
12.3641095389944));
#25680=CARTESIAN_POINT('Ctrl Pts',(-1.70152412968286,-1.11711290300786,
12.30741090743));
#25681=CARTESIAN_POINT('Ctrl Pts',(-1.68679791418894,-0.998163120888784,
12.1996368857678));
#25682=CARTESIAN_POINT('Ctrl Pts',(-1.6524367445998,-0.685665906795594,
11.9905518057572));
#25683=CARTESIAN_POINT('Ctrl Pts',(-1.60334935950164,-0.164421556499146,
11.8323643050256));
#25684=CARTESIAN_POINT('Ctrl Pts',(-1.53953575865813,0.540747957468112,
11.901617685449));
#25685=CARTESIAN_POINT('Ctrl Pts',(-1.49535711192252,0.965883684423983,
12.1560379983072));
#25686=CARTESIAN_POINT('Ctrl Pts',(-1.4536328344594,1.28717780938966,12.4773646847382));
#25687=CARTESIAN_POINT('Ctrl Pts',(-1.41927166486658,1.50525376566623,12.7876189220491));
#25688=CARTESIAN_POINT('Ctrl Pts',(-1.35545806402325,1.69493846692438,13.4676051398953));
#25689=CARTESIAN_POINT('Ctrl Pts',(-1.29164446321183,1.55357584047738,14.1783939299935));
#25690=CARTESIAN_POINT('Ctrl Pts',(-1.22783086237105,1.11817335073225,14.734117053682));
#25691=CARTESIAN_POINT('Ctrl Pts',(-1.19346969277715,0.797965353074917,
14.9372224500198));
#25692=CARTESIAN_POINT('Ctrl Pts',(-1.14683667684874,0.328840193056562,
15.1320794625458));
#25693=CARTESIAN_POINT('Ctrl Pts',(-1.10265803009968,-0.170461188953638,
15.1805232343716));
#25694=CARTESIAN_POINT('Ctrl Pts',(-1.04375316786571,-0.781072783835267,
14.9610508385942));
#25695=CARTESIAN_POINT('Ctrl Pts',(-1.01430073671879,-1.04140710776821,
14.7683279748065));
#25696=CARTESIAN_POINT('Ctrl Pts',(-0.979939567130956,-1.30597646868345,
14.5036867373158));
#25697=CARTESIAN_POINT('Ctrl Pts',(-0.960304613064202,-1.4270605691062,
14.3226287109822));
#25698=CARTESIAN_POINT('Ctrl Pts',(-0.935760920374095,-1.52930100872486,
14.0756739209351));
#25699=CARTESIAN_POINT('Ctrl Pts',(-0.928397812551484,-1.55636742199646,
14.0001138510484));
#25700=CARTESIAN_POINT('Ctrl Pts',(-0.913671597093866,-1.59911265933892,
13.8455369235439));
#25701=CARTESIAN_POINT('Ctrl Pts',(-0.88421916601447,-1.65431209129421,
13.5287124742323));
#25702=CARTESIAN_POINT('Ctrl Pts',(-0.847403627128462,-1.61421626509089,
13.1221241103553));
#25703=CARTESIAN_POINT('Ctrl Pts',(-0.808133718938854,-1.44962467809318,
12.7251977888485));
#25704=CARTESIAN_POINT('Ctrl Pts',(-0.78359002629623,-1.30052263608422,
12.5019186100426));
#25705=CARTESIAN_POINT('Ctrl Pts',(-0.76886381077922,-1.19269127101649,
12.3829668682071));
#25706=CARTESIAN_POINT('Ctrl Pts',(-0.754137595149626,-1.07932525044337,
12.2696043978058));
#25707=CARTESIAN_POINT('Ctrl Pts',(-0.734502641072207,-0.913282101181525,
12.1332231457686));
#25708=CARTESIAN_POINT('Ctrl Pts',(-0.714867686988017,-0.723821617740119,
12.0320856016891));
#25709=CARTESIAN_POINT('Ctrl Pts',(-0.675597778820173,-0.32887384745749,
11.8678982144759));
#25710=CARTESIAN_POINT('Ctrl Pts',(-0.628964762829318,0.19826785403632,
11.8168787027133));
#25711=CARTESIAN_POINT('Ctrl Pts',(-0.565151162002638,0.856314278625342,
12.0715613404292));
#25712=CARTESIAN_POINT('Ctrl Pts',(-0.516063776796385,1.2669674670857,12.4254554520173));
#25713=CARTESIAN_POINT('Ctrl Pts',(-0.484156976433268,1.44749830932253,
12.7268633891509));
#25714=CARTESIAN_POINT('Ctrl Pts',(-0.454704545415558,1.57023839812038,
13.0230879375965));
#25715=CARTESIAN_POINT('Ctrl Pts',(-0.430160852743294,1.63585223537756,
13.285143483846));
#25716=CARTESIAN_POINT('Ctrl Pts',(-0.400708421628965,1.63580953116395,
13.6073742665564));
#25717=CARTESIAN_POINT('Ctrl Pts',(-0.376164728954184,1.59657052806564,
13.8720348170695));
#25718=CARTESIAN_POINT('Ctrl Pts',(-0.361438513458364,1.54982470601694,
14.026220050662));
#25719=CARTESIAN_POINT('Ctrl Pts',(-0.349166667134025,1.49869362646351,
14.1496661593144));
#25720=CARTESIAN_POINT('Ctrl Pts',(-0.344257928557389,1.4770370638121,14.1985479979232));
#25721=CARTESIAN_POINT('Ctrl Pts',(-0.334440451474348,1.42895428828331,
14.2940474291423));
#25722=CARTESIAN_POINT('Ctrl Pts',(-0.317259866709618,1.332717968861,14.4547305965666));
#25723=CARTESIAN_POINT('Ctrl Pts',(-0.302533651204796,1.23046378536219,
14.5792352145037));
#25724=CARTESIAN_POINT('Ctrl Pts',(-0.26571811232627,0.947273180307621,
14.86293984835));
#25725=CARTESIAN_POINT('Ctrl Pts',(-0.211721988644085,0.416651601106899,
15.1631715574816));
#25726=CARTESIAN_POINT('Ctrl Pts',(-0.128273433716417,-0.525303820823094,
15.1403331888213));
#25727=CARTESIAN_POINT('Ctrl Pts',(-0.0374617710681013,-1.38485327505203,
14.5670907032476));
#25728=CARTESIAN_POINT('Ctrl Pts',(0.0263518297750454,-1.63379435128198,
13.8742842613791));
#25729=CARTESIAN_POINT('Ctrl Pts',(0.0950741689632889,-1.63382972703326,
13.1258710146013));
#25730=CARTESIAN_POINT('Ctrl Pts',(0.158887769808821,-1.38495508123797,
12.4330413982481));
#25731=CARTESIAN_POINT('Ctrl Pts',(0.249699432452321,-0.52545935207591,
11.8597170827633));
#25732=CARTESIAN_POINT('Ctrl Pts',(0.333147987387138,0.416491690732399,
11.8367914807877));
#25733=CARTESIAN_POINT('Ctrl Pts',(0.387144111066703,0.947143527898697,
12.1369717461611));
#25734=CARTESIAN_POINT('Ctrl Pts',(0.423959649936313,1.23035674071828,12.4206532587168));
#25735=CARTESIAN_POINT('Ctrl Pts',(0.436231496205733,1.31559067564619,12.5243893912344));
#25736=CARTESIAN_POINT('Ctrl Pts',(0.450957711741397,1.4013704881953,12.6599178389611));
#25737=CARTESIAN_POINT('Ctrl Pts',(0.4607751887345,1.45409117498363,12.7529378493789));
#25738=CARTESIAN_POINT('Ctrl Pts',(0.468138296558858,1.48840440040474,12.8255047097806));
#25739=CARTESIAN_POINT('Ctrl Pts',(0.477955773727791,1.52931520386143,12.9242574281315));
#25740=CARTESIAN_POINT('Ctrl Pts',(0.492681989231907,1.58341885399309,13.0754019220946));
#25741=CARTESIAN_POINT('Ctrl Pts',(0.51722568191251,1.6358025154813,13.3387617413545));
#25742=CARTESIAN_POINT('Ctrl Pts',(0.551586851479718,1.6358622587284,13.7147015657294));
#25743=CARTESIAN_POINT('Ctrl Pts',(0.576130544154049,1.57028636551549,13.9767616281306));
#25744=CARTESIAN_POINT('Ctrl Pts',(0.605582975172473,1.44757211442134,14.272998526345));
#25745=CARTESIAN_POINT('Ctrl Pts',(0.637489775533693,1.26707042745046,14.5744235528787));
#25746=CARTESIAN_POINT('Ctrl Pts',(0.686577160741821,0.856450056310684,
14.9283569884486));
#25747=CARTESIAN_POINT('Ctrl Pts',(0.750390761567867,0.198427790429692,
15.1831021639917));
#25748=CARTESIAN_POINT('Ctrl Pts',(0.797023777559325,-0.328719012736018,
15.1321327619175));
#25749=CARTESIAN_POINT('Ctrl Pts',(0.83629368572729,-0.723682311592208,
14.9679828445898));
#25750=CARTESIAN_POINT('Ctrl Pts',(0.85592863981007,-0.913152446732621,
14.8668632900606));
#25751=CARTESIAN_POINT('Ctrl Pts',(0.875563593888921,-1.07920850799294,
14.7304977869275));
#25752=CARTESIAN_POINT('Ctrl Pts',(0.890289809517802,-1.19258529192622,
14.6171460730064));
#25753=CARTESIAN_POINT('Ctrl Pts',(0.905016025034186,-1.30042793054723,
14.4982045532945));
#25754=CARTESIAN_POINT('Ctrl Pts',(0.929559717682546,-1.44955115512858,
14.2749395277779));
#25755=CARTESIAN_POINT('Ctrl Pts',(0.968829625859914,-1.61418037039209,
13.8780288156127));
#25756=CARTESIAN_POINT('Ctrl Pts',(1.00564516475731,-1.65431477124166,13.4714442854307));
#25757=CARTESIAN_POINT('Ctrl Pts',(1.03509759583151,-1.59914537217458,13.1546146181273));
#25758=CARTESIAN_POINT('Ctrl Pts',(1.04982381129091,-1.55641478567852,13.0000336344831));
#25759=CARTESIAN_POINT('Ctrl Pts',(1.0571869191131,-1.52935553879155,12.9244710046119));
#25760=CARTESIAN_POINT('Ctrl Pts',(1.08173061180252,-1.42713848945209,12.6775065180917));
#25761=CARTESIAN_POINT('Ctrl Pts',(1.10136556586942,-1.30607158736917,12.4964370303868));
#25762=CARTESIAN_POINT('Ctrl Pts',(1.13572673545794,-1.04152729433169,12.2317707234624));
#25763=CARTESIAN_POINT('Ctrl Pts',(1.16517916660448,-0.781211253495427,
12.0390231851748));
#25764=CARTESIAN_POINT('Ctrl Pts',(1.22408402883849,-0.170620462432981,
11.8194929249613));
#25765=CARTESIAN_POINT('Ctrl Pts',(1.26826267558795,0.328685516234155,11.8678893662407));
#25766=CARTESIAN_POINT('Ctrl Pts',(1.31489569151535,0.79782912167651,12.0627019246719));
#25767=CARTESIAN_POINT('Ctrl Pts',(1.34925686111136,1.11805638087561,12.2657769596875));
#25768=CARTESIAN_POINT('Ctrl Pts',(1.41307046195049,1.55351153230628,12.8214588224151));
#25769=CARTESIAN_POINT('Ctrl Pts',(1.47688406276225,1.69494153596926,13.532234210352));
#25770=CARTESIAN_POINT('Ctrl Pts',(1.54069766360644,1.50532127692099,14.2122383972142));
#25771=CARTESIAN_POINT('Ctrl Pts',(1.5750588332008,1.28727474124243,14.5225133116529));
#25772=CARTESIAN_POINT('Ctrl Pts',(1.61678311066043,0.966011054182616,14.8438704467015));
#25773=CARTESIAN_POINT('Ctrl Pts',(1.66096175739847,0.540899461717136,15.0983310548197));
#25774=CARTESIAN_POINT('Ctrl Pts',(1.72477535823702,-0.164263490526999,
15.1676512711812));
#25775=CARTESIAN_POINT('Ctrl Pts',(1.77386274333832,-0.685522828652171,
15.0095131764614));
#25776=CARTESIAN_POINT('Ctrl Pts',(1.80822391292843,-0.998039852607216,
14.8004577179364));
#25777=CARTESIAN_POINT('Ctrl Pts',(1.82295012842216,-1.11699985285216,14.6926949691893));
#25778=CARTESIAN_POINT('Ctrl Pts',(1.83031323629589,-1.17368049582136,14.6360017121857));
#25779=CARTESIAN_POINT('Ctrl Pts',(1.84013071334923,-1.24745194660516,14.5585685740192));
#25780=CARTESIAN_POINT('Ctrl Pts',(1.86467440601124,-1.41216963612087,14.3473485268086));
#25781=CARTESIAN_POINT('Ctrl Pts',(1.91130742191433,-1.63244957724005,13.8834556582109));
#25782=CARTESIAN_POINT('Ctrl Pts',(1.97021228419637,-1.66482413385211,13.2235358241412));
#25783=CARTESIAN_POINT('Ctrl Pts',(2.03402588490596,-1.39319814356631,12.5690742212523));
#25784=CARTESIAN_POINT('Ctrl Pts',(2.09538511638032,-0.911932631418002,
12.0873500335917));
#25785=CARTESIAN_POINT('Ctrl Pts',(2.15919871712108,-0.247644919118781,
11.8309693962473));
#25786=CARTESIAN_POINT('Ctrl Pts',(2.2254666871376,0.489702547485788,11.8853660789399));
#25787=CARTESIAN_POINT('Ctrl Pts',(2.29173465714865,1.13302959529792,12.2497895468869));
#25788=CARTESIAN_POINT('Ctrl Pts',(2.33591330392835,1.41686742328557,12.6527330373133));
#25789=CARTESIAN_POINT('Ctrl Pts',(2.36127511975716,1.52250637166547,12.9078531761878));
#25790=CARTESIAN_POINT('Ctrl Pts',(2.36495667370317,1.53664238670787,12.9453867337541));
#25791=CARTESIAN_POINT('Ctrl Pts',(2.36986541191653,1.5536140512705,12.9960670500936));
#25792=CARTESIAN_POINT('Ctrl Pts',(2.37641039940547,1.57514194868161,13.0640038860603));
#25793=CARTESIAN_POINT('Ctrl Pts',(2.38745505241297,1.60440147660552,13.1807958197083));
#25794=CARTESIAN_POINT('Ctrl Pts',(2.40218128278599,1.62796365750789,13.3395858727675));
#25795=CARTESIAN_POINT('Ctrl Pts',(2.41199874836342,1.63322205640795,13.4464832900758));
#25796=CARTESIAN_POINT('Ctrl Pts',(2.43654243007502,1.63322976252623,13.7136965402967));
#25797=CARTESIAN_POINT('Ctrl Pts',(2.45617743206558,1.59079533728359,13.9274562422369));
#25798=CARTESIAN_POINT('Ctrl Pts',(2.4782667196338,1.49871212944699,14.1496275339613));
#25799=CARTESIAN_POINT('Ctrl Pts',(2.5028103600564,1.39052109086099,14.3941006888739));
#25800=CARTESIAN_POINT('Ctrl Pts',(2.54698916595512,1.08724369463858,14.7824338036398));
#25801=CARTESIAN_POINT('Ctrl Pts',(2.61080254255296,0.462464018280852,15.1165555131629));
#25802=CARTESIAN_POINT('Ctrl Pts',(2.67461634115977,-0.247393003196471,
15.1690039491515));
#25803=CARTESIAN_POINT('Ctrl Pts',(2.74333874625233,-0.963000910327539,
14.8932808228982));
#25804=CARTESIAN_POINT('Ctrl Pts',(2.80960599038935,-1.46231188778867,14.3423162383898));
#25805=CARTESIAN_POINT('Ctrl Pts',(2.87342139427634,-1.66731758164261,13.6644668612195));
#25806=CARTESIAN_POINT('Ctrl Pts',(2.9421397828027,-1.59347520441855,12.9048899504509));
#25807=CARTESIAN_POINT('Ctrl Pts',(2.99543686361548,-1.25774848826549,12.4010519912542));
#25808=CARTESIAN_POINT('Ctrl Pts',(3.02908986191469,-0.964147003153576,
12.1810042236116));
#25809=CARTESIAN_POINT('Ctrl Pts',(3.03329287307245,-0.92648238051196,12.1550256572553));
#25810=CARTESIAN_POINT('Ctrl Pts',(-3.08759528491809,0.0023500709696575,
15.3669112794954));
#25811=CARTESIAN_POINT('Ctrl Pts',(-3.070364778818,-0.212646371255907,15.3671449067253));
#25812=CARTESIAN_POINT('Ctrl Pts',(-3.03594205588516,-0.640224871273036,
15.2930636162465));
#25813=CARTESIAN_POINT('Ctrl Pts',(-2.97203928859788,-1.34405177464685,
14.8959035131867));
#25814=CARTESIAN_POINT('Ctrl Pts',(-2.90579059611891,-1.82179168220255,
14.180783442706));
#25815=CARTESIAN_POINT('Ctrl Pts',(-2.8370582186335,-1.90595073708206,13.3119961697794));
#25816=CARTESIAN_POINT('Ctrl Pts',(-2.77324913208513,-1.67174130404843,
12.5373404820452));
#25817=CARTESIAN_POINT('Ctrl Pts',(-2.70697934869721,-1.1009493781795,11.9073944503979));
#25818=CARTESIAN_POINT('Ctrl Pts',(-2.63825717411256,-0.282964643060395,
11.5921720805156));
#25819=CARTESIAN_POINT('Ctrl Pts',(-2.57444406802585,0.528477611992774,
11.6520800065705));
#25820=CARTESIAN_POINT('Ctrl Pts',(-2.51062990712246,1.24274101975633,12.0339183867967));
#25821=CARTESIAN_POINT('Ctrl Pts',(-2.46645165807834,1.58936201945163,12.4778870234411));
#25822=CARTESIAN_POINT('Ctrl Pts',(-2.44190783487501,1.71315248791266,12.7572594832551));
#25823=CARTESIAN_POINT('Ctrl Pts',(-2.41981842205487,1.8183263300599,13.0112815736336));
#25824=CARTESIAN_POINT('Ctrl Pts',(-2.40018358765284,1.86696052951785,13.255540997676));
#25825=CARTESIAN_POINT('Ctrl Pts',(-2.37563986763414,1.86695758479274,13.5610368182778));
#25826=CARTESIAN_POINT('Ctrl Pts',(-2.36582236194615,1.86095970736867,13.6832217734386));
#25827=CARTESIAN_POINT('Ctrl Pts',(-2.35109618359108,1.8340383937764,13.8647453356404));
#25828=CARTESIAN_POINT('Ctrl Pts',(-2.34005150062928,1.80060082651263,13.9982489249835));
#25829=CARTESIAN_POINT('Ctrl Pts',(-2.33350652305318,1.77600090529121,14.0759124271069));
#25830=CARTESIAN_POINT('Ctrl Pts',(-2.32859778355624,1.75659799293553,14.1338445204053));
#25831=CARTESIAN_POINT('Ctrl Pts',(-2.32491622964828,1.74045665369918,14.1767545198982));
#25832=CARTESIAN_POINT('Ctrl Pts',(-2.29955441405339,1.61964487367634,14.4683693759585));
#25833=CARTESIAN_POINT('Ctrl Pts',(-2.25537576737961,1.29530781396324,14.929025377181));
#25834=CARTESIAN_POINT('Ctrl Pts',(-2.18910779718202,0.559905905457109,
15.3456504769967));
#25835=CARTESIAN_POINT('Ctrl Pts',(-2.12283982719947,-0.282930359999273,
15.4078999941006));
#25836=CARTESIAN_POINT('Ctrl Pts',(-2.05902622653861,-1.04231549003814,
15.1148878618827));
#25837=CARTESIAN_POINT('Ctrl Pts',(-1.99766699502949,-1.59247938955606,
14.564272017216));
#25838=CARTESIAN_POINT('Ctrl Pts',(-1.93385339428798,-1.90307453898268,
13.8161699129123));
#25839=CARTESIAN_POINT('Ctrl Pts',(-1.87494853210476,-1.86608125873476,
13.0618174246178));
#25840=CARTESIAN_POINT('Ctrl Pts',(-1.82831551613341,-1.61438776389863,
12.5315095874762));
#25841=CARTESIAN_POINT('Ctrl Pts',(-1.80377182346193,-1.42602447023497,
12.2900559477824));
#25842=CARTESIAN_POINT('Ctrl Pts',(-1.79395434644624,-1.34175398647389,
12.201528824612));
#25843=CARTESIAN_POINT('Ctrl Pts',(-1.78659123858441,-1.27694850031384,
12.1367313966333));
#25844=CARTESIAN_POINT('Ctrl Pts',(-1.77186502305241,-1.14098738956333,
12.013506241682));
#25845=CARTESIAN_POINT('Ctrl Pts',(-1.7375038534634,-0.783756830443404,
11.7745426475921));
#25846=CARTESIAN_POINT('Ctrl Pts',(-1.68841646838521,-0.187913082298619,
11.5937304847702));
#25847=CARTESIAN_POINT('Ctrl Pts',(-1.62460286756024,0.61815658478922,11.6728608723269));
#25848=CARTESIAN_POINT('Ctrl Pts',(-1.58042422078084,1.10413623186327,11.9638185378979));
#25849=CARTESIAN_POINT('Ctrl Pts',(-1.53869994331994,1.47138001066433,12.3309861788527));
#25850=CARTESIAN_POINT('Ctrl Pts',(-1.50433877374192,1.72072186236973,12.6857382584471));
#25851=CARTESIAN_POINT('Ctrl Pts',(-1.44052517292936,1.93748562326409,13.4629729665557));
#25852=CARTESIAN_POINT('Ctrl Pts',(-1.37671157203573,1.77587122939508,14.2755365403217));
#25853=CARTESIAN_POINT('Ctrl Pts',(-1.31289797121347,1.27821103918419,14.910720784742));
#25854=CARTESIAN_POINT('Ctrl Pts',(-1.27853680163774,0.912087345431337,
15.1429840770779));
#25855=CARTESIAN_POINT('Ctrl Pts',(-1.23190378572754,0.37589996465958,15.3655639266512));
#25856=CARTESIAN_POINT('Ctrl Pts',(-1.18772513897687,-0.194914574603933,
15.4210130110031));
#25857=CARTESIAN_POINT('Ctrl Pts',(-1.12882027666981,-0.892860720439233,
15.1701471113649));
#25858=CARTESIAN_POINT('Ctrl Pts',(-1.09936784558967,-1.19047435017082,
14.9497506527899));
#25859=CARTESIAN_POINT('Ctrl Pts',(-1.06500667599683,-1.49288243745837,
14.6473828402657));
#25860=CARTESIAN_POINT('Ctrl Pts',(-1.04537172186518,-1.63124495617839,
14.440195073271));
#25861=CARTESIAN_POINT('Ctrl Pts',(-1.02082802926375,-1.74818285448208,
14.1580460636463));
#25862=CARTESIAN_POINT('Ctrl Pts',(-1.01346492148097,-1.77908694402207,
14.0716427230622));
#25863=CARTESIAN_POINT('Ctrl Pts',(-0.998738705857055,-1.82799370925915,
13.8949520830598));
#25864=CARTESIAN_POINT('Ctrl Pts',(-0.969286275024268,-1.89101395941206,
13.5327858149411));
#25865=CARTESIAN_POINT('Ctrl Pts',(-0.932470735954739,-1.84521085036033,
13.0680056680855));
#25866=CARTESIAN_POINT('Ctrl Pts',(-0.89320082783347,-1.65706813257767,
12.6142812638122));
#25867=CARTESIAN_POINT('Ctrl Pts',(-0.868657135111634,-1.48660805742424,
12.3590420738917));
#25868=CARTESIAN_POINT('Ctrl Pts',(-0.853930919637501,-1.36335663025442,
12.2230840215225));
#25869=CARTESIAN_POINT('Ctrl Pts',(-0.839204704031034,-1.23376026936314,
12.0934568578651));
#25870=CARTESIAN_POINT('Ctrl Pts',(-0.8195697499311,-1.04394701268137,11.9376775261929));
#25871=CARTESIAN_POINT('Ctrl Pts',(-0.7999347958418,-0.827386737992478,
11.8219078046918));
#25872=CARTESIAN_POINT('Ctrl Pts',(-0.760664887668704,-0.375884998960593,
11.6344876086694));
#25873=CARTESIAN_POINT('Ctrl Pts',(-0.714031871708202,0.226667196248288,
11.5759533828502));
#25874=CARTESIAN_POINT('Ctrl Pts',(-0.65021827085275,0.97889333543878,11.8671971878041));
#25875=CARTESIAN_POINT('Ctrl Pts',(-0.601130885626391,1.44829992606202,
12.2717276845478));
#25876=CARTESIAN_POINT('Ctrl Pts',(-0.569224085280087,1.65466780097147,
12.6162485693903));
#25877=CARTESIAN_POINT('Ctrl Pts',(-0.53977165428826,1.79495718711597,12.9548992928255));
#25878=CARTESIAN_POINT('Ctrl Pts',(-0.515227961643534,1.86996301017078,
13.2544352024425));
#25879=CARTESIAN_POINT('Ctrl Pts',(-0.485775530482349,1.86990635043761,
13.6227923522052));
#25880=CARTESIAN_POINT('Ctrl Pts',(-0.461231837841324,1.82504811787028,
13.9253227089901));
#25881=CARTESIAN_POINT('Ctrl Pts',(-0.446505622315567,1.77160362358178,
14.1015741272446));
#25882=CARTESIAN_POINT('Ctrl Pts',(-0.434233775961515,1.71316198986504,
14.2426890400414));
#25883=CARTESIAN_POINT('Ctrl Pts',(-0.429325037372163,1.68839398250032,
14.2985571130423));
#25884=CARTESIAN_POINT('Ctrl Pts',(-0.419507560431212,1.6334513413436,14.4077416262965));
#25885=CARTESIAN_POINT('Ctrl Pts',(-0.40232697556216,1.52339204904435,14.5913779147532));
#25886=CARTESIAN_POINT('Ctrl Pts',(-0.387600760055443,1.40657398765396,
14.7337625495905));
#25887=CARTESIAN_POINT('Ctrl Pts',(-0.350785221174236,1.08273851420154,
15.0579597690902));
#25888=CARTESIAN_POINT('Ctrl Pts',(-0.296789097516509,0.476285039428357,
15.4012909875185));
#25889=CARTESIAN_POINT('Ctrl Pts',(-0.213340542615734,-0.600556246952718,
15.3749620338903));
#25890=CARTESIAN_POINT('Ctrl Pts',(-0.122528879886235,-1.58304430910793,
14.7197956084861));
#25891=CARTESIAN_POINT('Ctrl Pts',(-0.0587152790700956,-1.8675942981973,
13.927777469134));
#25892=CARTESIAN_POINT('Ctrl Pts',(0.0100070600863068,-1.86761983033918,
13.0723336751479));
#25893=CARTESIAN_POINT('Ctrl Pts',(0.0738206608959717,-1.58311665986085,
12.2802987218011));
#25894=CARTESIAN_POINT('Ctrl Pts',(0.164632323640247,-0.600668197270314,
11.6250749647134));
#25895=CARTESIAN_POINT('Ctrl Pts',(0.248080878521423,0.476171360890716,
11.5986828860266));
#25896=CARTESIAN_POINT('Ctrl Pts',(0.302077002185279,1.08264277791298,11.9419808031196));
#25897=CARTESIAN_POINT('Ctrl Pts',(0.338892541089085,1.40649893417158,12.266157604826));
#25898=CARTESIAN_POINT('Ctrl Pts',(0.351164387374828,1.50384840958494,12.3848125514054));
#25899=CARTESIAN_POINT('Ctrl Pts',(0.365890602801437,1.60195104912399,12.5396951787418));
#25900=CARTESIAN_POINT('Ctrl Pts',(0.375708079966948,1.66219089380516,12.6460487393483));
#25901=CARTESIAN_POINT('Ctrl Pts',(0.383071187745898,1.70142775366068,12.7289881483073));
#25902=CARTESIAN_POINT('Ctrl Pts',(0.392888664884959,1.74818788890808,12.8418781801734));
#25903=CARTESIAN_POINT('Ctrl Pts',(0.407614880391224,1.81002885866779,13.0146550273087));
#25904=CARTESIAN_POINT('Ctrl Pts',(0.432158573017531,1.86990438259484,13.3157009880243));
#25905=CARTESIAN_POINT('Ctrl Pts',(0.466519742664319,1.8699655452867,13.7454525475317));
#25906=CARTESIAN_POINT('Ctrl Pts',(0.491063435304432,1.79499221766936,14.0449929131399));
#25907=CARTESIAN_POINT('Ctrl Pts',(0.520515866293551,1.65472151719971,14.3836519320234));
#25908=CARTESIAN_POINT('Ctrl Pts',(0.552422666642926,1.44837375641488,14.7281855842315));
#25909=CARTESIAN_POINT('Ctrl Pts',(0.60151005186875,0.978990666418381,15.1327440801011));
#25910=CARTESIAN_POINT('Ctrl Pts',(0.665323652724684,0.226781365827923,
15.4240327960859));
#25911=CARTESIAN_POINT('Ctrl Pts',(0.71195666868146,-0.375774382679836,
15.3655342908919));
#25912=CARTESIAN_POINT('Ctrl Pts',(0.751226576855593,-0.827287339935277,
15.1781408845209));
#25913=CARTESIAN_POINT('Ctrl Pts',(0.770861530946073,-1.0438544481067,15.0623839856104));
#25914=CARTESIAN_POINT('Ctrl Pts',(0.790496485045808,-1.23367697134313,
14.9066159119171));
#25915=CARTESIAN_POINT('Ctrl Pts',(0.805222700653011,-1.36328099370934,
14.776996415965));
#25916=CARTESIAN_POINT('Ctrl Pts',(0.819948916128669,-1.48654046797679,
14.6410456587964));
#25917=CARTESIAN_POINT('Ctrl Pts',(0.844492608835747,-1.65701565369615,
14.3858165693403));
#25918=CARTESIAN_POINT('Ctrl Pts',(0.883762516987446,-1.84518520703327,
13.932103302506));
#25919=CARTESIAN_POINT('Ctrl Pts',(0.920578056028856,-1.89101584313679,
13.4673259234246));
#25920=CARTESIAN_POINT('Ctrl Pts',(0.950030486875574,-1.82801700727461,
13.1051559267996));
#25921=CARTESIAN_POINT('Ctrl Pts',(0.964756702494275,-1.77912068879012,
12.9284624028924));
#25922=CARTESIAN_POINT('Ctrl Pts',(0.972119810278298,-1.74822170447994,
12.8420572325272));
#25923=CARTESIAN_POINT('Ctrl Pts',(0.996663502882085,-1.63130050620839,
12.5599013225452));
#25924=CARTESIAN_POINT('Ctrl Pts',(1.01629845701254,-1.49295022231228,12.352705383945));
#25925=CARTESIAN_POINT('Ctrl Pts',(1.05065962660513,-1.19056003230052,12.050319698693));
#25926=CARTESIAN_POINT('Ctrl Pts',(1.08011205768541,-0.892959426854112,
11.8299056561741));
#25927=CARTESIAN_POINT('Ctrl Pts',(1.13901691999234,-0.195028119944808,
11.5789984993715));
#25928=CARTESIAN_POINT('Ctrl Pts',(1.18319556674322,0.375789682526766,11.634413850994));
#25929=CARTESIAN_POINT('Ctrl Pts',(1.22982858265304,0.911990235958854,11.856961997154));
#25930=CARTESIAN_POINT('Ctrl Pts',(1.26418975222758,1.27812764581854,12.0892036582747));
#25931=CARTESIAN_POINT('Ctrl Pts',(1.3280033530514,1.77582538844162,12.7243584776999));
#25932=CARTESIAN_POINT('Ctrl Pts',(1.39181695394423,1.93748780829106,13.5369124982985));
#25933=CARTESIAN_POINT('Ctrl Pts',(1.45563055475692,1.72077000069959,14.3141600253852));
#25934=CARTESIAN_POINT('Ctrl Pts',(1.48999172433415,1.47144910986013,14.6689268368013));
#25935=CARTESIAN_POINT('Ctrl Pts',(1.53171600179601,1.10422705446681,15.0361161891462));
#25936=CARTESIAN_POINT('Ctrl Pts',(1.57589464857577,0.618264596492589,15.3271025815264));
#25937=CARTESIAN_POINT('Ctrl Pts',(1.6397082494017,-0.187800383852184,15.4062806204875));
#25938=CARTESIAN_POINT('Ctrl Pts',(1.68879563447951,-0.78365481480013,15.2255036805631));
#25939=CARTESIAN_POINT('Ctrl Pts',(1.72315680406778,-1.14089950151332,14.9865612032227));
#25940=CARTESIAN_POINT('Ctrl Pts',(1.73788301959999,-1.27686789199295,14.8633440871825));
#25941=CARTESIAN_POINT('Ctrl Pts',(1.74524612746181,-1.34167720988981,14.7985504880953));
#25942=CARTESIAN_POINT('Ctrl Pts',(1.75506360447765,-1.4259529256506,14.7100283526174));
#25943=CARTESIAN_POINT('Ctrl Pts',(1.77960729714949,-1.6143304908496,14.4685858375326));
#25944=CARTESIAN_POINT('Ctrl Pts',(1.82624031312,-1.86605531676253,13.9382928885807));
#25945=CARTESIAN_POINT('Ctrl Pts',(1.8851451753049,-1.90309317982369,13.1839425839232));
#25946=CARTESIAN_POINT('Ctrl Pts',(1.94895877604335,-1.5925422036829,12.4358221265291));
#25947=CARTESIAN_POINT('Ctrl Pts',(2.01031800755653,-1.04241078847366,11.8851737608717));
#25948=CARTESIAN_POINT('Ctrl Pts',(2.07413160821739,-0.283042883570731,
11.5921167431507));
#25949=CARTESIAN_POINT('Ctrl Pts',(2.14039957820167,0.559797274712904,11.6543164405991));
#25950=CARTESIAN_POINT('Ctrl Pts',(2.20666754840405,1.29522400889582,12.0708980789732));
#25951=CARTESIAN_POINT('Ctrl Pts',(2.25084619508075,1.6195887412875,12.5315349098769));
#25952=CARTESIAN_POINT('Ctrl Pts',(2.27620801067512,1.74041786042992,12.8231426370461));
#25953=CARTESIAN_POINT('Ctrl Pts',(2.27988956458325,1.75656173412752,12.8660516752081));
#25954=CARTESIAN_POINT('Ctrl Pts',(2.28479830407995,1.77596808494156,12.9239826309265));
#25955=CARTESIAN_POINT('Ctrl Pts',(2.29134328165695,1.80057259257038,13.0016446570642));
#25956=CARTESIAN_POINT('Ctrl Pts',(2.30238796461873,1.8340181463693,13.1351463223963));
#25957=CARTESIAN_POINT('Ctrl Pts',(2.31711414297562,1.8609502466527,13.3166682127696));
#25958=CARTESIAN_POINT('Ctrl Pts',(2.32693164866254,1.86695551980756,13.4388529249682));
#25959=CARTESIAN_POINT('Ctrl Pts',(2.35147536869532,1.8669761579952,13.7443483740352));
#25960=CARTESIAN_POINT('Ctrl Pts',(2.37111020309486,1.81835939666339,13.9886114325472));
#25961=CARTESIAN_POINT('Ctrl Pts',(2.3931996159295,1.71319995454039,14.2426393076694));
#25962=CARTESIAN_POINT('Ctrl Pts',(2.41774343911922,1.58942689168338,14.5220193282036));
#25963=CARTESIAN_POINT('Ctrl Pts',(2.46192168824902,1.24283702002585,14.9660103282504));
#25964=CARTESIAN_POINT('Ctrl Pts',(2.52573584912865,0.528597455391128,15.3478865186278));
#25965=CARTESIAN_POINT('Ctrl Pts',(2.58954895542082,-0.282823439666157,
15.407853412087));
#25966=CARTESIAN_POINT('Ctrl Pts',(2.65827112993319,-1.10083352415133,15.0926576029327));
#25967=CARTESIAN_POINT('Ctrl Pts',(2.7245409139849,-1.67158419892642,14.4627976259999));
#25968=CARTESIAN_POINT('Ctrl Pts',(2.78835000017331,-1.90590776116979,13.6880601642426));
#25969=CARTESIAN_POINT('Ctrl Pts',(2.85708237956506,-1.821479964611,12.8195313357051));
#25970=CARTESIAN_POINT('Ctrl Pts',(2.91035772328115,-1.4376982387087,12.2440093096638));
#25971=CARTESIAN_POINT('Ctrl Pts',(2.94402092726701,-1.10215653765364,11.9922029531339));
#25972=CARTESIAN_POINT('Ctrl Pts',(2.94822541613613,-1.05904260584525,11.9625368481551));
#25973=CARTESIAN_POINT('Ctrl Pts',(-3.17266220035259,0.00264184562465942,
15.6006308241626));
#25974=CARTESIAN_POINT('Ctrl Pts',(-3.15544971768883,-0.239046808317434,
15.6009202622642));
#25975=CARTESIAN_POINT('Ctrl Pts',(-3.12102872579492,-0.720158267641467,
15.5176257131219));
#25976=CARTESIAN_POINT('Ctrl Pts',(-3.05708907174061,-1.51248273306104,
15.0705362781659));
#25977=CARTESIAN_POINT('Ctrl Pts',(-2.99086741120179,-2.04980411836316,
14.2660656413471));
#25978=CARTESIAN_POINT('Ctrl Pts',(-2.92212104198698,-2.1445664440175,13.288402600722));
#25979=CARTESIAN_POINT('Ctrl Pts',(-2.8583182735956,-1.88101160882473,12.4168213143143));
#25980=CARTESIAN_POINT('Ctrl Pts',(-2.7920459500128,-1.23875968366752,11.7079913692117));
#25981=CARTESIAN_POINT('Ctrl Pts',(-2.72332400615456,-0.318351097498607,
11.3533357827765));
#25982=CARTESIAN_POINT('Ctrl Pts',(-2.65951159229766,0.594666833883564,
11.420732594117));
#25983=CARTESIAN_POINT('Ctrl Pts',(-2.59569664716482,1.39833550923656,11.8504187872197));
#25984=CARTESIAN_POINT('Ctrl Pts',(-2.55151895485121,1.78838606602427,12.3499173356549));
#25985=CARTESIAN_POINT('Ctrl Pts',(-2.5269749488977,1.92762083664646,12.6643104262796));
#25986=CARTESIAN_POINT('Ctrl Pts',(-2.50488541080207,2.04601496321456,12.9501032916501));
#25987=CARTESIAN_POINT('Ctrl Pts',(-2.48525074400365,2.10067625814384,13.2249852988262));
#25988=CARTESIAN_POINT('Ctrl Pts',(-2.46070698565595,2.10067806416113,13.5687043580597));
#25989=CARTESIAN_POINT('Ctrl Pts',(-2.45088943986216,2.09392530800916,13.7061920430449));
#25990=CARTESIAN_POINT('Ctrl Pts',(-2.43616331352013,2.063631791612,13.9104351957971));
#25991=CARTESIAN_POINT('Ctrl Pts',(-2.42511860060563,2.02600652422355,14.0606546557986));
#25992=CARTESIAN_POINT('Ctrl Pts',(-2.41857363294159,1.99832432702032,14.1480389593073));
#25993=CARTESIAN_POINT('Ctrl Pts',(-2.41366489216172,1.97649509446574,14.2132245903546));
#25994=CARTESIAN_POINT('Ctrl Pts',(-2.40998333829098,1.95832480905997,14.2615042017653));
#25995=CARTESIAN_POINT('Ctrl Pts',(-2.38462152292895,1.82242492077781,14.5896371766628));
#25996=CARTESIAN_POINT('Ctrl Pts',(-2.34044287635804,1.4574325852988,15.1079453504089));
#25997=CARTESIAN_POINT('Ctrl Pts',(-2.2741749059696,0.629981383084626,15.5767198045092));
#25998=CARTESIAN_POINT('Ctrl Pts',(-2.20790693601996,-0.318384334109432,
15.646747379099));
#25999=CARTESIAN_POINT('Ctrl Pts',(-2.14409333543653,-1.17282687254162,
15.317041154053));
#26000=CARTESIAN_POINT('Ctrl Pts',(-2.08273410389093,-1.79186597979423,
14.6974827997507));
#26001=CARTESIAN_POINT('Ctrl Pts',(-2.01892050311859,-2.14131186029559,
13.8557240815807));
#26002=CARTESIAN_POINT('Ctrl Pts',(-1.96001564103395,-2.09969863559914,
13.0069296488875));
#26003=CARTESIAN_POINT('Ctrl Pts',(-1.91338262499469,-1.81645082636161,
12.4102412367691));
#26004=CARTESIAN_POINT('Ctrl Pts',(-1.88883893231528,-1.6045509056256,12.1385586862707));
#26005=CARTESIAN_POINT('Ctrl Pts',(-1.87902145533625,-1.50970215352713,
12.0389534490745));
#26006=CARTESIAN_POINT('Ctrl Pts',(-1.87165834748703,-1.43679234243196,
11.9660376433793));
#26007=CARTESIAN_POINT('Ctrl Pts',(-1.85693213191582,-1.28380123614643,
11.8274039902691));
#26008=CARTESIAN_POINT('Ctrl Pts',(-1.82257096232786,-0.881849651288155,
11.558510752652));
#26009=CARTESIAN_POINT('Ctrl Pts',(-1.77348357727153,-0.21141052754035,
11.3550706699088));
#26010=CARTESIAN_POINT('Ctrl Pts',(-1.70966997646036,0.695576906938657,
11.4441452651285));
#26011=CARTESIAN_POINT('Ctrl Pts',(-1.66549132964107,1.24238709858536,11.771472748311));
#26012=CARTESIAN_POINT('Ctrl Pts',(-1.62376705217685,1.655612733367,12.1846907466758));
#26013=CARTESIAN_POINT('Ctrl Pts',(-1.58940588261669,1.93613052167727,12.5838088251675));
#26014=CARTESIAN_POINT('Ctrl Pts',(-1.52559228183367,2.18004640024346,13.4583839812046));
#26015=CARTESIAN_POINT('Ctrl Pts',(-1.46177868085939,1.99819061811832,14.3726391361564));
#26016=CARTESIAN_POINT('Ctrl Pts',(-1.39796508005353,1.43818525007012,15.0873649788857));
#26017=CARTESIAN_POINT('Ctrl Pts',(-1.36360391049841,1.02626889486372,15.3486477476018));
#26018=CARTESIAN_POINT('Ctrl Pts',(-1.31697089460524,0.422912135353946,
15.599164614062));
#26019=CARTESIAN_POINT('Ctrl Pts',(-1.27279224785391,-0.219332827926,15.6615028656883));
#26020=CARTESIAN_POINT('Ctrl Pts',(-1.2138873854739,-1.00467417934464,15.3792058981596));
#26021=CARTESIAN_POINT('Ctrl Pts',(-1.18443495446031,-1.33952818945933,
15.1312597853418));
#26022=CARTESIAN_POINT('Ctrl Pts',(-1.15007378486252,-1.67979938218662,
14.7909543366238));
#26023=CARTESIAN_POINT('Ctrl Pts',(-1.13043883066505,-1.83550446245088,
14.5579405445852));
#26024=CARTESIAN_POINT('Ctrl Pts',(-1.10589513815342,-1.96703997856123,
14.240389049116));
#26025=CARTESIAN_POINT('Ctrl Pts',(-1.09853203041032,-2.00182960412185,
14.1431839218754));
#26026=CARTESIAN_POINT('Ctrl Pts',(-1.08380581461998,-2.05683123962386,
13.9443682479003));
#26027=CARTESIAN_POINT('Ctrl Pts',(-1.05435338403389,-2.12777334415797,
13.536861775514));
#26028=CARTESIAN_POINT('Ctrl Pts',(-1.0175378447822,-2.0762083485259,13.0139000451585));
#26029=CARTESIAN_POINT('Ctrl Pts',(-0.978267936728251,-1.864499032025,12.5033759025148));
#26030=CARTESIAN_POINT('Ctrl Pts',(-0.953724243927657,-1.67270341789268,
12.2161912935285));
#26031=CARTESIAN_POINT('Ctrl Pts',(-0.93899802849587,-1.5340127312506,12.0632069998174));
#26032=CARTESIAN_POINT('Ctrl Pts',(-0.924271812912939,-1.38819254281156,
11.9173769826473));
#26033=CARTESIAN_POINT('Ctrl Pts',(-0.904636858791085,-1.17461691688123,
11.7420376710293));
#26034=CARTESIAN_POINT('Ctrl Pts',(-0.885001904695471,-0.930935491319084,
11.6118636578801));
#26035=CARTESIAN_POINT('Ctrl Pts',(-0.84573199651817,-0.422923427845423,
11.4008528077841));
#26036=CARTESIAN_POINT('Ctrl Pts',(-0.799098980586865,0.255078212786275,
11.3351181015767));
#26037=CARTESIAN_POINT('Ctrl Pts',(-0.735285379702259,1.10146391779465,
11.6627814277576));
#26038=CARTESIAN_POINT('Ctrl Pts',(-0.686197994457681,1.6296328843616,12.1179713327371));
#26039=CARTESIAN_POINT('Ctrl Pts',(-0.654291194127137,1.86182645070982,
12.5056389077366));
#26040=CARTESIAN_POINT('Ctrl Pts',(-0.624838763160051,2.01967849078206,
12.8866708235145));
#26041=CARTESIAN_POINT('Ctrl Pts',(-0.60029507054379,2.10406567799361,13.2237189739029));
#26042=CARTESIAN_POINT('Ctrl Pts',(-0.57084263933558,2.10399684935638,13.6381840752747));
#26043=CARTESIAN_POINT('Ctrl Pts',(-0.546298946728076,2.05351727011022,
13.9785897887072));
#26044=CARTESIAN_POINT('Ctrl Pts',(-0.531572731173083,1.99338238766352,
14.1769042061779));
#26045=CARTESIAN_POINT('Ctrl Pts',(-0.519300884788924,1.92761739567746,
14.3356823998713));
#26046=CARTESIAN_POINT('Ctrl Pts',(-0.514392146187137,1.89975372144083,
14.3985487843327));
#26047=CARTESIAN_POINT('Ctrl Pts',(-0.504574669387815,1.83791895148544,
14.5213910515937));
#26048=CARTESIAN_POINT('Ctrl Pts',(-0.487394084415219,1.71410350172111,
14.7280360584275));
#26049=CARTESIAN_POINT('Ctrl Pts',(-0.472667868905623,1.58262085472758,
14.888210024574));
#26050=CARTESIAN_POINT('Ctrl Pts',(-0.435852330022712,1.21829850806929,
15.2530421057079));
#26051=CARTESIAN_POINT('Ctrl Pts',(-0.381856206388399,0.535859744814445,
15.6392692230569));
#26052=CARTESIAN_POINT('Ctrl Pts',(-0.298407651514801,-0.67574596699535,
15.6097342394618));
#26053=CARTESIAN_POINT('Ctrl Pts',(-0.20759598870574,-1.78125190703748,
14.8724643137972));
#26054=CARTESIAN_POINT('Ctrl Pts',(-0.143782387914756,-2.10141357731427,
13.9813209628623));
#26055=CARTESIAN_POINT('Ctrl Pts',(-0.0750600487909853,-2.10142877451732,
13.018745682568));
#26056=CARTESIAN_POINT('Ctrl Pts',(-0.0112464480162327,-1.78129552929104,
12.127592539261));
#26057=CARTESIAN_POINT('Ctrl Pts',(0.079565214828448,-0.67581288028697,
11.3902881479926));
#26058=CARTESIAN_POINT('Ctrl Pts',(0.163013769655459,0.53579047445301,11.3607166917808));
#26059=CARTESIAN_POINT('Ctrl Pts',(0.217009893304003,1.21824103378077,11.7469232259717));
#26060=CARTESIAN_POINT('Ctrl Pts',(0.253825432241908,1.58257316404802,12.1117453517784));
#26061=CARTESIAN_POINT('Ctrl Pts',(0.266097278544301,1.69215006954595,12.2452185124881));
#26062=CARTESIAN_POINT('Ctrl Pts',(0.280823493861359,1.80250551956799,12.4195149158672));
#26063=CARTESIAN_POINT('Ctrl Pts',(0.290640971199572,1.87029759818536,12.5391729746263));
#26064=CARTESIAN_POINT('Ctrl Pts',(0.298004078932886,1.91443752392828,12.6325030347934));
#26065=CARTESIAN_POINT('Ctrl Pts',(0.307821556042263,1.96705153765617,12.7595242806143));
#26066=CARTESIAN_POINT('Ctrl Pts',(0.322547771550418,2.03663286377444,12.9539313301886));
#26067=CARTESIAN_POINT('Ctrl Pts',(0.347091464122481,2.10399912325221,13.2926681274472));
#26068=CARTESIAN_POINT('Ctrl Pts',(0.381452633849436,2.10406095745389,13.7762140318887));
#26069=CARTESIAN_POINT('Ctrl Pts',(0.405996326453825,2.01970108901493,14.1132638203997));
#26070=CARTESIAN_POINT('Ctrl Pts',(0.435448757415273,1.86185886016731,14.4943011233421));
#26071=CARTESIAN_POINT('Ctrl Pts',(0.467355557750643,1.62967766233521,14.8819763128389));
#26072=CARTESIAN_POINT('Ctrl Pts',(0.516442942996658,1.10152229544305,15.3371831862365));
#26073=CARTESIAN_POINT('Ctrl Pts',(0.580256543880559,0.255146656090134,
15.6648734409929));
#26074=CARTESIAN_POINT('Ctrl Pts',(0.626889559804317,-0.422857263281462,
15.5991601609565));
#26075=CARTESIAN_POINT('Ctrl Pts',(0.66615946798391,-0.930876015826006,
15.3881653339733));
#26076=CARTESIAN_POINT('Ctrl Pts',(0.685794422082415,-1.17456155931576,
15.2579989996418));
#26077=CARTESIAN_POINT('Ctrl Pts',(0.705429376203152,-1.38814271520269,
15.0826664192684));
#26078=CARTESIAN_POINT('Ctrl Pts',(0.720155591788415,-1.5339674905036,14.9368409887842));
#26079=CARTESIAN_POINT('Ctrl Pts',(0.734881807223654,-1.67266298412755,
14.7838610537252));
#26080=CARTESIAN_POINT('Ctrl Pts',(0.759425499988951,-1.86446763640772,
14.4966824904347));
#26081=CARTESIAN_POINT('Ctrl Pts',(0.798695408116211,-2.07619298774507,
13.9861650044251));
#26082=CARTESIAN_POINT('Ctrl Pts',(0.83551094730015,-2.1277744490612,13.4632049483027));
#26083=CARTESIAN_POINT('Ctrl Pts',(0.864963377919054,-2.05684513787007,
13.0556962539315));
#26084=CARTESIAN_POINT('Ctrl Pts',(0.879689593697196,-2.00184974289138,
12.856878855445));
#26085=CARTESIAN_POINT('Ctrl Pts',(0.88705270144308,-1.96706316877626,12.7596726372977));
#26086=CARTESIAN_POINT('Ctrl Pts',(0.911596393960796,-1.83553762188005,
12.4421170175806));
#26087=CARTESIAN_POINT('Ctrl Pts',(0.931231348155162,-1.67983986643869,
12.2090983517141));
#26088=CARTESIAN_POINT('Ctrl Pts',(0.96559251775177,-1.33957935861203,11.8687822298386));
#26089=CARTESIAN_POINT('Ctrl Pts',(0.99504494876616,-1.00473313541158,11.620825614142));
#26090=CARTESIAN_POINT('Ctrl Pts',(1.05394981114623,-0.219400648575714,
11.3385040063844));
#26091=CARTESIAN_POINT('Ctrl Pts',(1.09812845789801,0.422846266856786,11.4008221062241));
#26092=CARTESIAN_POINT('Ctrl Pts',(1.14476147379055,1.02621088612219,11.6513200396668));
#26093=CARTESIAN_POINT('Ctrl Pts',(1.17912264334457,1.43813543913076,11.9125898832225));
#26094=CARTESIAN_POINT('Ctrl Pts',(1.24293624415171,1.99816323522134,12.6272981531672));
#26095=CARTESIAN_POINT('Ctrl Pts',(1.30674984512595,2.18004770840565,13.5415476016066));
#26096=CARTESIAN_POINT('Ctrl Pts',(1.37056344590792,1.93615927629818,14.4161304124479));
#26097=CARTESIAN_POINT('Ctrl Pts',(1.40492461546698,1.6556540141085,14.8152572944509));
#26098=CARTESIAN_POINT('Ctrl Pts',(1.44664889293198,1.24244134800518,15.2284882608853));
#26099=CARTESIAN_POINT('Ctrl Pts',(1.49082753975291,0.695641431593744,15.5558329045212));
#26100=CARTESIAN_POINT('Ctrl Pts',(1.55464114056533,-0.211343205044639,
15.6449359634957));
#26101=CARTESIAN_POINT('Ctrl Pts',(1.60372852562089,-0.881788707995604,
15.4415169212182));
#26102=CARTESIAN_POINT('Ctrl Pts',(1.63808969520711,-1.28374872909566,15.1726362981186));
#26103=CARTESIAN_POINT('Ctrl Pts',(1.65281591077819,-1.43674418522118,15.0340074462966));
#26104=CARTESIAN_POINT('Ctrl Pts',(1.66017901862767,-1.5096562843569,14.9610939287589));
#26105=CARTESIAN_POINT('Ctrl Pts',(1.66999649560661,-1.60450816196902,14.8614916681869));
#26106=CARTESIAN_POINT('Ctrl Pts',(1.6945401882874,-1.81641660638884,14.5898157678553));
#26107=CARTESIAN_POINT('Ctrl Pts',(1.74117320432588,-2.09968312529506,13.993136245687));
#26108=CARTESIAN_POINT('Ctrl Pts',(1.80007806641223,-2.14132297639453,13.1443431199714));
#26109=CARTESIAN_POINT('Ctrl Pts',(1.86389166718199,-1.79190346307116,12.3025734370431));
#26110=CARTESIAN_POINT('Ctrl Pts',(1.92525089873163,-1.1728837333095,11.6829956582692));
#26111=CARTESIAN_POINT('Ctrl Pts',(1.9890644993147,-0.318451445307582,11.353262621575));
#26112=CARTESIAN_POINT('Ctrl Pts',(2.05533246926636,0.629916684121097,11.4232604409134));
#26113=CARTESIAN_POINT('Ctrl Pts',(2.12160043965998,1.45738279440301,11.8920089333997));
#26114=CARTESIAN_POINT('Ctrl Pts',(2.16577908623353,1.82239184147097,12.4103056664616));
#26115=CARTESIAN_POINT('Ctrl Pts',(2.19114090159337,1.95830212268135,12.7384343791443));
#26116=CARTESIAN_POINT('Ctrl Pts',(2.19482245546371,1.97647393187141,12.7867134206883));
#26117=CARTESIAN_POINT('Ctrl Pts',(2.19973119624365,1.99830521034253,12.8518983669964));
#26118=CARTESIAN_POINT('Ctrl Pts',(2.20627616390887,2.02599016863268,12.9392817993886));
#26119=CARTESIAN_POINT('Ctrl Pts',(2.21732087682484,2.06362019625161,13.0895000864374));
#26120=CARTESIAN_POINT('Ctrl Pts',(2.23204700316566,2.09392025952937,13.2937422834945));
#26121=CARTESIAN_POINT('Ctrl Pts',(2.24186454896205,2.10067736162775,13.4312297636866));
#26122=CARTESIAN_POINT('Ctrl Pts',(2.26640830731602,2.1006866380108,13.7749488306902));
#26123=CARTESIAN_POINT('Ctrl Pts',(2.286042974127,2.04603571825695,14.0498326403604));
#26124=CARTESIAN_POINT('Ctrl Pts',(2.30813251222673,1.9276507441991,14.3356292078984));
#26125=CARTESIAN_POINT('Ctrl Pts',(2.33267651818434,1.78842576055076,14.6500263621867));
#26126=CARTESIAN_POINT('Ctrl Pts',(2.37685421054368,1.39839795140035,15.1495402659449));
#26127=CARTESIAN_POINT('Ctrl Pts',(2.44066915571005,0.594740868894852,15.5792454847316));
#26128=CARTESIAN_POINT('Ctrl Pts',(2.50448156968343,-0.318252030767666,
15.6466850868822));
#26129=CARTESIAN_POINT('Ctrl Pts',(2.5732035136348,-1.23868770045141,15.2920299004919));
#26130=CARTESIAN_POINT('Ctrl Pts',(2.63947583757363,-1.88086695443964,14.5832859786279));
#26131=CARTESIAN_POINT('Ctrl Pts',(2.70327860614168,-2.14454478615246,13.7115935900664));
#26132=CARTESIAN_POINT('Ctrl Pts',(2.77202497624202,-2.04943982851017,12.7342369759876));
#26133=CARTESIAN_POINT('Ctrl Pts',(2.82527858318522,-1.61782105646327,12.0867954330277));
#26134=CARTESIAN_POINT('Ctrl Pts',(2.8589519925713,-1.24010853015882,11.8034581198931));
#26135=CARTESIAN_POINT('Ctrl Pts',(2.8631579592014,-1.19160472684239,11.7700461798512));
#26136=CARTESIAN_POINT('',(-2.91382504120091,0.,14.89));
#26137=CARTESIAN_POINT('Origin',(-3.29867228626928,0.,15.245));
#26138=CARTESIAN_POINT('Ctrl Pts',(-2.86395232247026,1.18339323898477,11.7647413855289));
#26139=CARTESIAN_POINT('Ctrl Pts',(-2.85951639598233,1.23470680988399,11.799740100392));
#26140=CARTESIAN_POINT('Ctrl Pts',(-2.83299103552865,1.5324114987355,12.0225088821029));
#26141=CARTESIAN_POINT('Ctrl Pts',(-2.8040120778353,1.78814814342653,12.3501521071371));
#26142=CARTESIAN_POINT('Ctrl Pts',(-2.77946807208677,1.92737178398469,12.6645011910224));
#26143=CARTESIAN_POINT('Ctrl Pts',(-2.75737853413057,2.04574294616347,12.9502605082012));
#26144=CARTESIAN_POINT('Ctrl Pts',(-2.73774386712553,2.10040352107426,13.2250982876992));
#26145=CARTESIAN_POINT('Ctrl Pts',(-2.71320010881799,2.10039759285345,13.5687716283892));
#26146=CARTESIAN_POINT('Ctrl Pts',(-2.703382563069,2.0936420873127,13.7062412062418));
#26147=CARTESIAN_POINT('Ctrl Pts',(-2.68865643666704,2.06334666234638,13.9104570270601));
#26148=CARTESIAN_POINT('Ctrl Pts',(-2.67761172378578,2.02572215584014,14.0606557808409));
#26149=CARTESIAN_POINT('Ctrl Pts',(-2.67106675611039,1.99804077971579,14.1480281091204));
#26150=CARTESIAN_POINT('Ctrl Pts',(-2.66615801533196,1.97621227192314,14.2132048011292));
#26151=CARTESIAN_POINT('Ctrl Pts',(-2.66247646146109,1.95804284955894,14.2614776811265));
#26152=CARTESIAN_POINT('Ctrl Pts',(-2.63711464609784,1.82215054249416,14.5895642078971));
#26153=CARTESIAN_POINT('Ctrl Pts',(-2.59293599952233,1.45719179411054,15.107792259493));
#26154=CARTESIAN_POINT('Ctrl Pts',(-2.52666802913216,0.629832203340271,
15.5764801682427));
#26155=CARTESIAN_POINT('Ctrl Pts',(-2.46040005918036,-0.318413945911626,
15.6464676527716));
#26156=CARTESIAN_POINT('Ctrl Pts',(-2.39658645859582,-1.17273725777722,
15.3167756828035));
#26157=CARTESIAN_POINT('Ctrl Pts',(-2.33522722704962,-1.79167816896257,
14.6972758001249));
#26158=CARTESIAN_POINT('Ctrl Pts',(-2.27141362627676,-2.14105325390368,
13.855612208645));
#26159=CARTESIAN_POINT('Ctrl Pts',(-2.21250876419197,-2.09941852228509,
13.0069263498048));
#26160=CARTESIAN_POINT('Ctrl Pts',(-2.16587574815266,-1.81618760322336,
12.4103221850427));
#26161=CARTESIAN_POINT('Ctrl Pts',(-2.14133205547323,-1.60430579232672,
12.13868064052));
#26162=CARTESIAN_POINT('Ctrl Pts',(-2.13151457849414,-1.50946592983573,
12.0390909700533));
#26163=CARTESIAN_POINT('Ctrl Pts',(-2.12415147064491,-1.43656303221216,
11.9661866807793));
#26164=CARTESIAN_POINT('Ctrl Pts',(-2.10942525507374,-1.28358690527117,
11.8275753375537));
#26165=CARTESIAN_POINT('Ctrl Pts',(-2.07506408548576,-0.881677639438382,
11.5587288109207));
#26166=CARTESIAN_POINT('Ctrl Pts',(-2.02597670042933,-0.211316719569808,
11.3553356115629));
#26167=CARTESIAN_POINT('Ctrl Pts',(-1.96216309961809,0.695553256549286,
11.4444274965203));
#26168=CARTESIAN_POINT('Ctrl Pts',(-1.91798445279889,1.24228418885524,11.7717307237019));
#26169=CARTESIAN_POINT('Ctrl Pts',(-1.87626017533466,1.65544468008186,12.1849091373921));
#26170=CARTESIAN_POINT('Ctrl Pts',(-1.84189900577446,1.93591474668381,12.5839855411706));
#26171=CARTESIAN_POINT('Ctrl Pts',(-1.77808540499141,2.17977217767513,13.4584576635979));
#26172=CARTESIAN_POINT('Ctrl Pts',(-1.71427180401722,1.99791066935068,14.3725915504926));
#26173=CARTESIAN_POINT('Ctrl Pts',(-1.65045820321132,1.43795381725481,15.0872093791297));
#26174=CARTESIAN_POINT('Ctrl Pts',(-1.61609703365616,1.02608112988485,15.3484460912615));
#26175=CARTESIAN_POINT('Ctrl Pts',(-1.56946401776296,0.422792880231089,
15.5989118787714));
#26176=CARTESIAN_POINT('Ctrl Pts',(-1.52528537101175,-0.219372883281587,
15.6612220798083));
#26177=CARTESIAN_POINT('Ctrl Pts',(-1.46638050863173,-1.00460604457137,
15.3789362729773));
#26178=CARTESIAN_POINT('Ctrl Pts',(-1.43692807761804,-1.33940996924325,
15.1310108721175));
#26179=CARTESIAN_POINT('Ctrl Pts',(-1.40256690802025,-1.67962743720217,
14.790737877859));
#26180=CARTESIAN_POINT('Ctrl Pts',(-1.38293195382286,-1.83530555995113,
14.5577485921235));
#26181=CARTESIAN_POINT('Ctrl Pts',(-1.35838826131112,-1.96681455751747,
14.2402332233263));
#26182=CARTESIAN_POINT('Ctrl Pts',(-1.35102515356799,-2.00159671759724,
14.1430392814066));
#26183=CARTESIAN_POINT('Ctrl Pts',(-1.33629893777783,-2.05658519035004,
13.9442470225823));
#26184=CARTESIAN_POINT('Ctrl Pts',(-1.30684650719147,-2.12750545897677,
13.5367898517779));
#26185=CARTESIAN_POINT('Ctrl Pts',(-1.27003096793995,-2.07593057890912,
13.0138958671947));
#26186=CARTESIAN_POINT('Ctrl Pts',(-1.23076105988595,-1.86423205700168,
12.5034429312468));
#26187=CARTESIAN_POINT('Ctrl Pts',(-1.20621736708542,-1.67245166038405,
12.2163007047761));
#26188=CARTESIAN_POINT('Ctrl Pts',(-1.1914911516536,-1.53377371678283,12.0633401357287));
#26189=CARTESIAN_POINT('Ctrl Pts',(-1.17676493607063,-1.38796737947216,
11.9175331486101));
#26190=CARTESIAN_POINT('Ctrl Pts',(-1.15712998194875,-1.17441323673287,
11.7422228942938));
#26191=CARTESIAN_POINT('Ctrl Pts',(-1.1374950278532,-0.930758522391391,
11.6120730373285));
#26192=CARTESIAN_POINT('Ctrl Pts',(-1.09822511967589,-0.422803967350463,
11.4011055450012));
#26193=CARTESIAN_POINT('Ctrl Pts',(-1.05159210374468,0.255114060124627,
11.3354006658051));
#26194=CARTESIAN_POINT('Ctrl Pts',(-0.987778502859985,1.10138252402949,
11.6630493850669));
#26195=CARTESIAN_POINT('Ctrl Pts',(-0.938691117615512,1.62947047446097,
12.1181985558448));
#26196=CARTESIAN_POINT('Ctrl Pts',(-0.906784317284843,1.86162252844231,
12.505824402897));
#26197=CARTESIAN_POINT('Ctrl Pts',(-0.877331886317726,2.01944264609616,
12.8868131774084));
#26198=CARTESIAN_POINT('Ctrl Pts',(-0.852788193701485,2.10380859651136,
13.2238214133424));
#26199=CARTESIAN_POINT('Ctrl Pts',(-0.823335762493315,2.10372675620362,
13.6382341331381));
#26200=CARTESIAN_POINT('Ctrl Pts',(-0.798792069885758,2.05324287076447,
13.9785952306268));
#26201=CARTESIAN_POINT('Ctrl Pts',(-0.784065854330827,1.99310933344462,
14.1768826785089));
#26202=CARTESIAN_POINT('Ctrl Pts',(-0.7717940079467,1.92734766933172,14.335638732088));
#26203=CARTESIAN_POINT('Ctrl Pts',(-0.766885269344943,1.89948553670055,
14.3984962882538));
#26204=CARTESIAN_POINT('Ctrl Pts',(-0.757067792545443,1.8376547328267,14.5213210863396));
#26205=CARTESIAN_POINT('Ctrl Pts',(-0.739887207572969,1.71384840296856,
14.7279360406703));
#26206=CARTESIAN_POINT('Ctrl Pts',(-0.725160992063393,1.5823773053324,14.8880855588829));
#26207=CARTESIAN_POINT('Ctrl Pts',(-0.688345453180475,1.21808924244413,
15.2528597399623));
#26208=CARTESIAN_POINT('Ctrl Pts',(-0.63434932954611,0.535724535273187,
15.6390163094263));
#26209=CARTESIAN_POINT('Ctrl Pts',(-0.550900774672618,-0.6757274452496,
15.609444965228));
#26210=CARTESIAN_POINT('Ctrl Pts',(-0.460089111863575,-1.78107000044726,
14.8722340315906));
#26211=CARTESIAN_POINT('Ctrl Pts',(-0.396275511072554,-2.10116286876526,
13.9811937613502));
#26212=CARTESIAN_POINT('Ctrl Pts',(-0.327553171948746,-2.10114784905051,
13.018740961484));
#26213=CARTESIAN_POINT('Ctrl Pts',(-0.263739571173964,-1.78102745715508,
12.1277110014121));
#26214=CARTESIAN_POINT('Ctrl Pts',(-0.172927908329469,-0.675661904576781,
11.3905350167616));
#26215=CARTESIAN_POINT('Ctrl Pts',(-0.0894793535022535,0.535789576569599,
11.3610032710076));
#26216=CARTESIAN_POINT('Ctrl Pts',(-0.0354832298537147,1.21814183783093,
11.747182094498));
#26217=CARTESIAN_POINT('Ctrl Pts',(0.00133230908414512,1.58241678739983,
12.1119691836169));
#26218=CARTESIAN_POINT('Ctrl Pts',(0.0136041553865288,1.69197569693335,
12.2454288356657));
#26219=CARTESIAN_POINT('Ctrl Pts',(0.0283303707037281,1.80231176016096,
12.4197066355812));
#26220=CARTESIAN_POINT('Ctrl Pts',(0.0381478480417329,1.87009150500503,
12.5393516987898));
#26221=CARTESIAN_POINT('Ctrl Pts',(0.0455109557751048,1.91422294038976,
12.6326713282807));
#26222=CARTESIAN_POINT('Ctrl Pts',(0.0553284328845138,1.96682631953794,
12.7596781644253));
#26223=CARTESIAN_POINT('Ctrl Pts',(0.0700546483926733,2.03639275364112,
12.9540628133223));
#26224=CARTESIAN_POINT('Ctrl Pts',(0.0945983409647811,2.10373988430058,
13.2927589040249));
#26225=CARTESIAN_POINT('Ctrl Pts',(0.128959510691625,2.1037865350476,13.7762436940241));
#26226=CARTESIAN_POINT('Ctrl Pts',(0.153503203296114,2.01942674468552,14.1132482690728));
#26227=CARTESIAN_POINT('Ctrl Pts',(0.182955634257591,1.86159251610715,14.4942325177201));
#26228=CARTESIAN_POINT('Ctrl Pts',(0.214862434592872,1.62942849097079,14.8818513989961));
#26229=CARTESIAN_POINT('Ctrl Pts',(0.263949819838949,1.10132555773969,15.3369843770367));
#26230=CARTESIAN_POINT('Ctrl Pts',(0.327763420722699,0.255046583726186,
15.6646068840464));
#26231=CARTESIAN_POINT('Ctrl Pts',(0.374396436646611,-0.422869598616443,
15.5988808622999));
#26232=CARTESIAN_POINT('Ctrl Pts',(0.413666344826193,-0.93081759534357,
15.3878974965819));
#26233=CARTESIAN_POINT('Ctrl Pts',(0.433301298924743,-1.17446825510573,
15.2577400181351));
#26234=CARTESIAN_POINT('Ctrl Pts',(0.452936253045398,-1.38801691891332,
15.0824230855869));
#26235=CARTESIAN_POINT('Ctrl Pts',(0.467662468630681,-1.53381868681228,
14.9366115293155));
#26236=CARTESIAN_POINT('Ctrl Pts',(0.482388684065977,-1.67249183188709,
14.7836466105238));
#26237=CARTESIAN_POINT('Ctrl Pts',(0.506932376831184,-1.86426323547285,
14.4964983877605));
#26238=CARTESIAN_POINT('Ctrl Pts',(0.546202284958494,-2.07594573733582,
13.9860388151222));
#26239=CARTESIAN_POINT('Ctrl Pts',(0.58301782414224,-2.12750424881575,13.463143268723));
#26240=CARTESIAN_POINT('Ctrl Pts',(0.61247025476142,-2.05657118613531,13.0556883300511));
#26241=CARTESIAN_POINT('Ctrl Pts',(0.62719647053937,-2.00157647080744,12.8568978000849));
#26242=CARTESIAN_POINT('Ctrl Pts',(0.634559578285301,-1.96679125863703,
12.7597049515784));
#26243=CARTESIAN_POINT('Ctrl Pts',(0.659103270803122,-1.83527229136505,
12.4421937174885));
#26244=CARTESIAN_POINT('Ctrl Pts',(0.67873822499742,-1.67958686286578,12.2092093349896));
#26245=CARTESIAN_POINT('Ctrl Pts',(0.713099394594027,-1.33935871215268,
11.8689470329008));
#26246=CARTESIAN_POINT('Ctrl Pts',(0.742551825608453,-1.0045470059286,11.6210321549827));
#26247=CARTESIAN_POINT('Ctrl Pts',(0.801456687988358,-0.219304983886525,
11.33877101901));
#26248=CARTESIAN_POINT('Ctrl Pts',(0.845635334740273,0.422858819730382,
11.4011013952));
#26249=CARTESIAN_POINT('Ctrl Pts',(0.892268350632809,1.02613920072941,11.6515861350263));
#26250=CARTESIAN_POINT('Ctrl Pts',(0.926629520186844,1.43800368130773,11.9128357874006));
#26251=CARTESIAN_POINT('Ctrl Pts',(0.99044312099397,1.99793808743644,12.6274712081551));
#26252=CARTESIAN_POINT('Ctrl Pts',(1.05425672196811,2.17977088478312,13.5416108112303));
#26253=CARTESIAN_POINT('Ctrl Pts',(1.11807032275011,1.93588599253454,14.4160752800524));
#26254=CARTESIAN_POINT('Ctrl Pts',(1.15243149230917,1.65540339740651,14.8151428801159));
#26255=CARTESIAN_POINT('Ctrl Pts',(1.19415576977416,1.2422299359489,15.2283083230172));
#26256=CARTESIAN_POINT('Ctrl Pts',(1.23833441659508,0.695488745466205,15.5555943973105));
#26257=CARTESIAN_POINT('Ctrl Pts',(1.30214801740745,-0.211384009584384,
15.6446578133189));
#26258=CARTESIAN_POINT('Ctrl Pts',(1.35123540246295,-0.881738497810867,
15.4412435944634));
#26259=CARTESIAN_POINT('Ctrl Pts',(1.38559657204916,-1.28363930202604,15.172384458236));
#26260=CARTESIAN_POINT('Ctrl Pts',(1.40032278762018,-1.43661106863639,15.0337683155675));
#26261=CARTESIAN_POINT('Ctrl Pts',(1.40768589546967,-1.50951167457381,14.9608617378445));
#26262=CARTESIAN_POINT('Ctrl Pts',(1.41750337244863,-1.60434840567024,14.8612690911551));
#26263=CARTESIAN_POINT('Ctrl Pts',(1.44204706512938,-1.81622166540711,14.5896209074415));
#26264=CARTESIAN_POINT('Ctrl Pts',(1.48868008116764,-2.09943371647049,13.9930079562618));
#26265=CARTESIAN_POINT('Ctrl Pts',(1.54758494325403,-2.14104170095398,13.144320866245));
#26266=CARTESIAN_POINT('Ctrl Pts',(1.61139854402315,-1.79163977666453,12.3026685936186));
#26267=CARTESIAN_POINT('Ctrl Pts',(1.672757775572,-1.17267887511365,11.6831886072225));
#26268=CARTESIAN_POINT('Ctrl Pts',(1.73657137615399,-0.318344426567643,
11.3535241406746));
#26269=CARTESIAN_POINT('Ctrl Pts',(1.80283934610328,0.629901232782519,11.4235428712566));
#26270=CARTESIAN_POINT('Ctrl Pts',(1.86910731649445,1.45724767055709,11.8922581094627));
#26271=CARTESIAN_POINT('Ctrl Pts',(1.9132859630631,1.82219364420109,12.4105006201815));
#26272=CARTESIAN_POINT('Ctrl Pts',(1.93864777842214,1.958076391633,12.7385920533271));
#26273=CARTESIAN_POINT('Ctrl Pts',(1.94232933229241,1.97624436428055,12.786865560793));
#26274=CARTESIAN_POINT('Ctrl Pts',(1.9472380730709,1.9980708388772,12.8520429490877));
#26275=CARTESIAN_POINT('Ctrl Pts',(1.95378304074728,2.02574952526818,12.9394162047849));
#26276=CARTESIAN_POINT('Ctrl Pts',(1.96482775362835,2.06336995074317,13.0896166528483));
#26277=CARTESIAN_POINT('Ctrl Pts',(1.97955388002742,2.09365953804166,13.2938339723862));
#26278=CARTESIAN_POINT('Ctrl Pts',(1.9893714257774,2.10041134743223,13.4313042539146));
#26279=CARTESIAN_POINT('Ctrl Pts',(2.01391518408421,2.10040911756558,13.7749798122416));
#26280=CARTESIAN_POINT('Ctrl Pts',(2.03354985106829,2.04575275009202,14.0498267163717));
#26281=CARTESIAN_POINT('Ctrl Pts',(2.05563938902259,1.92737336277738,14.3355834398345));
#26282=CARTESIAN_POINT('Ctrl Pts',(2.08018339476934,1.78815549053371,14.6499365896423));
#26283=CARTESIAN_POINT('Ctrl Pts',(2.12436108771495,1.39815247612617,15.1493719808017));
#26284=CARTESIAN_POINT('Ctrl Pts',(2.1881760319483,0.594574019921796,15.5790015900282));
#26285=CARTESIAN_POINT('Ctrl Pts',(2.25198844660101,-0.318322870616011,
15.6463919965956));
#26286=CARTESIAN_POINT('Ctrl Pts',(2.32071039067994,-1.23866577243641,15.2917708772129));
#26287=CARTESIAN_POINT('Ctrl Pts',(2.38698271143203,-1.88078189450323,14.5830446809642));
#26288=CARTESIAN_POINT('Ctrl Pts',(2.450785486869,-2.14449521632646,13.7115329395622));
#26289=CARTESIAN_POINT('Ctrl Pts',(2.51953184050711,-2.04937889610162,12.7340785859711));
#26290=CARTESIAN_POINT('Ctrl Pts',(2.58575353157662,-1.51228301440999,11.9296669778702));
#26291=CARTESIAN_POINT('Ctrl Pts',(2.64970641129486,-0.719879659816408,
11.482543891491));
#26292=CARTESIAN_POINT('Ctrl Pts',(2.68414064416519,-0.238646463251669,
11.3992812306547));
#26293=CARTESIAN_POINT('Ctrl Pts',(2.70136633287573,0.00319878278718031,
11.3996354935645));
#26294=CARTESIAN_POINT('Ctrl Pts',(-2.94898729103638,1.05177980826717,11.9577756495737));
#26295=CARTESIAN_POINT('Ctrl Pts',(-2.94455138545693,1.09739106504139,11.9888760681277));
#26296=CARTESIAN_POINT('Ctrl Pts',(-2.918026110446,1.3619620785344,12.186884227221));
#26297=CARTESIAN_POINT('Ctrl Pts',(-2.88904678767022,1.58922760362333,12.4781026097179));
#26298=CARTESIAN_POINT('Ctrl Pts',(-2.86450296461958,1.71300194233482,12.7574567944657));
#26299=CARTESIAN_POINT('Ctrl Pts',(-2.84241355188039,1.8181539629972,13.0114540002238));
#26300=CARTESIAN_POINT('Ctrl Pts',(-2.82277871735286,1.86678055104444,13.2556912711833));
#26301=CARTESIAN_POINT('Ctrl Pts',(-2.79823499734993,1.86676441116482,13.5611506108829));
#26302=CARTESIAN_POINT('Ctrl Pts',(-2.78841749169422,1.86076014318703,13.6833245219451));
#26303=CARTESIAN_POINT('Ctrl Pts',(-2.77369131329709,1.83383161817478,13.8648277310688));
#26304=CARTESIAN_POINT('Ctrl Pts',(-2.76264663035824,1.8003898778738,13.9983167301413));
#26305=CARTESIAN_POINT('Ctrl Pts',(-2.75610165277409,1.77578783700224,14.0759711000829));
#26306=CARTESIAN_POINT('Ctrl Pts',(-2.75119291327835,1.75638332024967,14.1338966609949));
#26307=CARTESIAN_POINT('Ctrl Pts',(-2.74751135937009,1.74024106899155,14.1768014870589));
#26308=CARTESIAN_POINT('Ctrl Pts',(-2.72214954377412,1.61942429167451,14.4683809016479));
#26309=CARTESIAN_POINT('Ctrl Pts',(-2.67797089709577,1.29509438279977,14.9289708470309));
#26310=CARTESIAN_POINT('Ctrl Pts',(-2.6117029268964,0.559739361759716,15.3455116670227));
#26311=CARTESIAN_POINT('Ctrl Pts',(-2.54543495691169,-0.283018800514111,
15.4077039754452));
#26312=CARTESIAN_POINT('Ctrl Pts',(-2.48162135624977,-1.04231371404291,
15.1146741383994));
#26313=CARTESIAN_POINT('Ctrl Pts',(-2.42026212474002,-1.59239241227961,
14.5640775634698));
#26314=CARTESIAN_POINT('Ctrl Pts',(-2.356448523998,-1.90291363513159,13.8160277442462));
#26315=CARTESIAN_POINT('Ctrl Pts',(-2.29754366181465,-1.8658791953148,13.0617489355256));
#26316=CARTESIAN_POINT('Ctrl Pts',(-2.25091064584323,-1.61417795247039,
12.5315062166412));
#26317=CARTESIAN_POINT('Ctrl Pts',(-2.22636695317173,-1.42581820826996,
12.2900866009581));
#26318=CARTESIAN_POINT('Ctrl Pts',(-2.216549476156,-1.34155044848788,12.2015728667815));
#26319=CARTESIAN_POINT('Ctrl Pts',(-2.20918636829416,-1.27674728353269,
12.1367854064728));
#26320=CARTESIAN_POINT('Ctrl Pts',(-2.19446015276218,-1.14079176069474,
12.0135799955576));
#26321=CARTESIAN_POINT('Ctrl Pts',(-2.16009898317316,-0.783580906846267,
11.7746602397536));
#26322=CARTESIAN_POINT('Ctrl Pts',(-2.11101159809488,-0.187782817615464,
11.5939005667503));
#26323=CARTESIAN_POINT('Ctrl Pts',(-2.04719799726984,0.618205729404025,
11.6730712407523));
#26324=CARTESIAN_POINT('Ctrl Pts',(-2.00301935049051,1.10412222965747,11.9640298571025));
#26325=CARTESIAN_POINT('Ctrl Pts',(-1.96129507302961,1.47130954923465,12.331184249062));
#26326=CARTESIAN_POINT('Ctrl Pts',(-1.92693390345156,1.72060698460052,12.6859172796413));
#26327=CARTESIAN_POINT('Ctrl Pts',(-1.86312030263897,1.93730413467564,13.463091044457));
#26328=CARTESIAN_POINT('Ctrl Pts',(-1.7993067017454,1.77565703033136,14.2755679481243));
#26329=CARTESIAN_POINT('Ctrl Pts',(-1.7354931009231,1.27800656389494,14.9106625105529));
#26330=CARTESIAN_POINT('Ctrl Pts',(-1.70113193134735,0.911903775153735,
15.1428819271019));
#26331=CARTESIAN_POINT('Ctrl Pts',(-1.6544989154371,0.375754078194938,15.3654086726963));
#26332=CARTESIAN_POINT('Ctrl Pts',(-1.61032026868658,-0.195009556823064,
15.4208186513374));
#26333=CARTESIAN_POINT('Ctrl Pts',(-1.55141540637949,-0.89287467908256,
15.1699353718112));
#26334=CARTESIAN_POINT('Ctrl Pts',(-1.52196297529924,-1.19044705982738,
14.9495422087379));
#26335=CARTESIAN_POINT('Ctrl Pts',(-1.48760180570641,-1.49280856824171,
14.6471851287901));
#26336=CARTESIAN_POINT('Ctrl Pts',(-1.46796685157482,-1.63114583675639,
14.4400090223007));
#26337=CARTESIAN_POINT('Ctrl Pts',(-1.44342315897332,-1.74805594016706,
14.1578798012588));
#26338=CARTESIAN_POINT('Ctrl Pts',(-1.43606005119052,-1.77895201880203,
14.0714828485797));
#26339=CARTESIAN_POINT('Ctrl Pts',(-1.42133383556671,-1.82784367389418,
13.8948060786019));
#26340=CARTESIAN_POINT('Ctrl Pts',(-1.39188140473377,-1.89083654696875,
13.532670438544));
#26341=CARTESIAN_POINT('Ctrl Pts',(-1.35506586566434,-1.84501027253879,
13.0679371083961));
#26342=CARTESIAN_POINT('Ctrl Pts',(-1.31579595754304,-1.65685861831594,
12.6142668799998));
#26343=CARTESIAN_POINT('Ctrl Pts',(-1.29125226482124,-1.4863996270751,12.3590620417495));
#26344=CARTESIAN_POINT('Ctrl Pts',(-1.27652604934709,-1.36315184596167,
12.223124185907));
#26345=CARTESIAN_POINT('Ctrl Pts',(-1.26179983374059,-1.23356011807307,
12.0935170469981));
#26346=CARTESIAN_POINT('Ctrl Pts',(-1.24216487964064,-1.04375563480033,
11.9377637595064));
#26347=CARTESIAN_POINT('Ctrl Pts',(-1.22252992555137,-0.827209047354781,
11.8220180667511));
#26348=CARTESIAN_POINT('Ctrl Pts',(-1.18326001737828,-0.375738967230657,
11.6346427649014));
#26349=CARTESIAN_POINT('Ctrl Pts',(-1.13662700141788,0.226759583587447,
11.5761502172032));
#26350=CARTESIAN_POINT('Ctrl Pts',(-1.07281340056232,0.978897200444188,
11.867410994966));
#26351=CARTESIAN_POINT('Ctrl Pts',(-1.02372601533608,1.44823540529516,12.2719311266445));
#26352=CARTESIAN_POINT('Ctrl Pts',(-0.991819214989638,1.65456333844798,
12.6164315560303));
#26353=CARTESIAN_POINT('Ctrl Pts',(-0.962366783997792,1.79481940789023,
12.9550584907526));
#26354=CARTESIAN_POINT('Ctrl Pts',(-0.937823091353101,1.86980040908937,
13.2545704979585));
#26355=CARTESIAN_POINT('Ctrl Pts',(-0.908370660191932,1.86972197127684,
13.6228927098112));
#26356=CARTESIAN_POINT('Ctrl Pts',(-0.883826967550878,1.82485010373173,
13.9253917288496));
#26357=CARTESIAN_POINT('Ctrl Pts',(-0.869100752025165,1.77140023412798,
14.1016232582535));
#26358=CARTESIAN_POINT('Ctrl Pts',(-0.856828905671129,1.71295578839072,
14.2427213235411));
#26359=CARTESIAN_POINT('Ctrl Pts',(-0.851920167081815,1.6881868322722,14.2985826390753));
#26360=CARTESIAN_POINT('Ctrl Pts',(-0.842102690140726,1.63324292701848,
14.4077535244));
#26361=CARTESIAN_POINT('Ctrl Pts',(-0.824922105271772,1.52318322321949,
14.5913659007489));
#26362=CARTESIAN_POINT('Ctrl Pts',(-0.81019588976506,1.40636770077858,14.7337299682696));
#26363=CARTESIAN_POINT('Ctrl Pts',(-0.773380350883849,1.08254357632472,
15.0578770878186));
#26364=CARTESIAN_POINT('Ctrl Pts',(-0.719384227226075,0.476127115050851,
15.4011394060682));
#26365=CARTESIAN_POINT('Ctrl Pts',(-0.635935672325424,-0.600610770607247,
15.3747474794605));
#26366=CARTESIAN_POINT('Ctrl Pts',(-0.545124009595912,-1.58296648710691,
14.7195854393962));
#26367=CARTESIAN_POINT('Ctrl Pts',(-0.481310408779742,-1.86744232190721,
13.9276261419255));
#26368=CARTESIAN_POINT('Ctrl Pts',(-0.412588069623317,-1.8674172716517,
13.0722641862657));
#26369=CARTESIAN_POINT('Ctrl Pts',(-0.348774468813634,-1.58289462307497,
12.2803217206137));
#26370=CARTESIAN_POINT('Ctrl Pts',(-0.257962806069509,-0.60050100556019,
11.625218534854));
#26371=CARTESIAN_POINT('Ctrl Pts',(-0.174514251188141,0.476238220638283,
11.5988907922679));
#26372=CARTESIAN_POINT('Ctrl Pts',(-0.1205181275243,1.08263207658234,11.9421915291005));
#26373=CARTESIAN_POINT('Ctrl Pts',(-0.083702588620523,1.40643852814198,
12.266356491699));
#26374=CARTESIAN_POINT('Ctrl Pts',(-0.0714307423348015,1.50377190616919,
12.3850057885532));
#26375=CARTESIAN_POINT('Ctrl Pts',(-0.056704526908075,1.60185605597705,
12.5398795378693));
#26376=CARTESIAN_POINT('Ctrl Pts',(-0.0468870497427143,1.66208392322534,
12.6462265542716));
#26377=CARTESIAN_POINT('Ctrl Pts',(-0.0395239419637206,1.70131215898071,
12.7291604128228));
#26378=CARTESIAN_POINT('Ctrl Pts',(-0.0297064648246382,1.74806119403677,
12.8420424941069));
#26379=CARTESIAN_POINT('Ctrl Pts',(-0.0149802493183748,1.80988609416315,
13.01480660082));
#26380=CARTESIAN_POINT('Ctrl Pts',(0.00956344330796528,1.86973816150673,
13.3158275547878));
#26381=CARTESIAN_POINT('Ctrl Pts',(0.0439246129546704,1.86977391645042,
13.7455383573357));
#26382=CARTESIAN_POINT('Ctrl Pts',(0.0684683055948698,1.7947899917414,14.0450459514158));
#26383=CARTESIAN_POINT('Ctrl Pts',(0.0979207365840127,1.65451257187983,
14.3836645907943));
#26384=CARTESIAN_POINT('Ctrl Pts',(0.129827536933279,1.44816401155227,14.7281533863918));
#26385=CARTESIAN_POINT('Ctrl Pts',(0.178914922159187,0.978801466284751,
15.1326460137714));
#26386=CARTESIAN_POINT('Ctrl Pts',(0.242728523014966,0.226646269966196,
15.4238627618682));
#26387=CARTESIAN_POINT('Ctrl Pts',(0.289361538971896,-0.375848970264699,
15.3653346814543));
#26388=CARTESIAN_POINT('Ctrl Pts',(0.32863144714602,-0.827308050222727,
15.177932788993));
#26389=CARTESIAN_POINT('Ctrl Pts',(0.348266401236533,-1.0438478212656,15.0621743080247));
#26390=CARTESIAN_POINT('Ctrl Pts',(0.367901355336211,-1.2336431249768,14.9064098355125));
#26391=CARTESIAN_POINT('Ctrl Pts',(0.38262757094342,-1.36322719731575,14.7767950409474));
#26392=CARTESIAN_POINT('Ctrl Pts',(0.397353786419115,-1.48646694621212,
14.6408499027268));
#26393=CARTESIAN_POINT('Ctrl Pts',(0.42189747912613,-1.65691087093242,14.3856350125846));
#26394=CARTESIAN_POINT('Ctrl Pts',(0.461167387277872,-1.84503571034646,
13.9319536706252));
#26395=CARTESIAN_POINT('Ctrl Pts',(0.497982926319137,-1.8908345576629,13.4672176837265));
#26396=CARTESIAN_POINT('Ctrl Pts',(0.527435357166049,-1.82782027363552,
13.1050857826764));
#26397=CARTESIAN_POINT('Ctrl Pts',(0.542161572784617,-1.77891817099809,
12.9284119001505));
#26398=CARTESIAN_POINT('Ctrl Pts',(0.549524680568676,-1.74801698741632,
12.8420167796121));
#26399=CARTESIAN_POINT('Ctrl Pts',(0.574068373172529,-1.63109018601349,
12.5598944683743));
#26400=CARTESIAN_POINT('Ctrl Pts',(0.59370332730294,-1.49274070366298,12.3527265616716));
#26401=CARTESIAN_POINT('Ctrl Pts',(0.628064496895538,-1.19036130281273,
12.0503873706824));
#26402=CARTESIAN_POINT('Ctrl Pts',(0.657516927975823,-0.892775905160294,
11.8300118089703));
#26403=CARTESIAN_POINT('Ctrl Pts',(0.716421790282611,-0.194895950072102,
11.5791698109191));
#26404=CARTESIAN_POINT('Ctrl Pts',(0.760600437033626,0.375864414459618,
11.6346135405221));
#26405=CARTESIAN_POINT('Ctrl Pts',(0.807233452943446,0.912000931911337,
11.8571720039664));
#26406=CARTESIAN_POINT('Ctrl Pts',(0.84159462251798,1.27808999763,12.0894130635292));
#26407=CARTESIAN_POINT('Ctrl Pts',(0.905408223341798,1.77570289947956,12.7245370657824));
#26408=CARTESIAN_POINT('Ctrl Pts',(0.969221824234544,1.93730196525167,13.5370235308092));
#26409=CARTESIAN_POINT('Ctrl Pts',(1.03303542504725,1.72055885411322,14.3141844798476));
#26410=CARTESIAN_POINT('Ctrl Pts',(1.06739659462448,1.47124045864297,14.6689027806501));
#26411=CARTESIAN_POINT('Ctrl Pts',(1.10912087208633,1.10403141746053,15.0360354618146));
#26412=CARTESIAN_POINT('Ctrl Pts',(1.1532995188661,0.618097747792482,15.3269653632982));
#26413=CARTESIAN_POINT('Ctrl Pts',(1.21711311969197,-0.187895466307751,
15.4060883879997));
#26414=CARTESIAN_POINT('Ctrl Pts',(1.26620050476972,-0.783682821932288,
15.2252935184613));
#26415=CARTESIAN_POINT('Ctrl Pts',(1.30056167435797,-1.14087952499533,14.9863526540441));
#26416=CARTESIAN_POINT('Ctrl Pts',(1.31528788989013,-1.27682775871608,14.8631392072867));
#26417=CARTESIAN_POINT('Ctrl Pts',(1.32265099775196,-1.34162708887353,14.7983479183875));
#26418=CARTESIAN_POINT('Ctrl Pts',(1.33246847476781,-1.42588961157989,14.709829197654));
#26419=CARTESIAN_POINT('Ctrl Pts',(1.35701216743962,-1.61423505890897,14.4683984701231));
#26420=CARTESIAN_POINT('Ctrl Pts',(1.40364518340993,-1.86590481711679,13.9381409687645));
#26421=CARTESIAN_POINT('Ctrl Pts',(1.46255004559483,-1.90289456011376,13.1838600527939));
#26422=CARTESIAN_POINT('Ctrl Pts',(1.52636364633265,-1.59232869850008,12.4358289376896));
#26423=CARTESIAN_POINT('Ctrl Pts',(1.58772287784506,-1.04221690767433,11.8852653514821));
#26424=CARTESIAN_POINT('Ctrl Pts',(1.65153647850482,-0.282903885450296,
11.5922810835848));
#26425=CARTESIAN_POINT('Ctrl Pts',(1.71780444848671,0.559852308259102,11.6545246982156));
#26426=CARTESIAN_POINT('Ctrl Pts',(1.78407241868674,1.29518426159801,12.0711103352848));
#26427=CARTESIAN_POINT('Ctrl Pts',(1.82825106535847,1.61949044289959,12.5317224786145));
#26428=CARTESIAN_POINT('Ctrl Pts',(1.85361288095202,1.74029071256228,12.8233096457127));
#26429=CARTESIAN_POINT('Ctrl Pts',(1.85729443485987,1.7564305234626,12.8662155716377));
#26430=CARTESIAN_POINT('Ctrl Pts',(1.86220317435584,1.77583158789889,12.9241421695384));
#26431=CARTESIAN_POINT('Ctrl Pts',(1.86874815193976,1.80042917108278,13.0017983055331));
#26432=CARTESIAN_POINT('Ctrl Pts',(1.87979283487919,1.83386347459296,13.135289209121));
#26433=CARTESIAN_POINT('Ctrl Pts',(1.89451901327258,1.86078214523026,13.3167955468064));
#26434=CARTESIAN_POINT('Ctrl Pts',(1.90433651893123,1.86677935000811,13.4389688837803));
#26435=CARTESIAN_POINT('Ctrl Pts',(1.92888023892041,1.86678190805501,13.7444357101596));
#26436=CARTESIAN_POINT('Ctrl Pts',(1.9485150734491,1.8181503635251,13.9886715771723));
#26437=CARTESIAN_POINT('Ctrl Pts',(1.97060448617354,1.71298620579008,14.2426695760738));
#26438=CARTESIAN_POINT('Ctrl Pts',(1.99514830924029,1.58920678796943,14.5220153067922));
#26439=CARTESIAN_POINT('Ctrl Pts',(2.03932655870192,1.24261702068429,14.9659420203183));
#26440=CARTESIAN_POINT('Ctrl Pts',(2.10314071900831,0.528409678047588,15.347741546511));
#26441=CARTESIAN_POINT('Ctrl Pts',(2.16695382561945,-0.282949484886631,
15.4076465636485));
#26442=CARTESIAN_POINT('Ctrl Pts',(2.23567600035159,-1.10090827734288,15.0924424888951));
#26443=CARTESIAN_POINT('Ctrl Pts',(2.30194578184805,-1.6715898090538,14.4625725258841));
#26444=CARTESIAN_POINT('Ctrl Pts',(2.36575487307431,-1.90597096237174,13.6879468659033));
#26445=CARTESIAN_POINT('Ctrl Pts',(2.43448724036195,-1.82145805582818,12.8193214271364));
#26446=CARTESIAN_POINT('Ctrl Pts',(2.50073595296765,-1.34391225562139,12.104238216233));
#26447=CARTESIAN_POINT('Ctrl Pts',(2.56465195236451,-0.63999730751846,11.7070280736045));
#26448=CARTESIAN_POINT('Ctrl Pts',(2.59908792453329,-0.212295699473147,
11.6329768668928));
#26449=CARTESIAN_POINT('Ctrl Pts',(2.61633167011827,0.00284556929259513,
11.6332663792972));
#26450=CARTESIAN_POINT('Ctrl Pts',(-3.03402225960255,0.920169500289213,
12.1508069720949));
#26451=CARTESIAN_POINT('Ctrl Pts',(-3.02958637493129,0.960060201874113,
12.1780263141219));
#26452=CARTESIAN_POINT('Ctrl Pts',(-3.00306118536422,1.1915446741207,12.3512259484075));
#26453=CARTESIAN_POINT('Ctrl Pts',(-2.97408149750605,1.39040704521766,12.6059785856818));
#26454=CARTESIAN_POINT('Ctrl Pts',(-2.94953785715269,1.49860681286232,12.8504237378315));
#26455=CARTESIAN_POINT('Ctrl Pts',(-2.92744856963118,1.59068454416991,13.072587592917));
#26456=CARTESIAN_POINT('Ctrl Pts',(-2.90781356757833,1.63313005912254,13.2863194450445));
#26457=CARTESIAN_POINT('Ctrl Pts',(-2.88326988588137,1.63312353621953,13.553521441343));
#26458=CARTESIAN_POINT('Ctrl Pts',(-2.87345242031875,1.62786623540166,13.6604114149956));
#26459=CARTESIAN_POINT('Ctrl Pts',(-2.85872618992664,1.60430567893626,13.8191933720227));
#26460=CARTESIAN_POINT('Ctrl Pts',(-2.84768153693031,1.57504838849142,13.9359780710016));
#26461=CARTESIAN_POINT('Ctrl Pts',(-2.84113654943735,1.55352166107146,14.0039114130109));
#26462=CARTESIAN_POINT('Ctrl Pts',(-2.83622781122445,1.53655095176889,14.0545888622835));
#26463=CARTESIAN_POINT('Ctrl Pts',(-2.83254625727853,1.52241574345267,14.0921204234963));
#26464=CARTESIAN_POINT('Ctrl Pts',(-2.80718444145174,1.41678309361852,14.347226232301));
#26465=CARTESIAN_POINT('Ctrl Pts',(-2.76300579467544,1.1329635040614,14.7501457186005));
#26466=CARTESIAN_POINT('Ctrl Pts',(-2.6967378246562,0.489672671131416,15.114548514947));
#26467=CARTESIAN_POINT('Ctrl Pts',(-2.63046985464307,-0.247633377770316,
15.1689412363303));
#26468=CARTESIAN_POINT('Ctrl Pts',(-2.56665625390239,-0.911884404744357,
14.912574079968));
#26469=CARTESIAN_POINT('Ctrl Pts',(-2.50529702242643,-1.39312343471216,
14.4308757228267));
#26470=CARTESIAN_POINT('Ctrl Pts',(-2.44148342171928,-1.66473450900518,
13.7764493906401));
#26471=CARTESIAN_POINT('Ctrl Pts',(-2.38257855943633,-1.63236162107275,
13.1165653158355));
#26472=CARTESIAN_POINT('Ctrl Pts',(-2.33594554353368,-1.41209346995343,
12.6526975531263));
#26473=CARTESIAN_POINT('Ctrl Pts',(-2.31140185087204,-1.24738462820272,
12.441488964872));
#26474=CARTESIAN_POINT('Ctrl Pts',(-2.30158437381822,-1.17361718385254,
12.3640600256991));
#26475=CARTESIAN_POINT('Ctrl Pts',(-2.29422126594484,-1.11693960792093,
12.3073698470986));
#26476=CARTESIAN_POINT('Ctrl Pts',(-2.27949505045088,-0.997986048126505,
12.1996129366123));
#26477=CARTESIAN_POINT('Ctrl Pts',(-2.24513388086172,-0.685485933856807,
11.990568875841));
#26478=CARTESIAN_POINT('Ctrl Pts',(-2.19604649576334,-0.164254747381628,
11.8324394379657));
#26479=CARTESIAN_POINT('Ctrl Pts',(-2.13223289491963,0.540869967667105,
11.9017559617062));
#26480=CARTESIAN_POINT('Ctrl Pts',(-2.08805424818418,0.96595860097193,12.15620272179));
#26481=CARTESIAN_POINT('Ctrl Pts',(-2.04632997072101,1.28720491445197,12.4775422504944));
#26482=CARTESIAN_POINT('Ctrl Pts',(-2.01196880112813,1.50523979116393,12.787800305018));
#26483=CARTESIAN_POINT('Ctrl Pts',(-1.9481552002848,1.69484966835682,13.4677675453008));
#26484=CARTESIAN_POINT('Ctrl Pts',(-1.88434159947337,1.55342731976602,14.1785043884778));
#26485=CARTESIAN_POINT('Ctrl Pts',(-1.82052799863252,1.11799586960201,14.734156071574));
#26486=CARTESIAN_POINT('Ctrl Pts',(-1.78616682903858,0.797785855142485,
14.9372200074867));
#26487=CARTESIAN_POINT('Ctrl Pts',(-1.73953381311012,0.328667738149594,
15.1320217157569));
#26488=CARTESIAN_POINT('Ctrl Pts',(-1.69535516636144,-0.170611178336508,
15.1804155041868));
#26489=CARTESIAN_POINT('Ctrl Pts',(-1.63645030412725,-0.781168837678439,
14.9608972194216));
#26490=CARTESIAN_POINT('Ctrl Pts',(-1.60699787298018,-1.04147077861518,
14.7681600649693));
#26491=CARTESIAN_POINT('Ctrl Pts',(-1.57263670339236,-1.30600071406174,
14.5035081513716));
#26492=CARTESIAN_POINT('Ctrl Pts',(-1.55300174932564,-1.42706109438727,
14.3224484754254));
#26493=CARTESIAN_POINT('Ctrl Pts',(-1.52845805663552,-1.52927263928429,
14.0754974223444));
#26494=CARTESIAN_POINT('Ctrl Pts',(-1.5210949488129,-1.55633041503445,13.9999388879625));
#26495=CARTESIAN_POINT('Ctrl Pts',(-1.50636873335532,-1.59905869561866,
13.8453662892381));
#26496=CARTESIAN_POINT('Ctrl Pts',(-1.47691630227588,-1.6542250679665,13.5285538081163));
#26497=CARTESIAN_POINT('Ctrl Pts',(-1.44010076338987,-1.61409287864128,
13.1219913011565));
#26498=CARTESIAN_POINT('Ctrl Pts',(-1.40083085520029,-1.44947263129895,
12.7251021192302));
#26499=CARTESIAN_POINT('Ctrl Pts',(-1.37628716255761,-1.30035750492487,
12.5018492233465));
#26500=CARTESIAN_POINT('Ctrl Pts',(-1.36156094704064,-1.19252072049869,
12.3829141693026));
#26501=CARTESIAN_POINT('Ctrl Pts',(-1.34683473141102,-1.07915009456125,
12.2695686129219));
#26502=CARTESIAN_POINT('Ctrl Pts',(-1.32719977733342,-0.913103031170408,
12.133210596805));
#26503=CARTESIAN_POINT('Ctrl Pts',(-1.30756482324941,-0.723643206763342,
12.0320965600779));
#26504=CARTESIAN_POINT('Ctrl Pts',(-1.26829491508155,-0.328701273622561,
11.8679559538835));
#26505=CARTESIAN_POINT('Ctrl Pts',(-1.22166189909103,0.198416733304813,
11.8169893707361));
#26506=CARTESIAN_POINT('Ctrl Pts',(-1.157848298264,0.856403344125254,12.0717207142664));
#26507=CARTESIAN_POINT('Ctrl Pts',(-1.10876091305799,1.26700075008309,12.4256347119853));
#26508=CARTESIAN_POINT('Ctrl Pts',(-1.07685411269456,1.44749324226499,12.7270434153079));
#26509=CARTESIAN_POINT('Ctrl Pts',(-1.04740168167682,1.57019859096341,13.0232635734239));
#26510=CARTESIAN_POINT('Ctrl Pts',(-1.0228579890047,1.63578404034369,13.2853111623653));
#26511=CARTESIAN_POINT('Ctrl Pts',(-0.993405557890351,1.63571078832615,
13.6075244739282));
#26512=CARTESIAN_POINT('Ctrl Pts',(-0.968861865215506,1.59644882660007,
13.8721669546422));
#26513=CARTESIAN_POINT('Ctrl Pts',(-0.954135649719787,1.54969090536267,
14.0263393865899));
#26514=CARTESIAN_POINT('Ctrl Pts',(-0.941863803395456,1.49855089459867,
14.1497739523841));
#26515=CARTESIAN_POINT('Ctrl Pts',(-0.936955064818857,1.47689087177173,
14.1986510834065));
#26516=CARTESIAN_POINT('Ctrl Pts',(-0.927137587735728,1.42880164807781,
14.2941407780118));
#26517=CARTESIAN_POINT('Ctrl Pts',(-0.909957002971033,1.33255530220944,
14.4548060833212));
#26518=CARTESIAN_POINT('Ctrl Pts',(-0.895230787466278,1.23029481064996,
14.579294205637));
#26519=CARTESIAN_POINT('Ctrl Pts',(-0.858415248587724,0.947092495740584,
14.8629563894098));
#26520=CARTESIAN_POINT('Ctrl Pts',(-0.804419124905459,0.416471133153839,
15.1631213076161));
#26521=CARTESIAN_POINT('Ctrl Pts',(-0.720970569978194,-0.525431236881228,
15.140193552971));
#26522=CARTESIAN_POINT('Ctrl Pts',(-0.630158907329698,-1.38487944782349,
14.566900993129));
#26523=CARTESIAN_POINT('Ctrl Pts',(-0.566345306486509,-1.63374111356011,
13.8741088568859));
#26524=CARTESIAN_POINT('Ctrl Pts',(-0.497622967298252,-1.63370556065679,
13.1257367092235));
#26525=CARTESIAN_POINT('Ctrl Pts',(-0.433809366452732,-1.3847789726291,
12.4329685854038));
#26526=CARTESIAN_POINT('Ctrl Pts',(-0.342997703809482,-0.52527584557229,
11.8597571249176));
#26527=CARTESIAN_POINT('Ctrl Pts',(-0.259549148874224,0.416626540888193,
11.836920727128));
#26528=CARTESIAN_POINT('Ctrl Pts',(-0.205553025194717,0.947221216760767,
12.1371347585086));
#26529=CARTESIAN_POINT('Ctrl Pts',(-0.168737486325147,1.23039239167878,
12.4208275322826));
#26530=CARTESIAN_POINT('Ctrl Pts',(-0.156465640055685,1.31561190938362,
12.5245660427945));
#26531=CARTESIAN_POINT('Ctrl Pts',(-0.141739424519946,1.40137424309293,
12.6600952641544));
#26532=CARTESIAN_POINT('Ctrl Pts',(-0.131921947526936,1.45408325127083,
12.7531152215987));
#26533=CARTESIAN_POINT('Ctrl Pts',(-0.124558839702545,1.48838774933109,
12.8256813917505));
#26534=CARTESIAN_POINT('Ctrl Pts',(-0.114741362533611,1.52928697674707,
12.9244326285369));
#26535=CARTESIAN_POINT('Ctrl Pts',(-0.100015147029465,1.58337337161512,
13.0755740476735));
#26536=CARTESIAN_POINT('Ctrl Pts',(-0.0754714543489009,1.63572924411331,
13.3389245508721));
#26537=CARTESIAN_POINT('Ctrl Pts',(-0.0411102847817865,1.63575335187083,
13.7148439986148));
#26538=CARTESIAN_POINT('Ctrl Pts',(-0.0165665921072617,1.5701561760943,
13.9768836663726));
#26539=CARTESIAN_POINT('Ctrl Pts',(0.0128858389111597,1.44742050019548,
14.2730929097655));
#26540=CARTESIAN_POINT('Ctrl Pts',(0.0447926392720795,1.26690003118422,
14.5744844766074));
#26541=CARTESIAN_POINT('Ctrl Pts',(0.0938800244804459,0.856268351960268,
14.9283599556911));
#26542=CARTESIAN_POINT('Ctrl Pts',(0.157693625306139,0.198257586748516,
15.1830290881431));
#26543=CARTESIAN_POINT('Ctrl Pts',(0.204326641297953,-0.328855799025312,
15.132012690545));
#26544=CARTESIAN_POINT('Ctrl Pts',(0.243596549465899,-0.723782207149813,
14.9678346732507));
#26545=CARTESIAN_POINT('Ctrl Pts',(0.263231503548857,-0.913232470143678,
14.8667027120325));
#26546=CARTESIAN_POINT('Ctrl Pts',(0.282866457627509,-1.07926662259235,
14.7303289658635));
#26547=CARTESIAN_POINT('Ctrl Pts',(0.297592673256385,-1.19262651054228,
14.6169726725508));
#26548=CARTESIAN_POINT('Ctrl Pts',(0.312318888772827,-1.30045202310849,
14.4980274007988));
#26549=CARTESIAN_POINT('Ctrl Pts',(0.336862581421082,-1.44954600310508,
14.2747603872182));
#26550=CARTESIAN_POINT('Ctrl Pts',(0.376132489598524,-1.61412863338867,
13.8778556113047));
#26551=CARTESIAN_POINT('Ctrl Pts',(0.412948028495775,-1.65422231886617,
13.4712893453838));
#26552=CARTESIAN_POINT('Ctrl Pts',(0.442400459570104,-1.59902591563155,
13.1544820886784));
#26553=CARTESIAN_POINT('Ctrl Pts',(0.457126675029423,-1.55628298468981,
12.9999135484931));
#26554=CARTESIAN_POINT('Ctrl Pts',(0.464489782851631,-1.52921804275104,
12.9243575754456));
#26555=CARTESIAN_POINT('Ctrl Pts',(0.489033475541114,-1.42698310993751,
12.6774162249364));
#26556=CARTESIAN_POINT('Ctrl Pts',(0.508668429607991,-1.305905545711,12.4963680285754));
#26557=CARTESIAN_POINT('Ctrl Pts',(0.543029599196515,-1.04135054659198,
12.2317411943687));
#26558=CARTESIAN_POINT('Ctrl Pts',(0.572482030342974,-0.781030328084433,
12.0390287250993));
#26559=CARTESIAN_POINT('Ctrl Pts',(0.631386892576705,-0.170451869762501,
11.8195683188816));
#26560=CARTESIAN_POINT('Ctrl Pts',(0.675565539326545,0.328822445454624,
11.8680094482727));
#26561=CARTESIAN_POINT('Ctrl Pts',(0.722198555253912,0.79792211316962,12.062855618652));
#26562=CARTESIAN_POINT('Ctrl Pts',(0.756559724849884,1.11811286227706,12.2659499226733));
#26563=CARTESIAN_POINT('Ctrl Pts',(0.82037332568896,1.55349164464191,12.8216428751273));
#26564=CARTESIAN_POINT('Ctrl Pts',(0.884186926500656,1.69484661024464,13.5323931254781));
#26565=CARTESIAN_POINT('Ctrl Pts',(0.948000527344836,1.5051722882597,14.2123423996626));
#26566=CARTESIAN_POINT('Ctrl Pts',(0.982361696939161,1.28710799282076,14.5225797792344));
#26567=CARTESIAN_POINT('Ctrl Pts',(1.02408597439874,0.965831243986841,14.8438888609862));
#26568=CARTESIAN_POINT('Ctrl Pts',(1.0682646211369,0.540718491046902,15.0982953355625));
#26569=CARTESIAN_POINT('Ctrl Pts',(1.13207822197524,-0.164412771655819,
15.1675450274765));
#26570=CARTESIAN_POINT('Ctrl Pts',(1.1811656070763,-0.685628935442496,15.0093662035735));
#26571=CARTESIAN_POINT('Ctrl Pts',(1.2155267766664,-0.9981092245177,14.8002925280399));
#26572=CARTESIAN_POINT('Ctrl Pts',(1.23025299216004,-1.11705256006795,14.6925243471944));
#26573=CARTESIAN_POINT('Ctrl Pts',(1.23761610003377,-1.17372476231246,14.6358287944356));
#26574=CARTESIAN_POINT('Ctrl Pts',(1.24743357708706,-1.24748486299388,14.5583928713913));
#26575=CARTESIAN_POINT('Ctrl Pts',(1.27197726974902,-1.41217366984488,14.3471686686388));
#26576=CARTESIAN_POINT('Ctrl Pts',(1.31861028565164,-1.63239775437311,13.8832801106741));
#26577=CARTESIAN_POINT('Ctrl Pts',(1.37751514793352,-1.66470802437629,13.2233930149844));
#26578=CARTESIAN_POINT('Ctrl Pts',(1.44132874864127,-1.39303462659156,12.5689926739555));
#26579=CARTESIAN_POINT('Ctrl Pts',(1.50268798011341,-0.911749558144166,
12.0873402447523));
#26580=CARTESIAN_POINT('Ctrl Pts',(1.56650158085077,-0.247473676131264,
11.8310365165478));
#26581=CARTESIAN_POINT('Ctrl Pts',(1.63276955086017,0.489828424940365,11.8855001177392));
#26582=CARTESIAN_POINT('Ctrl Pts',(1.69903752086455,1.1330858275586,12.2499648183537));
#26583=CARTESIAN_POINT('Ctrl Pts',(1.7432161676295,1.4168696997825,12.6529132192007));
#26584=CARTESIAN_POINT('Ctrl Pts',(1.76857798345518,1.52247870518676,12.9080295053983));
#26585=CARTESIAN_POINT('Ctrl Pts',(1.77225953740107,1.53661037226812,12.9455623561621));
#26586=CARTESIAN_POINT('Ctrl Pts',(1.77716827561365,1.55357633118333,12.9962415414666));
#26587=CARTESIAN_POINT('Ctrl Pts',(1.78371326310664,1.57509655384721,13.0641767165963));
#26588=CARTESIAN_POINT('Ctrl Pts',(1.79475791609898,1.60434347759022,13.1809651080057));
#26589=CARTESIAN_POINT('Ctrl Pts',(1.80948414649115,1.62788896182785,13.3397487002929));
#26590=CARTESIAN_POINT('Ctrl Pts',(1.819301612048,1.63313712936035,13.4466409112928));
#26591=CARTESIAN_POINT('Ctrl Pts',(1.84384529374514,1.63311844824755,13.7138391645349));
#26592=CARTESIAN_POINT('Ctrl Pts',(1.8634802957282,1.59066474212537,13.9275836013987));
#26593=CARTESIAN_POINT('Ctrl Pts',(1.8855695832519,1.49856463863765,14.1497336983763));
#26594=CARTESIAN_POINT('Ctrl Pts',(1.91011322357714,1.39035745604533,14.394184386848));
#26595=CARTESIAN_POINT('Ctrl Pts',(1.9542920295924,1.08705021048906,14.7824621967109));
#26596=CARTESIAN_POINT('Ctrl Pts',(2.01810540570555,0.462273209156912,15.1165143307525));
#26597=CARTESIAN_POINT('Ctrl Pts',(2.08191920435414,-0.247571374664457,
15.1688755025031));
#26598=CARTESIAN_POINT('Ctrl Pts',(2.15064160895298,-0.96311444391493,14.8931256206334));
#26599=CARTESIAN_POINT('Ctrl Pts',(2.2169088515672,-1.46241536607307,14.3420807405149));
#26600=CARTESIAN_POINT('Ctrl Pts',(2.28072425635766,-1.66732177281756,13.6643462346872));
#26601=CARTESIAN_POINT('Ctrl Pts',(2.34944263886444,-1.59359430353533,12.9045702858734));
#26602=CARTESIAN_POINT('Ctrl Pts',(2.41571836748289,-1.17545546442057,12.2787031132114));
#26603=CARTESIAN_POINT('Ctrl Pts',(2.47959749132094,-0.560059618033885,
11.9315903996426));
#26604=CARTESIAN_POINT('Ctrl Pts',(2.51403518517295,-0.185684347821608,
11.86658222976));
#26605=CARTESIAN_POINT('Ctrl Pts',(2.53129700762356,0.00248888451629452,
11.8668984646848));
#26606=CARTESIAN_POINT('Ctrl Pts',(-3.11905722816867,0.788556068408818,
12.3438412372351));
#26607=CARTESIAN_POINT('Ctrl Pts',(-3.1146213644059,0.822744462661041,12.3671622765409));
#26608=CARTESIAN_POINT('Ctrl Pts',(-3.08809626028157,1.02109524199808,12.515601306046));
#26609=CARTESIAN_POINT('Ctrl Pts',(-3.05911620734098,1.19148646818497,12.7339291160136));
#26610=CARTESIAN_POINT('Ctrl Pts',(-3.0345727496855,1.28423698062874,12.9433793370522));
#26611=CARTESIAN_POINT('Ctrl Pts',(-3.012483587381,1.36309551648216,13.1337811072441));
#26612=CARTESIAN_POINT('Ctrl Pts',(-2.99284841780566,1.39950709934089,13.316912415425));
#26613=CARTESIAN_POINT('Ctrl Pts',(-2.96830477441331,1.3994903573956,13.5459004268723));
#26614=CARTESIAN_POINT('Ctrl Pts',(-2.95848734894396,1.39498429573084,13.6374947293668));
#26615=CARTESIAN_POINT('Ctrl Pts',(-2.94376106655668,1.3747906388216,13.7735640779168));
#26616=CARTESIAN_POINT('Ctrl Pts',(-2.93271644350277,1.34971611395508,13.8736390201562));
#26617=CARTESIAN_POINT('Ctrl Pts',(-2.92617144610105,1.3312687232855,13.9318544049706));
#26618=CARTESIAN_POINT('Ctrl Pts',(-2.92126270917083,1.31672200136771,13.975280722022));
#26619=CARTESIAN_POINT('Ctrl Pts',(-2.91758115518753,1.30461397165259,14.0074442312418));
#26620=CARTESIAN_POINT('Ctrl Pts',(-2.89221933912803,1.21405681112827,14.2260429153886));
#26621=CARTESIAN_POINT('Ctrl Pts',(-2.84804069224887,0.970866105212703,
14.571324307522));
#26622=CARTESIAN_POINT('Ctrl Pts',(-2.78177272242044,0.419579819813183,
14.8835800117351));
#26623=CARTESIAN_POINT('Ctrl Pts',(-2.71550475237441,-0.212238228752434,
14.9301775586545));
#26624=CARTESIAN_POINT('Ctrl Pts',(-2.65169115155633,-0.781460863156941,
14.7104725350107));
#26625=CARTESIAN_POINT('Ctrl Pts',(-2.59033192011683,-1.19383767178126,
14.2976774875137));
#26626=CARTESIAN_POINT('Ctrl Pts',(-2.52651831944052,-1.42659490494421,
13.7368649239659));
#26627=CARTESIAN_POINT('Ctrl Pts',(-2.46761345705901,-1.39882228600251,
13.1713879038669));
#26628=CARTESIAN_POINT('Ctrl Pts',(-2.42098044122426,-1.21008384706513,
12.7738815820048));
#26629=CARTESIAN_POINT('Ctrl Pts',(-2.39643674857055,-1.0688970240368,12.5928949266493));
#26630=CARTESIAN_POINT('Ctrl Pts',(-2.38661927148008,-1.00570170912655,
12.5265419204679));
#26631=CARTESIAN_POINT('Ctrl Pts',(-2.37925616359409,-0.957123856235339,
12.4779685781114));
#26632=CARTESIAN_POINT('Ctrl Pts',(-2.36452994813932,-0.855190907485222,
12.3856175840845));
#26633=CARTESIAN_POINT('Ctrl Pts',(-2.33016877854912,-0.587389200609479,
12.206500313161));
#26634=CARTESIAN_POINT('Ctrl Pts',(-2.2810813934289,-0.14072084325576,12.0710044028659));
#26635=CARTESIAN_POINT('Ctrl Pts',(-2.21726779257138,0.463522436140825,
12.13039969068));
#26636=CARTESIAN_POINT('Ctrl Pts',(-2.1730891458758,0.827796642395821,12.3485019022086));
#26637=CARTESIAN_POINT('Ctrl Pts',(-2.13136486841596,1.10306977224913,12.6238173312992));
#26638=CARTESIAN_POINT('Ctrl Pts',(-2.09700369880523,1.28993205121074,12.8897320616277));
#26639=CARTESIAN_POINT('Ctrl Pts',(-2.03319009793237,1.45238162030186,13.4724009101037));
#26640=CARTESIAN_POINT('Ctrl Pts',(-1.96937649720154,1.3311736718366,14.0814808009882));
#26641=CARTESIAN_POINT('Ctrl Pts',(-1.9055628963443,0.958048639865271,14.5576091879427));
#26642=CARTESIAN_POINT('Ctrl Pts',(-1.87120172672977,0.683608478280005,
14.7316558797277));
#26643=CARTESIAN_POINT('Ctrl Pts',(-1.82456871078427,0.281628953814897,
14.8985184663949));
#26644=CARTESIAN_POINT('Ctrl Pts',(-1.78039006403628,-0.146247864930105,
14.9400120756112));
#26645=CARTESIAN_POINT('Ctrl Pts',(-1.72148520187501,-0.669437462685373,
14.7518963321265));
#26646=CARTESIAN_POINT('Ctrl Pts',(-1.6920327706614,-0.892507874178498,
14.5866913693728));
#26647=CARTESIAN_POINT('Ctrl Pts',(-1.65767160107852,-1.11918184099976,
14.3599554485608));
#26648=CARTESIAN_POINT('Ctrl Pts',(-1.6380366470776,-1.22290134327235,14.2047088389408));
#26649=CARTESIAN_POINT('Ctrl Pts',(-1.61349295429772,-1.31051403112513,
13.9931440110592));
#26650=CARTESIAN_POINT('Ctrl Pts',(-1.60612984643543,-1.33368570763948,
13.9283824504914));
#26651=CARTESIAN_POINT('Ctrl Pts',(-1.59140363114421,-1.37031719534642,
13.7959253448278));
#26652=CARTESIAN_POINT('Ctrl Pts',(-1.56195119981817,-1.41755613457247,
13.5244343938463));
#26653=CARTESIAN_POINT('Ctrl Pts',(-1.52513566111425,-1.38317257118645,
13.1760325375352));
#26654=CARTESIAN_POINT('Ctrl Pts',(-1.48586575285738,-1.24209919728576,
12.8359260637791));
#26655=CARTESIAN_POINT('Ctrl Pts',(-1.46132206029344,-1.11430546792535,
12.6446105506962));
#26656=CARTESIAN_POINT('Ctrl Pts',(-1.44659584473411,-1.02189885312362,
12.5426982172715));
#26657=CARTESIAN_POINT('Ctrl Pts',(-1.43186962908097,-0.924742834190651,
12.445552486113));
#26658=CARTESIAN_POINT('Ctrl Pts',(-1.4122346750253,-0.782445427376674,
12.3287514970302));
#26659=CARTESIAN_POINT('Ctrl Pts',(-1.39259972094758,-0.620093737820679,
12.2420415398033));
#26660=CARTESIAN_POINT('Ctrl Pts',(-1.35332981278393,-0.281636263334788,
12.1014932572049));
#26661=CARTESIAN_POINT('Ctrl Pts',(-1.30669679676423,0.17006225243843,12.0577388887696));
#26662=CARTESIAN_POINT('Ctrl Pts',(-1.24288319596633,0.733918023717241,
12.2760823434877));
#26663=CARTESIAN_POINT('Ctrl Pts',(-1.19379581077855,1.08576568076314,12.5793672935782));
#26664=CARTESIAN_POINT('Ctrl Pts',(-1.16188901039935,1.24043405633174,12.8376505666888));
#26665=CARTESIAN_POINT('Ctrl Pts',(-1.13243657935689,1.34557535185587,13.0915089017486));
#26666=CARTESIAN_POINT('Ctrl Pts',(-1.10789288665632,1.40177585596813,13.3160602501166));
#26667=CARTESIAN_POINT('Ctrl Pts',(-1.07844045558897,1.40170600578177,13.5921830605853));
#26668=CARTESIAN_POINT('Ctrl Pts',(-1.05389676288062,1.36805606273619,13.8189634607861));
#26669=CARTESIAN_POINT('Ctrl Pts',(-1.03917054741413,1.32798180613147,13.9510799754394));
#26670=CARTESIAN_POINT('Ctrl Pts',(-1.02689870111988,1.2841590185032,14.0568565549943));
#26671=CARTESIAN_POINT('Ctrl Pts',(-1.02198996255573,1.26559216632164,14.0987374408959));
#26672=CARTESIAN_POINT('Ctrl Pts',(-1.01217248533102,1.22438985324433,14.1805732328973));
#26673=CARTESIAN_POINT('Ctrl Pts',(-0.994991900669837,1.14189010858655,
14.318235939556));
#26674=CARTESIAN_POINT('Ctrl Pts',(-0.980265685167946,1.05428522966142,
14.424938644877));
#26675=CARTESIAN_POINT('Ctrl Pts',(-0.943450146291098,0.811546794400914,
14.6679737141968));
#26676=CARTESIAN_POINT('Ctrl Pts',(-0.889454022585424,0.356873734737775,
14.9252444568342));
#26677=CARTESIAN_POINT('Ctrl Pts',(-0.806005467631,-0.450314585645347,14.9054960137471));
#26678=CARTESIAN_POINT('Ctrl Pts',(-0.715193805062034,-1.1867759283488,
14.4142524142852));
#26679=CARTESIAN_POINT('Ctrl Pts',(-0.651380204193698,-1.40002055950109,
13.8205412187184));
#26680=CARTESIAN_POINT('Ctrl Pts',(-0.582657864972822,-1.39997497623281,
13.1792599528847));
#26681=CARTESIAN_POINT('Ctrl Pts',(-0.518844264092402,-1.18664613215041,
12.585579291146));
#26682=CARTESIAN_POINT('Ctrl Pts',(-0.428032601549523,-0.450114970484183,
12.094440696976));
#26683=CARTESIAN_POINT('Ctrl Pts',(-0.344584046560112,0.357075207419309,
12.0748081953586));
#26684=CARTESIAN_POINT('Ctrl Pts',(-0.290587922865303,0.811711418684831,
12.3321442177636));
#26685=CARTESIAN_POINT('Ctrl Pts',(-0.253772384029816,1.05441415769597,
12.5752148091857));
#26686=CARTESIAN_POINT('Ctrl Pts',(-0.241500537777015,1.12740810231216,
12.6641430019001));
#26687=CARTESIAN_POINT('Ctrl Pts',(-0.226774322131749,1.20091854863098,
12.7802681504964));
#26688=CARTESIAN_POINT('Ctrl Pts',(-0.216956845311384,1.24607566691818,
12.8599900719375));
#26689=CARTESIAN_POINT('Ctrl Pts',(-0.20959373744137,1.2754769729967,12.9221704644164));
#26690=CARTESIAN_POINT('Ctrl Pts',(-0.199776260242763,1.31052185463136,
13.0067969486097));
#26691=CARTESIAN_POINT('Ctrl Pts',(-0.185050044740512,1.35686671439483,
13.1363178263613));
#26692=CARTESIAN_POINT('Ctrl Pts',(-0.160506352005717,1.40172752399848,
13.3619931910802));
#26693=CARTESIAN_POINT('Ctrl Pts',(-0.126145182518741,1.40174073623245,
13.6841386578387));
#26694=CARTESIAN_POINT('Ctrl Pts',(-0.101601489808506,1.34551942205644,
13.908681333809));
#26695=CARTESIAN_POINT('Ctrl Pts',(-0.072149058762419,1.240340560484,14.1625249842377));
#26696=CARTESIAN_POINT('Ctrl Pts',(-0.0402422583875128,1.08563555157988,
14.4207864531663));
#26697=CARTESIAN_POINT('Ctrl Pts',(0.00884512680068361,0.733744263865131,
14.7240215729494));
#26698=CARTESIAN_POINT('Ctrl Pts',(0.0726587275984066,0.169857268657729,
14.9422849993108));
#26699=CARTESIAN_POINT('Ctrl Pts',(0.119291743623238,-0.281835160449523,
14.8984664262192));
#26700=CARTESIAN_POINT('Ctrl Pts',(0.158561651785726,-0.620272668097745,
14.7578700153382));
#26701=CARTESIAN_POINT('Ctrl Pts',(0.178196605860647,-0.78261203441093,
14.6711369668772));
#26702=CARTESIAN_POINT('Ctrl Pts',(0.197831559918322,-0.924892829664357,
14.5543157409681));
#26703=CARTESIAN_POINT('Ctrl Pts',(0.212557775569124,-1.02203502447049,
14.4571561863723));
#26704=CARTESIAN_POINT('Ctrl Pts',(0.227283991125964,-1.11442713372381,
14.3552307026066));
#26705=CARTESIAN_POINT('Ctrl Pts',(0.251827683716028,-1.24219364322043,
14.1638970162314));
#26706=CARTESIAN_POINT('Ctrl Pts',(0.291097591917902,-1.38321860530081,
13.8237704716166));
#26707=CARTESIAN_POINT('Ctrl Pts',(0.327913130672672,-1.41755260632012,
13.4753637614126));
#26708=CARTESIAN_POINT('Ctrl Pts',(0.357365561974734,-1.3702750193093,13.2038795417306));
#26709=CARTESIAN_POINT('Ctrl Pts',(0.372091777274669,-1.33362467627383,
13.0714276531952));
#26710=CARTESIAN_POINT('Ctrl Pts',(0.379454885135005,-1.31044378071783,
13.0066693926929));
#26711=CARTESIAN_POINT('Ctrl Pts',(0.403998577910522,-1.22280097664773,
12.7951170424732));
#26712=CARTESIAN_POINT('Ctrl Pts',(0.423633531913512,-1.11905938241173,
12.6398852089949));
#26713=CARTESIAN_POINT('Ctrl Pts',(0.457994701498026,-0.892353142221933,
12.4131815643651));
#26714=CARTESIAN_POINT('Ctrl Pts',(0.487447132710345,-0.66925921781202,
12.2480083652116));
#26715=CARTESIAN_POINT('Ctrl Pts',(0.546351994870958,-0.146042848998138,
12.0599671108965));
#26716=CARTESIAN_POINT('Ctrl Pts',(0.590530641619899,0.281828057894891,
12.1015216368775));
#26717=CARTESIAN_POINT('Ctrl Pts',(0.637163657564549,0.683783822214472,
12.2684414511951));
#26718=CARTESIAN_POINT('Ctrl Pts',(0.67152482718102,0.958199202226451,12.4425272138518));
#26719=CARTESIAN_POINT('Ctrl Pts',(0.735338428036789,1.33125644777318,12.9187087178781));
#26720=CARTESIAN_POINT('Ctrl Pts',(0.799152028767091,1.45237768566226,13.5278058611153));
#26721=CARTESIAN_POINT('Ctrl Pts',(0.862965629641978,1.28984517196703,14.1104515813163));
#26722=CARTESIAN_POINT('Ctrl Pts',(0.897326799254478,1.10294504271018,14.3763397106384));
#26723=CARTESIAN_POINT('Ctrl Pts',(0.93905107671091,0.827632726114737,14.6516159527686));
#26724=CARTESIAN_POINT('Ctrl Pts',(0.983229723407923,0.463327489001278,
14.8696663168148));
#26725=CARTESIAN_POINT('Ctrl Pts',(1.04704332425977,-0.140924226201367,
14.9289755924517));
#26726=CARTESIAN_POINT('Ctrl Pts',(1.09613070938308,-0.587573258897613,
14.793416119096));
#26727=CARTESIAN_POINT('Ctrl Pts',(1.13049187897521,-0.855349451405556,
14.614260734394));
#26728=CARTESIAN_POINT('Ctrl Pts',(1.14521809443,-0.957269247127293,14.5218952336081));
#26729=CARTESIAN_POINT('Ctrl Pts',(1.15258120231606,-1.00584018321824,14.4733149769537));
#26730=CARTESIAN_POINT('Ctrl Pts',(1.16239867940624,-1.06902604877892,14.4069529765618));
#26731=CARTESIAN_POINT('Ctrl Pts',(1.18694237205925,-1.21018709119309,14.2259462340624));
#26732=CARTESIAN_POINT('Ctrl Pts',(1.23357538789392,-1.39886884688823,13.8284131208944));
#26733=CARTESIAN_POINT('Ctrl Pts',(1.29248025027432,-1.42656089820532,13.2629322038511));
#26734=CARTESIAN_POINT('Ctrl Pts',(1.35629385095077,-1.19372354209459,12.7021530167634));
#26735=CARTESIAN_POINT('Ctrl Pts',(1.41765308238647,-0.781287592708931,
12.2894169897012));
#26736=CARTESIAN_POINT('Ctrl Pts',(1.4814666832016,-0.212033131166725,12.0697934600203));
#26737=CARTESIAN_POINT('Ctrl Pts',(1.5477346532436,0.419779491092501,12.1164819470839));
#26738=CARTESIAN_POINT('Ctrl Pts',(1.61400262305684,0.971022431641602,12.4288170433353));
#26739=CARTESIAN_POINT('Ctrl Pts',(1.65818126992488,1.21416646777651,12.774135089221));
#26740=CARTESIAN_POINT('Ctrl Pts',(1.68354308598506,1.30469303591977,12.9927470969396));
#26741=CARTESIAN_POINT('Ctrl Pts',(1.68722463996854,1.31679653379992,13.0249123682082));
#26742=CARTESIAN_POINT('Ctrl Pts',(1.69213337689861,1.33133708616498,13.0683407618607));
#26743=CARTESIAN_POINT('Ctrl Pts',(1.69867837429913,1.34977620422811,13.1265588187185));
#26744=CARTESIAN_POINT('Ctrl Pts',(1.70972299734984,1.37483700647468,13.2266376630337));
#26745=CARTESIAN_POINT('Ctrl Pts',(1.72444927973632,1.3950115748963,13.3627102778487));
#26746=CARTESIAN_POINT('Ctrl Pts',(1.73426670520185,1.39950513574301,13.4543055384039));
#26747=CARTESIAN_POINT('Ctrl Pts',(1.75881034858134,1.39949125223529,13.6832950819811));
#26748=CARTESIAN_POINT('Ctrl Pts',(1.77844551810905,1.36306231207927,13.86642843719));
#26749=CARTESIAN_POINT('Ctrl Pts',(1.80053468040288,1.28417749446346,14.0568198428129));
#26750=CARTESIAN_POINT('Ctrl Pts',(1.82507813804813,1.19140871647897,14.26626307035));
#26751=CARTESIAN_POINT('Ctrl Pts',(1.8692575005794,0.931514766722571,14.5990322547947));
#26752=CARTESIAN_POINT('Ctrl Pts',(1.93307009276571,0.396108856903805,14.8852542750114));
#26753=CARTESIAN_POINT('Ctrl Pts',(1.99688458337269,-0.212197990694309,
14.9301300790991));
#26754=CARTESIAN_POINT('Ctrl Pts',(2.06560721862504,-0.825356962352493,
14.693797228026));
#26755=CARTESIAN_POINT('Ctrl Pts',(2.13187192198348,-1.25322327405421,14.2216085927445));
#26756=CARTESIAN_POINT('Ctrl Pts',(2.19569364256406,-1.42879756538438,13.6407601664489));
#26757=CARTESIAN_POINT('Ctrl Pts',(2.26439803871978,-1.36567344200437,12.989813124798));
#26758=CARTESIAN_POINT('Ctrl Pts',(2.33070078887648,-1.00708473766736,12.453274391172));
#26759=CARTESIAN_POINT('Ctrl Pts',(2.39454303239137,-0.480177286341525,
12.1560745526581));
#26760=CARTESIAN_POINT('Ctrl Pts',(2.42898246554838,-0.159333681076682,
12.1002778996127));
#26761=CARTESIAN_POINT('Ctrl Pts',(2.44626234486601,0.00213567231429039,
12.1005293499708));
#26762=CARTESIAN_POINT('',(2.62767578687551,5.23816853614149E-11,11.6014703833234));
#26763=CARTESIAN_POINT('Origin',(2.82743338823081,4.5822835629755E-15,11.8));
#26764=CARTESIAN_POINT('Origin',(6.2,0.,14.67));
#26765=CARTESIAN_POINT('',(6.2,-1.4328367550024E-16,12.33));
#26766=CARTESIAN_POINT('Origin',(6.2,0.,13.5));
#26767=CARTESIAN_POINT('Origin',(6.16,0.,13.5));
#26768=CARTESIAN_POINT('',(6.12,-1.53080849893419E-16,12.25));
#26769=CARTESIAN_POINT('Origin',(6.12,0.,13.5));
#26770=CARTESIAN_POINT('',(6.16,-1.4818226269683E-16,12.29));
#26771=CARTESIAN_POINT('Origin',(5.3225,0.,13.5));
#26772=CARTESIAN_POINT('',(4.525,-1.53080849893419E-16,12.25));
#26773=CARTESIAN_POINT('Origin',(4.525,0.,13.5));
#26774=CARTESIAN_POINT('',(5.3225,-1.53080849893419E-16,12.25));
#26775=CARTESIAN_POINT('Origin',(4.525,0.,15.));
#26776=CARTESIAN_POINT('',(4.525,-1.83697019872103E-16,12.));
#26777=CARTESIAN_POINT('Origin',(4.525,0.,13.5));
#26778=CARTESIAN_POINT('Origin',(4.5,0.,13.5));
#26779=CARTESIAN_POINT('',(4.475,-1.8982025386784E-16,11.95));
#26780=CARTESIAN_POINT('Origin',(4.475,0.,13.5));
#26781=CARTESIAN_POINT('',(4.5,-1.86758636869971E-16,11.975));
#26782=CARTESIAN_POINT('Origin',(4.2875,0.,13.5));
#26783=CARTESIAN_POINT('',(4.1,-1.8982025386784E-16,11.95));
#26784=CARTESIAN_POINT('Origin',(4.1,0.,13.5));
#26785=CARTESIAN_POINT('',(4.2875,-1.8982025386784E-16,11.95));
#26786=CARTESIAN_POINT('Origin',(4.1,0.,14.9));
#26787=CARTESIAN_POINT('Origin',(-4.1,0.,15.05));
#26788=CARTESIAN_POINT('',(-4.1,-1.8982025386784E-16,11.95));
#26789=CARTESIAN_POINT('Origin',(-4.1,0.,13.5));
#26790=CARTESIAN_POINT('Origin',(-4.2875,0.,13.5));
#26791=CARTESIAN_POINT('',(-4.475,-1.8982025386784E-16,11.95));
#26792=CARTESIAN_POINT('Origin',(-4.475,0.,13.5));
#26793=CARTESIAN_POINT('',(-4.2875,-1.8982025386784E-16,11.95));
#26794=CARTESIAN_POINT('Origin',(-4.5,0.,13.5));
#26795=CARTESIAN_POINT('',(-4.525,-1.83697019872103E-16,12.));
#26796=CARTESIAN_POINT('',(-4.5,1.86758636869971E-16,11.975));
#26797=CARTESIAN_POINT('Origin',(-4.525,0.,13.5));
#26798=CARTESIAN_POINT('Origin',(-4.525,0.,14.75));
#26799=CARTESIAN_POINT('',(-4.525,-1.53080849893419E-16,12.25));
#26800=CARTESIAN_POINT('Origin',(-4.525,0.,13.5));
#26801=CARTESIAN_POINT('Origin',(-5.8225,0.,13.5));
#26802=CARTESIAN_POINT('',(-7.12,-1.53080849893419E-16,12.25));
#26803=CARTESIAN_POINT('Origin',(-7.12,0.,13.5));
#26804=CARTESIAN_POINT('',(-5.8225,-1.53080849893419E-16,12.25));
#26805=CARTESIAN_POINT('Origin',(-7.16,0.,13.5));
#26806=CARTESIAN_POINT('',(-7.2,-1.4328367550024E-16,12.33));
#26807=CARTESIAN_POINT('',(-7.16,1.4818226269683E-16,12.29));
#26808=CARTESIAN_POINT('Origin',(-7.2,0.,13.5));
#26809=CARTESIAN_POINT('Origin',(-7.2,0.,13.5));
#86394=UNCERTAINTY_MEASURE_WITH_UNIT(LENGTH_MEASURE(0.001),#86430,
'DISTANCE_ACCURACY_VALUE',
'Maximum model space distance between geometric entities at asserted c
onnectivities');
#86409=UNCERTAINTY_MEASURE_WITH_UNIT(LENGTH_MEASURE(0.001),#86430,
'DISTANCE_ACCURACY_VALUE',
'Maximum model space distance between geometric entities at asserted c
onnectivities');
#86414=(
GEOMETRIC_REPRESENTATION_CONTEXT(3)
GLOBAL_UNCERTAINTY_ASSIGNED_CONTEXT((#86394))
GLOBAL_UNIT_ASSIGNED_CONTEXT((#86430,#86432,#86433))
REPRESENTATION_CONTEXT('','3D')
);
#86429=(
GEOMETRIC_REPRESENTATION_CONTEXT(3)
GLOBAL_UNCERTAINTY_ASSIGNED_CONTEXT((#86409))
GLOBAL_UNIT_ASSIGNED_CONTEXT((#86430,#86432,#86433))
REPRESENTATION_CONTEXT('','3D')
);
#86430=(
LENGTH_UNIT()
NAMED_UNIT(*)
SI_UNIT(.CENTI.,.METRE.)
);
#86432=(
NAMED_UNIT(*)
PLANE_ANGLE_UNIT()
SI_UNIT($,.RADIAN.)
);
#86433=(
NAMED_UNIT(*)
SI_UNIT($,.STERADIAN.)
SOLID_ANGLE_UNIT()
);
#86438=SHAPE_DEFINITION_REPRESENTATION(#86457,#86505);
#86457=PRODUCT_DEFINITION_SHAPE('',$,#86525);
#86505=SHAPE_REPRESENTATION('',(#16419),#86414);
#86520=PRODUCT_DEFINITION_CONTEXT('part definition',#86579,'design');
#86525=PRODUCT_DEFINITION('Hardened Steel Worm Shaft m3 z1',
'Hardened Steel Worm Shaft m3 z1',#86544,#86520);
#86544=PRODUCT_DEFINITION_FORMATION('',$,#86585);
#86579=APPLICATION_CONTEXT(
'Core Data for Automotive Mechanical Design Process');
#86580=PRODUCT_CONTEXT('part definition',#86579,'mechanical');
#86585=PRODUCT('Hardened Steel Worm Shaft m3 z1',
'Hardened Steel Worm Shaft m3 z1',$,(#86580));
#86604=PRESENTATION_STYLE_ASSIGNMENT((#86622));
#86622=SURFACE_STYLE_USAGE(.BOTH.,#86640);
#86640=SURFACE_SIDE_STYLE('',(#86658));
#86658=SURFACE_STYLE_FILL_AREA(#86676);
#86676=FILL_AREA_STYLE('Opaque(212,215,220)',(#86694));
#86694=FILL_AREA_STYLE_COLOUR('Opaque(212,215,220)',#86712);
#86712=COLOUR_RGB('Opaque(212,215,220)', 0.40784314, 0.44705882, 0.49803922);
ENDSEC;
END-ISO-10303-21;
